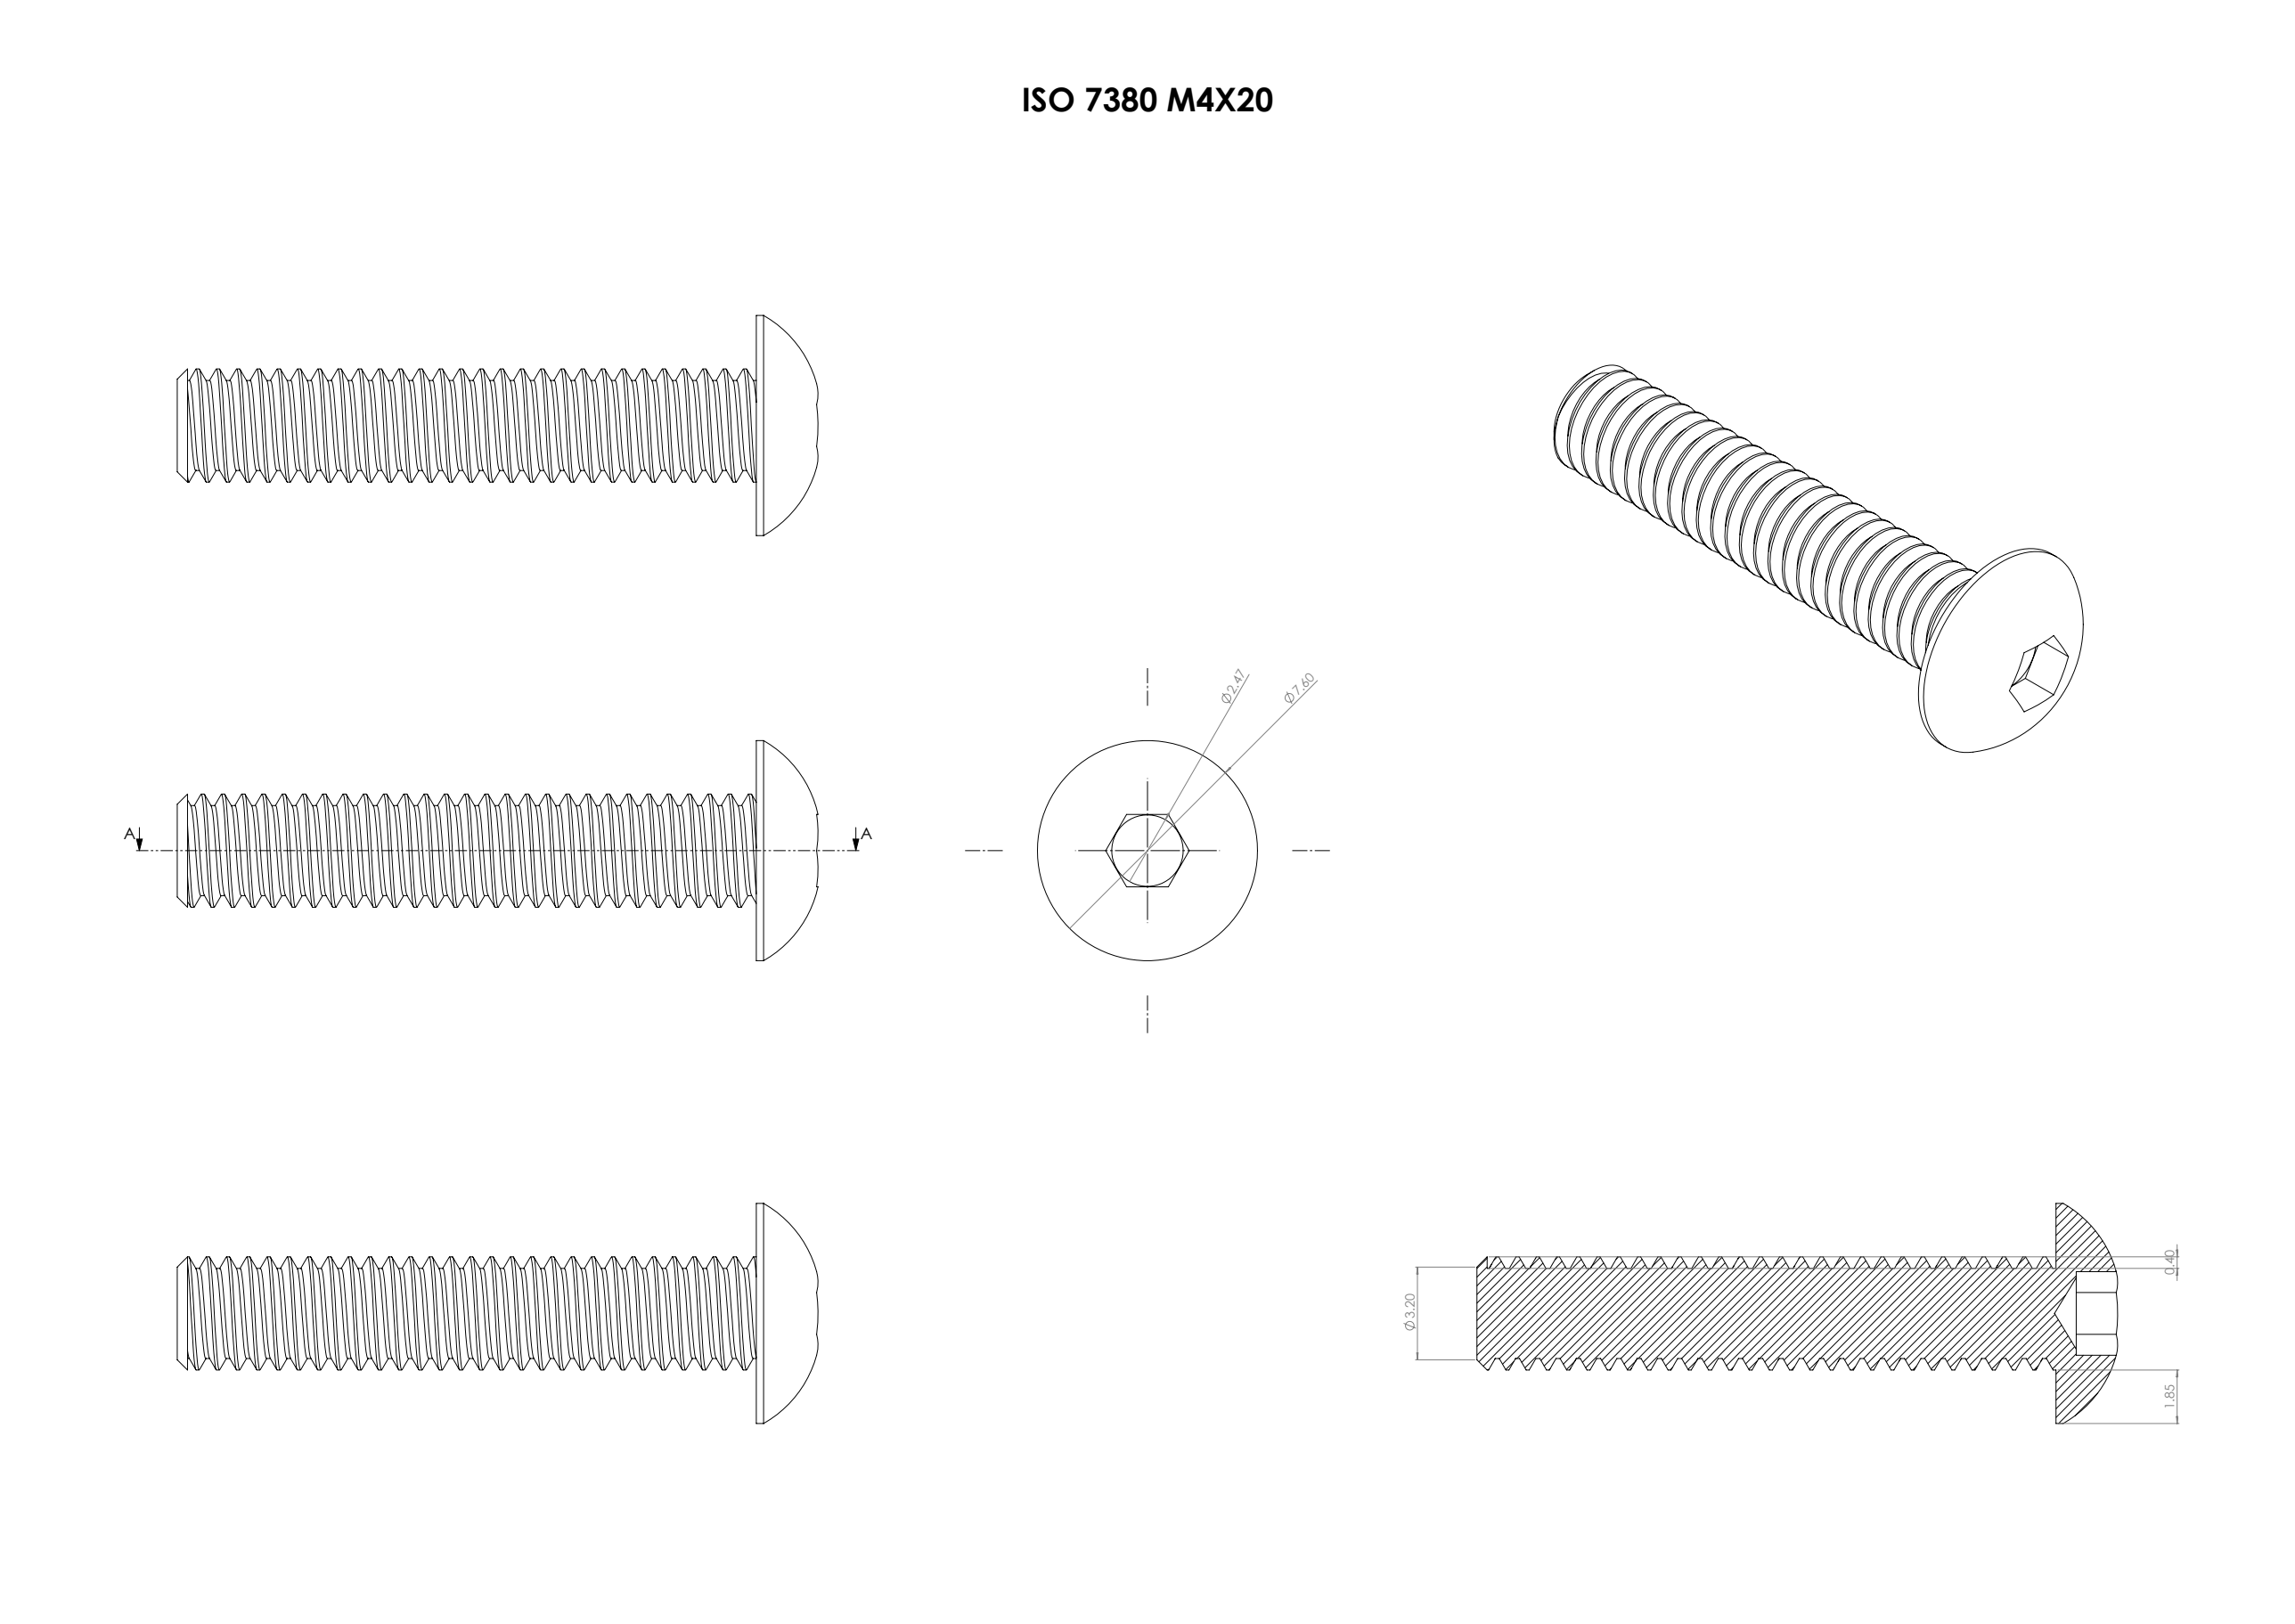
ISO-10303-21;
HEADER;
/* Generated by software containing ST-Developer
 * from STEP Tools, Inc. (www.steptools.com) 
 */

FILE_DESCRIPTION(
/* description */ (''),
/* implementation_level */ '2;1');

FILE_NAME(
/* name */ '11_ISO_7380_M4x20.step',
/* time_stamp */ '2026-10-21T02:01:14-07:00',
/* author */ (''),
/* organization */ (''),
/* preprocessor_version */ 'ST-DEVELOPER v20.2',
/* originating_system */ 'Autodesk Translation Framework v15.15.0.0',
/* authorisation */ '');

FILE_SCHEMA (('AUTOMOTIVE_DESIGN { 1 0 10303 214 3 1 1 }'));
ENDSEC;

DATA;
#10=MECHANICAL_DESIGN_GEOMETRIC_PRESENTATION_REPRESENTATION('',(#623),#37181);
#103=(
BOUNDED_SURFACE()
B_SPLINE_SURFACE(2,2,((#34249,#34250,#34251,#34252,#34253,#34254,#34255,
#34256,#34257),(#34258,#34259,#34260,#34261,#34262,#34263,#34264,#34265,
#34266),(#34267,#34268,#34269,#34270,#34271,#34272,#34273,#34274,#34275)),
 .UNSPECIFIED.,.F.,.T.,.F.)
B_SPLINE_SURFACE_WITH_KNOTS((3,3),(3,2,2,2,3),(0.516279708895519,1.35421937474488),
(-3.14159265358979,-1.5707963267949,0.,1.5707963267949,3.14159265358979),
 .UNSPECIFIED.)
GEOMETRIC_REPRESENTATION_ITEM()
RATIONAL_B_SPLINE_SURFACE(((1.,0.707106781186548,1.,0.707106781186548,1.,
0.707106781186548,1.,0.707106781186548,1.),(0.91350851712624,0.645948067131631,
0.91350851712624,0.645948067131631,0.91350851712624,0.645948067131631,0.91350851712624,
0.645948067131631,0.91350851712624),(1.,0.707106781186548,1.,0.707106781186548,
1.,0.707106781186548,1.,0.707106781186548,1.)))
REPRESENTATION_ITEM('')
SURFACE()
);
#116=B_SPLINE_SURFACE_WITH_KNOTS('',3,3,((#32297,#32298,#32299,#32300,#32301,
#32302,#32303,#32304,#32305,#32306,#32307,#32308,#32309,#32310,#32311,#32312,
#32313,#32314,#32315,#32316,#32317,#32318,#32319,#32320,#32321,#32322,#32323,
#32324,#32325,#32326,#32327,#32328,#32329,#32330,#32331,#32332,#32333,#32334,
#32335,#32336,#32337,#32338,#32339,#32340,#32341,#32342,#32343,#32344,#32345,
#32346,#32347,#32348,#32349,#32350,#32351,#32352,#32353,#32354,#32355,#32356,
#32357,#32358,#32359,#32360,#32361,#32362,#32363,#32364,#32365,#32366,#32367,
#32368,#32369,#32370,#32371,#32372,#32373,#32374,#32375,#32376,#32377,#32378,
#32379,#32380,#32381,#32382,#32383,#32384,#32385,#32386,#32387,#32388,#32389,
#32390,#32391,#32392,#32393,#32394,#32395,#32396,#32397,#32398,#32399,#32400,
#32401,#32402,#32403,#32404,#32405,#32406,#32407,#32408,#32409,#32410,#32411,
#32412,#32413,#32414,#32415,#32416,#32417,#32418,#32419,#32420,#32421,#32422,
#32423,#32424,#32425,#32426,#32427,#32428,#32429,#32430,#32431,#32432,#32433,
#32434,#32435,#32436,#32437,#32438,#32439,#32440,#32441,#32442,#32443,#32444,
#32445,#32446,#32447,#32448,#32449,#32450,#32451,#32452,#32453,#32454,#32455,
#32456,#32457,#32458,#32459,#32460,#32461,#32462,#32463,#32464,#32465,#32466,
#32467,#32468,#32469,#32470,#32471,#32472,#32473,#32474,#32475,#32476,#32477,
#32478),(#32479,#32480,#32481,#32482,#32483,#32484,#32485,#32486,#32487,
#32488,#32489,#32490,#32491,#32492,#32493,#32494,#32495,#32496,#32497,#32498,
#32499,#32500,#32501,#32502,#32503,#32504,#32505,#32506,#32507,#32508,#32509,
#32510,#32511,#32512,#32513,#32514,#32515,#32516,#32517,#32518,#32519,#32520,
#32521,#32522,#32523,#32524,#32525,#32526,#32527,#32528,#32529,#32530,#32531,
#32532,#32533,#32534,#32535,#32536,#32537,#32538,#32539,#32540,#32541,#32542,
#32543,#32544,#32545,#32546,#32547,#32548,#32549,#32550,#32551,#32552,#32553,
#32554,#32555,#32556,#32557,#32558,#32559,#32560,#32561,#32562,#32563,#32564,
#32565,#32566,#32567,#32568,#32569,#32570,#32571,#32572,#32573,#32574,#32575,
#32576,#32577,#32578,#32579,#32580,#32581,#32582,#32583,#32584,#32585,#32586,
#32587,#32588,#32589,#32590,#32591,#32592,#32593,#32594,#32595,#32596,#32597,
#32598,#32599,#32600,#32601,#32602,#32603,#32604,#32605,#32606,#32607,#32608,
#32609,#32610,#32611,#32612,#32613,#32614,#32615,#32616,#32617,#32618,#32619,
#32620,#32621,#32622,#32623,#32624,#32625,#32626,#32627,#32628,#32629,#32630,
#32631,#32632,#32633,#32634,#32635,#32636,#32637,#32638,#32639,#32640,#32641,
#32642,#32643,#32644,#32645,#32646,#32647,#32648,#32649,#32650,#32651,#32652,
#32653,#32654,#32655,#32656,#32657,#32658,#32659,#32660),(#32661,#32662,
#32663,#32664,#32665,#32666,#32667,#32668,#32669,#32670,#32671,#32672,#32673,
#32674,#32675,#32676,#32677,#32678,#32679,#32680,#32681,#32682,#32683,#32684,
#32685,#32686,#32687,#32688,#32689,#32690,#32691,#32692,#32693,#32694,#32695,
#32696,#32697,#32698,#32699,#32700,#32701,#32702,#32703,#32704,#32705,#32706,
#32707,#32708,#32709,#32710,#32711,#32712,#32713,#32714,#32715,#32716,#32717,
#32718,#32719,#32720,#32721,#32722,#32723,#32724,#32725,#32726,#32727,#32728,
#32729,#32730,#32731,#32732,#32733,#32734,#32735,#32736,#32737,#32738,#32739,
#32740,#32741,#32742,#32743,#32744,#32745,#32746,#32747,#32748,#32749,#32750,
#32751,#32752,#32753,#32754,#32755,#32756,#32757,#32758,#32759,#32760,#32761,
#32762,#32763,#32764,#32765,#32766,#32767,#32768,#32769,#32770,#32771,#32772,
#32773,#32774,#32775,#32776,#32777,#32778,#32779,#32780,#32781,#32782,#32783,
#32784,#32785,#32786,#32787,#32788,#32789,#32790,#32791,#32792,#32793,#32794,
#32795,#32796,#32797,#32798,#32799,#32800,#32801,#32802,#32803,#32804,#32805,
#32806,#32807,#32808,#32809,#32810,#32811,#32812,#32813,#32814,#32815,#32816,
#32817,#32818,#32819,#32820,#32821,#32822,#32823,#32824,#32825,#32826,#32827,
#32828,#32829,#32830,#32831,#32832,#32833,#32834,#32835,#32836,#32837,#32838,
#32839,#32840,#32841,#32842),(#32843,#32844,#32845,#32846,#32847,#32848,
#32849,#32850,#32851,#32852,#32853,#32854,#32855,#32856,#32857,#32858,#32859,
#32860,#32861,#32862,#32863,#32864,#32865,#32866,#32867,#32868,#32869,#32870,
#32871,#32872,#32873,#32874,#32875,#32876,#32877,#32878,#32879,#32880,#32881,
#32882,#32883,#32884,#32885,#32886,#32887,#32888,#32889,#32890,#32891,#32892,
#32893,#32894,#32895,#32896,#32897,#32898,#32899,#32900,#32901,#32902,#32903,
#32904,#32905,#32906,#32907,#32908,#32909,#32910,#32911,#32912,#32913,#32914,
#32915,#32916,#32917,#32918,#32919,#32920,#32921,#32922,#32923,#32924,#32925,
#32926,#32927,#32928,#32929,#32930,#32931,#32932,#32933,#32934,#32935,#32936,
#32937,#32938,#32939,#32940,#32941,#32942,#32943,#32944,#32945,#32946,#32947,
#32948,#32949,#32950,#32951,#32952,#32953,#32954,#32955,#32956,#32957,#32958,
#32959,#32960,#32961,#32962,#32963,#32964,#32965,#32966,#32967,#32968,#32969,
#32970,#32971,#32972,#32973,#32974,#32975,#32976,#32977,#32978,#32979,#32980,
#32981,#32982,#32983,#32984,#32985,#32986,#32987,#32988,#32989,#32990,#32991,
#32992,#32993,#32994,#32995,#32996,#32997,#32998,#32999,#33000,#33001,#33002,
#33003,#33004,#33005,#33006,#33007,#33008,#33009,#33010,#33011,#33012,#33013,
#33014,#33015,#33016,#33017,#33018,#33019,#33020,#33021,#33022,#33023,#33024)),
 .UNSPECIFIED.,.F.,.F.,.F.,(4,4),(4,1,1,1,1,1,1,1,1,1,1,1,1,1,1,1,1,1,1,
1,1,1,1,1,1,1,1,1,1,1,1,1,1,1,1,1,1,1,1,1,1,1,1,1,1,1,1,1,1,1,1,1,1,1,1,
1,1,1,1,1,1,1,1,1,1,1,1,1,1,1,1,1,1,1,1,1,1,1,1,1,1,1,1,1,1,1,1,1,1,1,1,
1,1,1,1,1,1,1,1,1,1,1,1,1,1,1,1,1,1,1,1,1,1,1,1,1,1,1,1,1,1,1,1,1,1,1,1,
1,1,1,1,1,1,1,1,1,1,1,1,1,1,1,1,1,1,1,1,1,1,1,1,1,1,1,1,1,1,1,1,1,1,1,1,
1,1,1,1,1,1,1,1,1,1,1,1,1,1,1,1,4),(0.,0.0460148164544131),(8.3105869227399,
9.3072753236828,10.3039637246257,11.3006521255686,12.2973405265115,13.2940289274544,
14.2907173283973,15.2874057293402,16.2840941302831,17.280782531226,18.2774709321689,
19.2741593331118,20.2708477340547,21.2675361349975,22.2642245359404,23.2609129368833,
24.2576013378262,25.2542897387691,26.250978139712,27.2476665406549,28.2443549415978,
29.2410433425407,30.2377317434836,31.2344201444265,32.2311085453694,33.2277969463123,
34.2244853472552,35.2211737481981,36.217862149141,37.2145505500839,38.2112389510268,
39.2079273519697,40.2046157529126,41.2013041538555,42.1979925547984,43.1946809557413,
44.1913693566841,45.188057757627,46.18474615857,47.1814345595128,48.1781229604557,
49.1748113613986,50.1714997623415,51.1681881632844,52.1648765642273,53.1615649651702,
54.1582533661131,55.154941767056,56.1516301679989,57.1483185689418,58.1450069698847,
59.1416953708276,60.1383837717705,61.1350721727134,62.1317605736563,63.1284489745992,
64.1251373755421,65.121825776485,66.1185141774279,67.1152025783708,68.1118909793137,
69.1085793802565,70.1052677811994,71.1019561821423,72.0986445830852,73.0953329840281,
74.092021384971,75.0887097859139,76.0853981868568,77.0820865877997,78.0787749887426,
79.0754633896855,80.0721517906284,81.0688401915713,82.0655285925142,83.0622169934571,
84.0589053944,85.0555937953429,86.0522821962858,87.0489705972287,88.0456589981716,
89.0423473991145,90.0390358000574,91.0357242010002,92.0324126019432,93.029101002886,
94.0257894038289,95.0224778047718,96.0191662057147,97.0158546066576,98.0125430076005,
99.0092314085434,100.005919809486,101.002608210429,101.999296611372,102.995985012315,
103.992673413258,104.989361814201,105.986050215144,106.982738616087,107.979427017029,
108.976115417972,109.972803818915,110.969492219858,111.966180620801,112.962869021744,
113.959557422687,114.95624582363,115.952934224573,116.949622625516,117.946311026458,
118.942999427401,119.939687828344,120.936376229287,121.93306463023,122.929753031173,
123.926441432116,124.923129833059,125.919818234002,126.916506634944,127.913195035887,
128.90988343683,129.906571837773,130.903260238716,131.899948639659,132.896637040602,
133.893325441545,134.890013842488,135.886702243431,136.883390644373,137.880079045316,
138.876767446259,139.873455847202,140.870144248145,141.866832649088,142.863521050031,
143.860209450974,144.856897851917,145.85358625286,146.850274653802,147.846963054745,
148.843651455688,149.840339856631,150.837028257574,151.833716658517,152.83040505946,
153.827093460403,154.823781861346,155.820470262288,156.817158663231,157.813847064174,
158.810535465117,159.80722386606,160.803912267003,161.800600667946,162.797289068889,
163.793977469832,164.790665870775,165.787354271717,166.78404267266,167.780731073603,
168.777419474546,169.774107875489,170.770796276432,171.767484677375,172.764173078318,
173.760861479261,174.757549880203,175.754238281146,176.750926682089,177.747615083032,
178.744303483975,179.740991884918,180.737680285861,181.734368686804,182.731057087747,
183.72774548869,184.724433889632,185.721122290575,186.717810691518),
 .UNSPECIFIED.);
#117=B_SPLINE_SURFACE_WITH_KNOTS('',3,3,((#33328,#33329,#33330,#33331,#33332,
#33333,#33334,#33335,#33336,#33337,#33338,#33339,#33340,#33341,#33342,#33343,
#33344,#33345,#33346,#33347,#33348,#33349,#33350,#33351,#33352,#33353,#33354,
#33355,#33356,#33357,#33358,#33359,#33360,#33361,#33362,#33363,#33364,#33365,
#33366,#33367,#33368,#33369,#33370,#33371,#33372,#33373,#33374,#33375,#33376,
#33377,#33378,#33379,#33380,#33381,#33382,#33383,#33384,#33385,#33386,#33387,
#33388,#33389,#33390,#33391,#33392,#33393,#33394,#33395,#33396,#33397,#33398,
#33399,#33400,#33401,#33402,#33403,#33404,#33405,#33406,#33407,#33408,#33409,
#33410,#33411,#33412,#33413,#33414,#33415,#33416,#33417,#33418,#33419,#33420,
#33421,#33422,#33423,#33424,#33425,#33426,#33427,#33428,#33429,#33430,#33431,
#33432,#33433,#33434,#33435,#33436,#33437,#33438,#33439,#33440,#33441,#33442,
#33443,#33444,#33445,#33446,#33447,#33448,#33449,#33450,#33451,#33452,#33453,
#33454,#33455,#33456,#33457,#33458,#33459,#33460,#33461,#33462,#33463,#33464,
#33465,#33466,#33467,#33468,#33469,#33470,#33471,#33472,#33473,#33474,#33475,
#33476,#33477,#33478,#33479,#33480,#33481,#33482,#33483,#33484,#33485,#33486,
#33487,#33488,#33489,#33490,#33491,#33492,#33493,#33494,#33495,#33496,#33497,
#33498,#33499,#33500,#33501,#33502,#33503,#33504,#33505,#33506,#33507,#33508,
#33509),(#33510,#33511,#33512,#33513,#33514,#33515,#33516,#33517,#33518,
#33519,#33520,#33521,#33522,#33523,#33524,#33525,#33526,#33527,#33528,#33529,
#33530,#33531,#33532,#33533,#33534,#33535,#33536,#33537,#33538,#33539,#33540,
#33541,#33542,#33543,#33544,#33545,#33546,#33547,#33548,#33549,#33550,#33551,
#33552,#33553,#33554,#33555,#33556,#33557,#33558,#33559,#33560,#33561,#33562,
#33563,#33564,#33565,#33566,#33567,#33568,#33569,#33570,#33571,#33572,#33573,
#33574,#33575,#33576,#33577,#33578,#33579,#33580,#33581,#33582,#33583,#33584,
#33585,#33586,#33587,#33588,#33589,#33590,#33591,#33592,#33593,#33594,#33595,
#33596,#33597,#33598,#33599,#33600,#33601,#33602,#33603,#33604,#33605,#33606,
#33607,#33608,#33609,#33610,#33611,#33612,#33613,#33614,#33615,#33616,#33617,
#33618,#33619,#33620,#33621,#33622,#33623,#33624,#33625,#33626,#33627,#33628,
#33629,#33630,#33631,#33632,#33633,#33634,#33635,#33636,#33637,#33638,#33639,
#33640,#33641,#33642,#33643,#33644,#33645,#33646,#33647,#33648,#33649,#33650,
#33651,#33652,#33653,#33654,#33655,#33656,#33657,#33658,#33659,#33660,#33661,
#33662,#33663,#33664,#33665,#33666,#33667,#33668,#33669,#33670,#33671,#33672,
#33673,#33674,#33675,#33676,#33677,#33678,#33679,#33680,#33681,#33682,#33683,
#33684,#33685,#33686,#33687,#33688,#33689,#33690,#33691),(#33692,#33693,
#33694,#33695,#33696,#33697,#33698,#33699,#33700,#33701,#33702,#33703,#33704,
#33705,#33706,#33707,#33708,#33709,#33710,#33711,#33712,#33713,#33714,#33715,
#33716,#33717,#33718,#33719,#33720,#33721,#33722,#33723,#33724,#33725,#33726,
#33727,#33728,#33729,#33730,#33731,#33732,#33733,#33734,#33735,#33736,#33737,
#33738,#33739,#33740,#33741,#33742,#33743,#33744,#33745,#33746,#33747,#33748,
#33749,#33750,#33751,#33752,#33753,#33754,#33755,#33756,#33757,#33758,#33759,
#33760,#33761,#33762,#33763,#33764,#33765,#33766,#33767,#33768,#33769,#33770,
#33771,#33772,#33773,#33774,#33775,#33776,#33777,#33778,#33779,#33780,#33781,
#33782,#33783,#33784,#33785,#33786,#33787,#33788,#33789,#33790,#33791,#33792,
#33793,#33794,#33795,#33796,#33797,#33798,#33799,#33800,#33801,#33802,#33803,
#33804,#33805,#33806,#33807,#33808,#33809,#33810,#33811,#33812,#33813,#33814,
#33815,#33816,#33817,#33818,#33819,#33820,#33821,#33822,#33823,#33824,#33825,
#33826,#33827,#33828,#33829,#33830,#33831,#33832,#33833,#33834,#33835,#33836,
#33837,#33838,#33839,#33840,#33841,#33842,#33843,#33844,#33845,#33846,#33847,
#33848,#33849,#33850,#33851,#33852,#33853,#33854,#33855,#33856,#33857,#33858,
#33859,#33860,#33861,#33862,#33863,#33864,#33865,#33866,#33867,#33868,#33869,
#33870,#33871,#33872,#33873),(#33874,#33875,#33876,#33877,#33878,#33879,
#33880,#33881,#33882,#33883,#33884,#33885,#33886,#33887,#33888,#33889,#33890,
#33891,#33892,#33893,#33894,#33895,#33896,#33897,#33898,#33899,#33900,#33901,
#33902,#33903,#33904,#33905,#33906,#33907,#33908,#33909,#33910,#33911,#33912,
#33913,#33914,#33915,#33916,#33917,#33918,#33919,#33920,#33921,#33922,#33923,
#33924,#33925,#33926,#33927,#33928,#33929,#33930,#33931,#33932,#33933,#33934,
#33935,#33936,#33937,#33938,#33939,#33940,#33941,#33942,#33943,#33944,#33945,
#33946,#33947,#33948,#33949,#33950,#33951,#33952,#33953,#33954,#33955,#33956,
#33957,#33958,#33959,#33960,#33961,#33962,#33963,#33964,#33965,#33966,#33967,
#33968,#33969,#33970,#33971,#33972,#33973,#33974,#33975,#33976,#33977,#33978,
#33979,#33980,#33981,#33982,#33983,#33984,#33985,#33986,#33987,#33988,#33989,
#33990,#33991,#33992,#33993,#33994,#33995,#33996,#33997,#33998,#33999,#34000,
#34001,#34002,#34003,#34004,#34005,#34006,#34007,#34008,#34009,#34010,#34011,
#34012,#34013,#34014,#34015,#34016,#34017,#34018,#34019,#34020,#34021,#34022,
#34023,#34024,#34025,#34026,#34027,#34028,#34029,#34030,#34031,#34032,#34033,
#34034,#34035,#34036,#34037,#34038,#34039,#34040,#34041,#34042,#34043,#34044,
#34045,#34046,#34047,#34048,#34049,#34050,#34051,#34052,#34053,#34054,#34055)),
 .UNSPECIFIED.,.F.,.F.,.F.,(4,4),(4,1,1,1,1,1,1,1,1,1,1,1,1,1,1,1,1,1,1,
1,1,1,1,1,1,1,1,1,1,1,1,1,1,1,1,1,1,1,1,1,1,1,1,1,1,1,1,1,1,1,1,1,1,1,1,
1,1,1,1,1,1,1,1,1,1,1,1,1,1,1,1,1,1,1,1,1,1,1,1,1,1,1,1,1,1,1,1,1,1,1,1,
1,1,1,1,1,1,1,1,1,1,1,1,1,1,1,1,1,1,1,1,1,1,1,1,1,1,1,1,1,1,1,1,1,1,1,1,
1,1,1,1,1,1,1,1,1,1,1,1,1,1,1,1,1,1,1,1,1,1,1,1,1,1,1,1,1,1,1,1,1,1,1,1,
1,1,1,1,1,1,1,1,1,1,1,1,1,1,1,1,4),(0.,0.0460148164544131),(11.6154215191108,
12.6121099200537,13.6087983209966,14.6054867219395,15.6021751228824,16.5988635238253,
17.5955519247682,18.592240325711,19.5889287266539,20.5856171275968,21.5823055285397,
22.5789939294826,23.5756823304255,24.5723707313684,25.5690591323113,26.5657475332542,
27.5624359341971,28.55912433514,29.5558127360829,30.5525011370258,31.5491895379687,
32.5458779389116,33.5425663398545,34.5392547407974,35.5359431417403,36.5326315426832,
37.5293199436261,38.526008344569,39.5226967455119,40.5193851464548,41.5160735473976,
42.5127619483405,43.5094503492834,44.5061387502263,45.5028271511692,46.4995155521121,
47.496203953055,48.4928923539979,49.4895807549408,50.4862691558837,51.4829575568266,
52.4796459577695,53.4763343587124,54.4730227596553,55.4697111605982,56.4663995615411,
57.463087962484,58.4597763634269,59.4564647643698,60.4531531653127,61.4498415662556,
62.4465299671985,63.4432183681413,64.4399067690842,65.4365951700271,66.43328357097,
67.4299719719129,68.4266603728558,69.4233487737987,70.4200371747416,71.4167255756845,
72.4134139766274,73.4101023775703,74.4067907785132,75.4034791794561,76.400167580399,
77.3968559813419,78.3935443822848,79.3902327832277,80.3869211841706,81.3836095851135,
82.3802979860564,83.3769863869992,84.3736747879422,85.3703631888851,86.3670515898279,
87.3637399907708,88.3604283917137,89.3571167926566,90.3538051935995,91.3504935945424,
92.3471819954853,93.3438703964282,94.3405587973711,95.337247198314,96.3339355992569,
97.3306240001998,98.3273124011427,99.3240008020856,100.320689203028,101.317377603971,
102.314066004914,103.310754405857,104.3074428068,105.304131207743,106.300819608686,
107.297508009629,108.294196410572,109.290884811515,110.287573212457,111.2842616134,
112.280950014343,113.277638415286,114.274326816229,115.271015217172,116.267703618115,
117.264392019058,118.261080420001,119.257768820943,120.254457221886,121.251145622829,
122.247834023772,123.244522424715,124.241210825658,125.237899226601,126.234587627544,
127.231276028487,128.22796442943,129.224652830372,130.221341231315,131.218029632258,
132.214718033201,133.211406434144,134.208094835087,135.20478323603,136.201471636973,
137.198160037916,138.194848438859,139.191536839801,140.188225240744,141.184913641687,
142.18160204263,143.178290443573,144.174978844516,145.171667245459,146.168355646402,
147.165044047345,148.161732448287,149.15842084923,150.155109250173,151.151797651116,
152.148486052059,153.145174453002,154.141862853945,155.138551254888,156.135239655831,
157.131928056774,158.128616457716,159.125304858659,160.121993259602,161.118681660545,
162.115370061488,163.112058462431,164.108746863374,165.105435264317,166.10212366526,
167.098812066202,168.095500467145,169.092188868088,170.088877269031,171.085565669974,
172.082254070917,173.07894247186,174.075630872803,175.072319273746,176.069007674689,
177.065696075631,178.062384476574,179.059072877517,180.05576127846,181.052449679403,
182.049138080346,183.045826481289,184.042514882232,185.039203283175,186.035891684118,
187.03258008506,188.029268486003,189.025956886946,190.022645287889),
 .UNSPECIFIED.);
#379=B_SPLINE_CURVE_WITH_KNOTS('',3,(#30252,#30253,#30254,#30255,#30256,
#30257,#30258,#30259,#30260,#30261),.UNSPECIFIED.,.F.,.F.,(4,3,3,4),(-4.09254174883827,
-3.98675360377158,-2.99006520282869,-2.06514013327809),.UNSPECIFIED.);
#380=B_SPLINE_CURVE_WITH_KNOTS('',3,(#30264,#30265,#30266,#30267,#30268,
#30269,#30270),.UNSPECIFIED.,.F.,.F.,(4,3,4),(0.,0.996688400942905,1.11419103802963),
 .UNSPECIFIED.);
#381=B_SPLINE_CURVE_WITH_KNOTS('',3,(#30275,#30276,#30277,#30278,#30279,
#30280,#30281,#30282,#30283,#30284,#30285,#30286,#30287,#30288,#30289,#30290,
#30291,#30292,#30293,#30294,#30295,#30296),.UNSPECIFIED.,.F.,.F.,(4,3,3,
3,3,3,3,4),(-10.3757270560179,-9.96688400942895,-8.97019560848606,-7.97350720754317,
-6.97681880660027,-5.98013040565738,-4.98344200471448,-4.09254174883827),
 .UNSPECIFIED.);
#382=B_SPLINE_CURVE_WITH_KNOTS('',3,(#30297,#30298,#30299,#30300,#30301,
#30302,#30303,#30304,#30305,#30306,#30307,#30308,#30309,#30310,#30311,#30312,
#30313,#30314,#30315,#30316,#30317,#30318),.UNSPECIFIED.,.F.,.F.,(4,3,3,
3,3,3,3,4),(1.11419103802963,1.9933768018858,2.99006520282869,3.98675360377159,
4.98344200471448,5.98013040565737,6.97681880660027,7.39737634520922),
 .UNSPECIFIED.);
#383=B_SPLINE_CURVE_WITH_KNOTS('',3,(#30323,#30324,#30325,#30326,#30327,
#30328,#30329,#30330,#30331,#30332,#30333,#30334,#30335,#30336,#30337,#30338,
#30339,#30340,#30341,#30342,#30343,#30344),.UNSPECIFIED.,.F.,.F.,(4,3,3,
3,3,3,3,4),(-16.6589123631975,-15.9470144150863,-14.9503260141434,-13.9536376132005,
-12.9569492122576,-11.9602608113147,-10.9635724103719,-10.3757270560179),
 .UNSPECIFIED.);
#384=B_SPLINE_CURVE_WITH_KNOTS('',3,(#30345,#30346,#30347,#30348,#30349,
#30350,#30351,#30352,#30353,#30354,#30355,#30356,#30357,#30358,#30359,#30360,
#30361,#30362,#30363,#30364,#30365,#30366),.UNSPECIFIED.,.F.,.F.,(4,3,3,
3,3,3,3,4),(7.39737634520922,7.97350720754316,8.97019560848606,9.96688400942896,
10.9635724103719,11.9602608113148,12.9569492122576,13.6805616523888),
 .UNSPECIFIED.);
#385=B_SPLINE_CURVE_WITH_KNOTS('',3,(#30371,#30372,#30373,#30374,#30375,
#30376,#30377,#30378,#30379,#30380,#30381,#30382,#30383,#30384,#30385,#30386,
#30387,#30388,#30389,#30390,#30391,#30392,#30393,#30394,#30395),
 .UNSPECIFIED.,.F.,.F.,(4,3,3,3,3,3,3,3,4),(-22.942097670377,-22.9238332216866,
-21.9271448207437,-20.9304564198008,-19.9337680188579,-18.937079617915,
-17.9403912169721,-16.9437028160292,-16.6589123631975),.UNSPECIFIED.);
#386=B_SPLINE_CURVE_WITH_KNOTS('',3,(#30396,#30397,#30398,#30399,#30400,
#30401,#30402,#30403,#30404,#30405,#30406,#30407,#30408,#30409,#30410,#30411,
#30412,#30413,#30414,#30415,#30416,#30417,#30418,#30419,#30420),
 .UNSPECIFIED.,.F.,.F.,(4,3,3,3,3,3,3,3,4),(13.6805616523888,13.9536376132005,
14.9503260141434,15.9470144150863,16.9437028160292,17.9403912169721,18.937079617915,
19.9337680188579,19.9637469595684),.UNSPECIFIED.);
#387=B_SPLINE_CURVE_WITH_KNOTS('',3,(#30425,#30426,#30427,#30428,#30429,
#30430,#30431,#30432,#30433,#30434,#30435,#30436,#30437,#30438,#30439,#30440,
#30441,#30442,#30443,#30444,#30445,#30446),.UNSPECIFIED.,.F.,.F.,(4,3,3,
3,3,3,3,4),(-29.2252829775566,-28.903963627344,-27.9072752264011,-26.9105868254582,
-25.9138984245153,-24.9172100235724,-23.9205216226295,-22.942097670377),
 .UNSPECIFIED.);
#388=B_SPLINE_CURVE_WITH_KNOTS('',3,(#30447,#30448,#30449,#30450,#30451,
#30452,#30453,#30454,#30455,#30456,#30457,#30458,#30459,#30460,#30461,#30462,
#30463,#30464,#30465,#30466,#30467,#30468),.UNSPECIFIED.,.F.,.F.,(4,3,3,
3,3,3,3,4),(19.9637469595684,20.9304564198008,21.9271448207437,22.9238332216866,
23.9205216226295,24.9172100235724,25.9138984245153,26.246932266748),
 .UNSPECIFIED.);
#389=B_SPLINE_CURVE_WITH_KNOTS('',3,(#30473,#30474,#30475,#30476,#30477,
#30478,#30479,#30480,#30481,#30482,#30483,#30484,#30485,#30486,#30487,#30488,
#30489,#30490,#30491,#30492,#30493,#30494),.UNSPECIFIED.,.F.,.F.,(4,3,3,
3,3,3,3,4),(-35.5084682847362,-34.8840940330013,-33.8874056320584,-32.8907172311156,
-31.8940288301727,-30.8973404292298,-29.9006520282869,-29.2252829775566),
 .UNSPECIFIED.);
#390=B_SPLINE_CURVE_WITH_KNOTS('',3,(#30495,#30496,#30497,#30498,#30499,
#30500,#30501,#30502,#30503,#30504,#30505,#30506,#30507,#30508,#30509,#30510,
#30511,#30512,#30513,#30514,#30515,#30516),.UNSPECIFIED.,.F.,.F.,(4,3,3,
3,3,3,3,4),(26.246932266748,26.9105868254582,27.9072752264011,28.903963627344,
29.9006520282869,30.8973404292298,31.8940288301727,32.5301175739276),
 .UNSPECIFIED.);
#391=B_SPLINE_CURVE_WITH_KNOTS('',3,(#30521,#30522,#30523,#30524,#30525,
#30526,#30527,#30528,#30529,#30530,#30531,#30532,#30533,#30534,#30535,#30536,
#30537,#30538,#30539,#30540,#30541,#30542),.UNSPECIFIED.,.F.,.F.,(4,3,3,
3,3,3,3,4),(-41.7916535919158,-40.8642244386587,-39.8675360377158,-38.8708476367729,
-37.87415923583,-36.8774708348871,-35.8807824339442,-35.5084682847362),
 .UNSPECIFIED.);
#392=B_SPLINE_CURVE_WITH_KNOTS('',3,(#30543,#30544,#30545,#30546,#30547,
#30548,#30549,#30550,#30551,#30552,#30553,#30554,#30555,#30556,#30557,#30558,
#30559,#30560,#30561,#30562,#30563,#30564),.UNSPECIFIED.,.F.,.F.,(4,3,3,
3,3,3,3,4),(32.5301175739276,32.8907172311156,33.8874056320585,34.8840940330014,
35.8807824339443,36.8774708348872,37.8741592358301,38.8133028811072),
 .UNSPECIFIED.);
#393=B_SPLINE_CURVE_WITH_KNOTS('',3,(#30569,#30570,#30571,#30572,#30573,
#30574,#30575,#30576,#30577,#30578,#30579,#30580,#30581,#30582,#30583,#30584,
#30585,#30586,#30587,#30588,#30589,#30590,#30591,#30592,#30593),
 .UNSPECIFIED.,.F.,.F.,(4,3,3,3,3,3,3,3,4),(-48.0748388990954,-47.841043245259,
-46.8443548443161,-45.8476664433732,-44.8509780424303,-43.8542896414874,
-42.8576012405445,-41.8609128396016,-41.7916535919158),.UNSPECIFIED.);
#394=B_SPLINE_CURVE_WITH_KNOTS('',3,(#30594,#30595,#30596,#30597,#30598,
#30599,#30600,#30601,#30602,#30603,#30604,#30605,#30606,#30607,#30608,#30609,
#30610,#30611,#30612,#30613,#30614,#30615,#30616,#30617,#30618),
 .UNSPECIFIED.,.F.,.F.,(4,3,3,3,3,3,3,3,4),(38.8133028811072,38.8708476367729,
39.8675360377158,40.8642244386587,41.8609128396016,42.8576012405445,43.8542896414874,
44.8509780424303,45.0964881882868),.UNSPECIFIED.);
#395=B_SPLINE_CURVE_WITH_KNOTS('',3,(#30623,#30624,#30625,#30626,#30627,
#30628,#30629,#30630,#30631,#30632,#30633,#30634,#30635,#30636,#30637,#30638,
#30639,#30640,#30641,#30642,#30643,#30644),.UNSPECIFIED.,.F.,.F.,(4,3,3,
3,3,3,3,4),(-54.358024206275,-53.8211736509164,-52.8244852499735,-51.8277968490306,
-50.8311084480877,-49.8344200471448,-48.8377316462019,-48.0748388990954),
 .UNSPECIFIED.);
#396=B_SPLINE_CURVE_WITH_KNOTS('',3,(#30645,#30646,#30647,#30648,#30649,
#30650,#30651,#30652,#30653,#30654,#30655,#30656,#30657,#30658,#30659,#30660,
#30661,#30662,#30663,#30664,#30665,#30666),.UNSPECIFIED.,.F.,.F.,(4,3,3,
3,3,3,3,4),(45.0964881882868,45.8476664433732,46.8443548443161,47.841043245259,
48.8377316462019,49.8344200471448,50.8311084480877,51.3796734954663),
 .UNSPECIFIED.);
#397=B_SPLINE_CURVE_WITH_KNOTS('',3,(#30671,#30672,#30673,#30674,#30675,
#30676,#30677,#30678,#30679,#30680,#30681,#30682,#30683,#30684,#30685,#30686,
#30687,#30688,#30689,#30690,#30691,#30692),.UNSPECIFIED.,.F.,.F.,(4,3,3,
3,3,3,3,4),(-60.6412095134546,-59.8013040565737,-58.8046156556308,-57.8079272546879,
-56.811238853745,-55.8145504528021,-54.8178620518593,-54.358024206275),
 .UNSPECIFIED.);
#398=B_SPLINE_CURVE_WITH_KNOTS('',3,(#30693,#30694,#30695,#30696,#30697,
#30698,#30699,#30700,#30701,#30702,#30703,#30704,#30705,#30706,#30707,#30708,
#30709,#30710,#30711,#30712,#30713,#30714),.UNSPECIFIED.,.F.,.F.,(4,3,3,
3,3,3,3,4),(51.3796734954663,51.8277968490306,52.8244852499735,53.8211736509164,
54.8178620518593,55.8145504528022,56.8112388537451,57.6628588026459),
 .UNSPECIFIED.);
#399=B_SPLINE_CURVE_WITH_KNOTS('',3,(#30719,#30720,#30721,#30722,#30723,
#30724,#30725,#30726,#30727,#30728,#30729,#30730,#30731,#30732,#30733,#30734,
#30735,#30736,#30737,#30738,#30739,#30740,#30741,#30742,#30743),
 .UNSPECIFIED.,.F.,.F.,(4,3,3,3,3,3,3,3,4),(-66.9243948206342,-66.778122863174,
-65.7814344622311,-64.7847460612882,-63.7880576603453,-62.7913692594024,
-61.7946808584595,-60.7979924575166,-60.6412095134546),.UNSPECIFIED.);
#400=B_SPLINE_CURVE_WITH_KNOTS('',3,(#30744,#30745,#30746,#30747,#30748,
#30749,#30750,#30751,#30752,#30753,#30754,#30755,#30756,#30757,#30758,#30759,
#30760,#30761,#30762,#30763,#30764,#30765,#30766,#30767,#30768),
 .UNSPECIFIED.,.F.,.F.,(4,3,3,3,3,3,3,3,4),(57.6628588026459,57.8079272546879,
58.8046156556308,59.8013040565737,60.7979924575166,61.7946808584595,62.7913692594024,
63.7880576603453,63.9460441098255),.UNSPECIFIED.);
#401=B_SPLINE_CURVE_WITH_KNOTS('',3,(#30773,#30774,#30775,#30776,#30777,
#30778,#30779,#30780,#30781,#30782,#30783,#30784,#30785,#30786,#30787,#30788,
#30789,#30790,#30791,#30792,#30793,#30794),.UNSPECIFIED.,.F.,.F.,(4,3,3,
3,3,3,3,4),(-73.2075801278138,-72.7582532688314,-71.7615648678885,-70.7648764669456,
-69.7681880660027,-68.7714996650598,-67.7748112641169,-66.9243948206342),
 .UNSPECIFIED.);
#402=B_SPLINE_CURVE_WITH_KNOTS('',3,(#30795,#30796,#30797,#30798,#30799,
#30800,#30801,#30802,#30803,#30804,#30805,#30806,#30807,#30808,#30809,#30810,
#30811,#30812,#30813,#30814,#30815,#30816),.UNSPECIFIED.,.F.,.F.,(4,3,3,
3,3,3,3,4),(63.9460441098255,64.7847460612882,65.7814344622311,66.778122863174,
67.7748112641169,68.7714996650598,69.7681880660027,70.2292294170051),
 .UNSPECIFIED.);
#403=B_SPLINE_CURVE_WITH_KNOTS('',3,(#30821,#30822,#30823,#30824,#30825,
#30826,#30827,#30828,#30829,#30830,#30831,#30832,#30833,#30834,#30835,#30836,
#30837,#30838,#30839,#30840,#30841,#30842),.UNSPECIFIED.,.F.,.F.,(4,3,3,
3,3,3,3,4),(-79.4907654349934,-78.7383836744887,-77.7416952735459,-76.745006872603,
-75.7483184716601,-74.7516300707172,-73.7549416697743,-73.2075801278138),
 .UNSPECIFIED.);
#404=B_SPLINE_CURVE_WITH_KNOTS('',3,(#30843,#30844,#30845,#30846,#30847,
#30848,#30849,#30850,#30851,#30852,#30853,#30854,#30855,#30856,#30857,#30858,
#30859,#30860,#30861,#30862,#30863,#30864),.UNSPECIFIED.,.F.,.F.,(4,3,3,
3,3,3,3,4),(70.2292294170051,70.7648764669456,71.7615648678885,72.7582532688314,
73.7549416697743,74.7516300707172,75.7483184716601,76.5124147241847),
 .UNSPECIFIED.);
#405=B_SPLINE_CURVE_WITH_KNOTS('',3,(#30869,#30870,#30871,#30872,#30873,
#30874,#30875,#30876,#30877,#30878,#30879,#30880,#30881,#30882,#30883,#30884,
#30885,#30886,#30887,#30888,#30889,#30890,#30891,#30892,#30893),
 .UNSPECIFIED.,.F.,.F.,(4,3,3,3,3,3,3,3,4),(-85.773950742173,-85.715202481089,
-84.7185140801461,-83.7218256792032,-82.7251372782603,-81.7284488773174,
-80.7317604763745,-79.7350720754316,-79.4907654349934),.UNSPECIFIED.);
#406=B_SPLINE_CURVE_WITH_KNOTS('',3,(#30894,#30895,#30896,#30897,#30898,
#30899,#30900,#30901,#30902,#30903,#30904,#30905,#30906,#30907,#30908,#30909,
#30910,#30911,#30912,#30913,#30914,#30915,#30916,#30917,#30918),
 .UNSPECIFIED.,.F.,.F.,(4,3,3,3,3,3,3,3,4),(76.5124147241847,76.745006872603,
77.7416952735459,78.7383836744888,79.7350720754317,80.7317604763746,81.7284488773175,
82.7251372782604,82.7956000313643),.UNSPECIFIED.);
#407=B_SPLINE_CURVE_WITH_KNOTS('',3,(#30923,#30924,#30925,#30926,#30927,
#30928,#30929,#30930,#30931,#30932,#30933,#30934,#30935,#30936,#30937,#30938,
#30939,#30940,#30941,#30942,#30943,#30944),.UNSPECIFIED.,.F.,.F.,(4,3,3,
3,3,3,3,4),(-92.0571360493526,-91.6953328867464,-90.6986444858035,-89.7019560848606,
-88.7052676839177,-87.7085792829748,-86.7118908820319,-85.773950742173),
 .UNSPECIFIED.);
#408=B_SPLINE_CURVE_WITH_KNOTS('',3,(#30945,#30946,#30947,#30948,#30949,
#30950,#30951,#30952,#30953,#30954,#30955,#30956,#30957,#30958,#30959,#30960,
#30961,#30962,#30963,#30964,#30965,#30966),.UNSPECIFIED.,.F.,.F.,(4,3,3,
3,3,3,3,4),(82.7956000313643,83.7218256792033,84.7185140801462,85.715202481089,
86.711890882032,87.7085792829748,88.7052676839177,89.0787853385439),
 .UNSPECIFIED.);
#409=B_SPLINE_CURVE_WITH_KNOTS('',3,(#30971,#30972,#30973,#30974,#30975,
#30976,#30977,#30978,#30979,#30980,#30981,#30982,#30983,#30984,#30985,#30986,
#30987,#30988,#30989,#30990,#30991,#30992),.UNSPECIFIED.,.F.,.F.,(4,3,3,
3,3,3,3,4),(-98.3403213565321,-97.6754632924037,-96.6787748914608,-95.682086490518,
-94.6853980895751,-93.6887096886322,-92.6920212876893,-92.0571360493526),
 .UNSPECIFIED.);
#410=B_SPLINE_CURVE_WITH_KNOTS('',3,(#30993,#30994,#30995,#30996,#30997,
#30998,#30999,#31000,#31001,#31002,#31003,#31004,#31005,#31006,#31007,#31008,
#31009,#31010,#31011,#31012,#31013,#31014),.UNSPECIFIED.,.F.,.F.,(4,3,3,
3,3,3,3,4),(89.0787853385439,89.7019560848606,90.6986444858035,91.6953328867464,
92.6920212876893,93.6887096886322,94.6853980895751,95.3619706457235),
 .UNSPECIFIED.);
#411=B_SPLINE_CURVE_WITH_KNOTS('',3,(#31019,#31020,#31021,#31022,#31023,
#31024,#31025,#31026,#31027,#31028,#31029,#31030,#31031,#31032,#31033,#31034,
#31035,#31036,#31037,#31038,#31039,#31040),.UNSPECIFIED.,.F.,.F.,(4,3,3,
3,3,3,3,4),(-104.623506663712,-103.655593698061,-102.658905297118,-101.662216896175,
-100.665528495232,-99.6688400942895,-98.6721516933466,-98.3403213565321),
 .UNSPECIFIED.);
#412=B_SPLINE_CURVE_WITH_KNOTS('',3,(#31041,#31042,#31043,#31044,#31045,
#31046,#31047,#31048,#31049,#31050,#31051,#31052,#31053,#31054,#31055,#31056,
#31057,#31058,#31059,#31060,#31061,#31062),.UNSPECIFIED.,.F.,.F.,(4,3,3,
3,3,3,3,4),(95.3619706457235,95.682086490518,96.6787748914609,97.6754632924038,
98.6721516933467,99.6688400942896,100.665528495232,101.645155952903),
 .UNSPECIFIED.);
#413=B_SPLINE_CURVE_WITH_KNOTS('',3,(#31067,#31068,#31069,#31070,#31071,
#31072,#31073,#31074,#31075,#31076,#31077,#31078,#31079,#31080,#31081,#31082,
#31083,#31084,#31085,#31086,#31087,#31088,#31089,#31090,#31091),
 .UNSPECIFIED.,.F.,.F.,(4,3,3,3,3,3,3,3,4),(-110.906691970891,-110.632412504661,
-109.635724103719,-108.639035702776,-107.642347301833,-106.64565890089,
-105.648970499947,-104.652282099004,-104.623506663712),.UNSPECIFIED.);
#414=B_SPLINE_CURVE_WITH_KNOTS('',3,(#31092,#31093,#31094,#31095,#31096,
#31097,#31098,#31099,#31100,#31101,#31102,#31103,#31104,#31105,#31106,#31107,
#31108,#31109,#31110,#31111,#31112,#31113,#31114,#31115,#31116),
 .UNSPECIFIED.,.F.,.F.,(4,3,3,3,3,3,3,3,4),(101.645155952903,101.662216896175,
102.658905297118,103.655593698061,104.652282099004,105.648970499947,106.64565890089,
107.642347301833,107.928341260083),.UNSPECIFIED.);
#415=B_SPLINE_CURVE_WITH_KNOTS('',3,(#31121,#31122,#31123,#31124,#31125,
#31126,#31127,#31128,#31129,#31130,#31131,#31132,#31133,#31134,#31135,#31136,
#31137,#31138,#31139,#31140,#31141,#31142),.UNSPECIFIED.,.F.,.F.,(4,3,3,
3,3,3,3,4),(-117.189877278071,-116.612542910319,-115.615854509376,-114.619166108433,
-113.62247770749,-112.625789306547,-111.629100905604,-110.906691970891),
 .UNSPECIFIED.);
#416=B_SPLINE_CURVE_WITH_KNOTS('',3,(#31143,#31144,#31145,#31146,#31147,
#31148,#31149,#31150,#31151,#31152,#31153,#31154,#31155,#31156,#31157,#31158,
#31159,#31160,#31161,#31162,#31163,#31164),.UNSPECIFIED.,.F.,.F.,(4,3,3,
3,3,3,3,4),(107.928341260083,108.639035702776,109.635724103719,110.632412504661,
111.629100905604,112.625789306547,113.62247770749,114.211526567262),
 .UNSPECIFIED.);
#417=B_SPLINE_CURVE_WITH_KNOTS('',3,(#31169,#31170,#31171,#31172,#31173,
#31174,#31175,#31176,#31177,#31178,#31179,#31180,#31181,#31182,#31183,#31184,
#31185,#31186,#31187,#31188,#31189,#31190),.UNSPECIFIED.,.F.,.F.,(4,3,3,
3,3,3,3,4),(-123.473062585251,-122.592673315976,-121.595984915033,-120.59929651409,
-119.602608113147,-118.605919712205,-117.609231311262,-117.189877278071),
 .UNSPECIFIED.);
#418=B_SPLINE_CURVE_WITH_KNOTS('',3,(#31191,#31192,#31193,#31194,#31195,
#31196,#31197,#31198,#31199,#31200,#31201,#31202,#31203,#31204,#31205,#31206,
#31207,#31208,#31209,#31210,#31211,#31212),.UNSPECIFIED.,.F.,.F.,(4,3,3,
3,3,3,3,4),(114.211526567262,114.619166108433,115.615854509376,116.612542910319,
117.609231311262,118.605919712205,119.602608113147,120.494711874442),
 .UNSPECIFIED.);
#419=B_SPLINE_CURVE_WITH_KNOTS('',3,(#31217,#31218,#31219,#31220,#31221,
#31222,#31223,#31224,#31225,#31226,#31227,#31228,#31229,#31230,#31231,#31232,
#31233,#31234,#31235,#31236,#31237,#31238,#31239,#31240,#31241),
 .UNSPECIFIED.,.F.,.F.,(4,3,3,3,3,3,3,3,4),(-129.75624789243,-129.569492122576,
-128.572803721634,-127.576115320691,-126.579426919748,-125.582738518805,
-124.586050117862,-123.589361716919,-123.473062585251),.UNSPECIFIED.);
#420=B_SPLINE_CURVE_WITH_KNOTS('',3,(#31242,#31243,#31244,#31245,#31246,
#31247,#31248,#31249,#31250,#31251,#31252,#31253,#31254,#31255,#31256,#31257,
#31258,#31259,#31260,#31261,#31262,#31263,#31264,#31265,#31266),
 .UNSPECIFIED.,.F.,.F.,(4,3,3,3,3,3,3,3,4),(120.494711874442,120.59929651409,
121.595984915033,122.592673315976,123.589361716919,124.586050117862,125.582738518805,
126.579426919748,126.777897181621),.UNSPECIFIED.);
#421=B_SPLINE_CURVE_WITH_KNOTS('',3,(#31271,#31272,#31273,#31274,#31275,
#31276,#31277,#31278,#31279,#31280,#31281,#31282,#31283,#31284,#31285,#31286,
#31287,#31288,#31289,#31290,#31291,#31292),.UNSPECIFIED.,.F.,.F.,(4,3,3,
3,3,3,3,4),(-136.03943319961,-135.549622528234,-134.552934127291,-133.556245726348,
-132.559557325405,-131.562868924462,-130.566180523519,-129.75624789243),
 .UNSPECIFIED.);
#422=B_SPLINE_CURVE_WITH_KNOTS('',3,(#31293,#31294,#31295,#31296,#31297,
#31298,#31299,#31300,#31301,#31302,#31303,#31304,#31305,#31306,#31307,#31308,
#31309,#31310,#31311,#31312,#31313,#31314),.UNSPECIFIED.,.F.,.F.,(4,3,3,
3,3,3,3,4),(126.777897181621,127.576115320691,128.572803721634,129.569492122576,
130.566180523519,131.562868924462,132.559557325405,133.061082488801),
 .UNSPECIFIED.);
#423=B_SPLINE_CURVE_WITH_KNOTS('',3,(#31319,#31320,#31321,#31322,#31323,
#31324,#31325,#31326,#31327,#31328,#31329,#31330,#31331,#31332,#31333,#31334,
#31335,#31336,#31337,#31338,#31339,#31340),.UNSPECIFIED.,.F.,.F.,(4,3,3,
3,3,3,3,4),(-142.322618506789,-141.529752933891,-140.533064532948,-139.536376132005,
-138.539687731062,-137.54299933012,-136.546310929177,-136.03943319961),
 .UNSPECIFIED.);
#424=B_SPLINE_CURVE_WITH_KNOTS('',3,(#31341,#31342,#31343,#31344,#31345,
#31346,#31347,#31348,#31349,#31350,#31351,#31352,#31353,#31354,#31355,#31356,
#31357,#31358,#31359,#31360,#31361,#31362),.UNSPECIFIED.,.F.,.F.,(4,3,3,
3,3,3,3,4),(133.061082488801,133.556245726348,134.552934127291,135.549622528234,
136.546310929177,137.54299933012,138.539687731063,139.344267795981),
 .UNSPECIFIED.);
#425=B_SPLINE_CURVE_WITH_KNOTS('',3,(#31367,#31368,#31369,#31370,#31371,
#31372,#31373,#31374,#31375,#31376,#31377,#31378,#31379,#31380,#31381,#31382,
#31383,#31384,#31385,#31386,#31387,#31388,#31389,#31390,#31391),
 .UNSPECIFIED.,.F.,.F.,(4,3,3,3,3,3,3,3,4),(-148.605803813969,-148.506571740491,
-147.509883339549,-146.513194938606,-145.516506537663,-144.51981813672,
-143.523129735777,-142.526441334834,-142.322618506789),.UNSPECIFIED.);
#426=B_SPLINE_CURVE_WITH_KNOTS('',3,(#31392,#31393,#31394,#31395,#31396,
#31397,#31398,#31399,#31400,#31401,#31402,#31403,#31404,#31405,#31406,#31407,
#31408,#31409,#31410,#31411,#31412,#31413,#31414,#31415,#31416),
 .UNSPECIFIED.,.F.,.F.,(4,3,3,3,3,3,3,3,4),(139.344267795981,139.536376132005,
140.533064532948,141.529752933891,142.526441334834,143.523129735777,144.51981813672,
145.516506537663,145.62745310316),.UNSPECIFIED.);
#427=B_SPLINE_CURVE_WITH_KNOTS('',3,(#31421,#31422,#31423,#31424,#31425,
#31426,#31427,#31428,#31429,#31430,#31431,#31432,#31433,#31434,#31435,#31436,
#31437,#31438,#31439,#31440,#31441,#31442),.UNSPECIFIED.,.F.,.F.,(4,3,3,
3,3,3,3,4),(-154.888989121148,-154.486702146149,-153.490013745206,-152.493325344263,
-151.49663694332,-150.499948542377,-149.503260141434,-148.605803813969),
 .UNSPECIFIED.);
#428=B_SPLINE_CURVE_WITH_KNOTS('',3,(#31443,#31444,#31445,#31446,#31447,
#31448,#31449,#31450,#31451,#31452,#31453,#31454,#31455,#31456,#31457,#31458,
#31459,#31460,#31461,#31462,#31463,#31464),.UNSPECIFIED.,.F.,.F.,(4,3,3,
3,3,3,3,4),(145.62745310316,146.513194938606,147.509883339549,148.506571740491,
149.503260141434,150.499948542377,151.49663694332,151.91063841034),
 .UNSPECIFIED.);
#429=B_SPLINE_CURVE_WITH_KNOTS('',3,(#31469,#31470,#31471,#31472,#31473,
#31474,#31475,#31476,#31477,#31478,#31479,#31480,#31481,#31482,#31483,#31484,
#31485,#31486,#31487,#31488,#31489,#31490),.UNSPECIFIED.,.F.,.F.,(4,3,3,
3,3,3,3,4),(-161.172174428328,-160.466832551806,-159.470144150863,-158.47345574992,
-157.476767348977,-156.480078948035,-155.483390547092,-154.888989121148),
 .UNSPECIFIED.);
#430=B_SPLINE_CURVE_WITH_KNOTS('',3,(#31491,#31492,#31493,#31494,#31495,
#31496,#31497,#31498,#31499,#31500,#31501,#31502,#31503,#31504,#31505,#31506,
#31507,#31508,#31509,#31510,#31511,#31512),.UNSPECIFIED.,.F.,.F.,(4,3,3,
3,3,3,3,4),(151.91063841034,152.493325344263,153.490013745206,154.486702146149,
155.483390547092,156.480078948035,157.476767348978,158.193823717519),
 .UNSPECIFIED.);
#431=B_SPLINE_CURVE_WITH_KNOTS('',3,(#31517,#31518,#31519,#31520,#31521,
#31522,#31523,#31524,#31525,#31526,#31527,#31528,#31529,#31530,#31531,#31532,
#31533,#31534,#31535,#31536,#31537,#31538,#31539,#31540,#31541),
 .UNSPECIFIED.,.F.,.F.,(4,3,3,3,3,3,3,3,4),(-167.455359735507,-167.443651358406,
-166.446962957464,-165.450274556521,-164.453586155578,-163.456897754635,
-162.460209353692,-161.463520952749,-161.172174428328),.UNSPECIFIED.);
#432=B_SPLINE_CURVE_WITH_KNOTS('',3,(#31542,#31543,#31544,#31545,#31546,
#31547,#31548,#31549,#31550,#31551,#31552,#31553,#31554,#31555,#31556,#31557,
#31558,#31559,#31560,#31561,#31562,#31563,#31564,#31565,#31566),
 .UNSPECIFIED.,.F.,.F.,(4,3,3,3,3,3,3,3,4),(158.193823717519,158.47345574992,
159.470144150863,160.466832551806,161.463520952749,162.460209353692,163.456897754635,
164.453586155578,164.477009024699),.UNSPECIFIED.);
#433=B_SPLINE_CURVE_WITH_KNOTS('',3,(#31571,#31572,#31573,#31574,#31575,
#31576,#31577,#31578,#31579,#31580,#31581,#31582,#31583,#31584,#31585,#31586,
#31587,#31588,#31589,#31590,#31591,#31592),.UNSPECIFIED.,.F.,.F.,(4,3,3,
3,3,3,3,4),(-173.738545042687,-173.423781764064,-172.427093363121,-171.430404962178,
-170.433716561235,-169.437028160292,-168.440339759349,-167.455359735507),
 .UNSPECIFIED.);
#434=B_SPLINE_CURVE_WITH_KNOTS('',3,(#31593,#31594,#31595,#31596,#31597,
#31598,#31599,#31600,#31601,#31602,#31603,#31604,#31605,#31606,#31607,#31608,
#31609,#31610,#31611,#31612,#31613,#31614),.UNSPECIFIED.,.F.,.F.,(4,3,3,
3,3,3,3,4),(164.477009024699,165.450274556521,166.446962957464,167.443651358406,
168.440339759349,169.437028160292,170.433716561235,170.760194331878),
 .UNSPECIFIED.);
#435=B_SPLINE_CURVE_WITH_KNOTS('',3,(#31620,#31621,#31622,#31623,#31624,
#31625),.UNSPECIFIED.,.F.,.F.,(4,1,1,4),(185.353966561798,186.035891684118,
187.03258008506,187.957505154611),.UNSPECIFIED.);
#436=B_SPLINE_CURVE_WITH_KNOTS('',3,(#31628,#31629,#31630,#31631,#31632),
 .UNSPECIFIED.,.F.,.F.,(4,1,4),(185.353966561798,185.721122290575,186.717810691518),
 .UNSPECIFIED.);
#437=B_SPLINE_CURVE_WITH_KNOTS('',3,(#31637,#31638,#31639,#31640,#31641,
#31642,#31643,#31644,#31645,#31646),.UNSPECIFIED.,.F.,.F.,(4,1,1,1,1,1,
1,4),(179.070781254618,180.05576127846,181.052449679403,182.049138080346,
183.045826481289,184.042514882232,185.039203283175,185.353966561798),
 .UNSPECIFIED.);
#438=B_SPLINE_CURVE_WITH_KNOTS('',3,(#31647,#31648,#31649,#31650,#31651,
#31652,#31653,#31654,#31655,#31656),.UNSPECIFIED.,.F.,.F.,(4,1,1,1,1,1,
1,4),(179.070781254618,179.740991884918,180.737680285861,181.734368686804,
182.731057087747,183.72774548869,184.724433889632,185.353966561798),
 .UNSPECIFIED.);
#439=B_SPLINE_CURVE_WITH_KNOTS('',3,(#31661,#31662,#31663,#31664,#31665,
#31666,#31667,#31668,#31669,#31670,#31671),.UNSPECIFIED.,.F.,.F.,(4,1,1,
1,1,1,1,1,4),(172.787595947439,173.07894247186,174.075630872803,175.072319273746,
176.069007674689,177.065696075631,178.062384476574,179.059072877517,179.070781254618),
 .UNSPECIFIED.);
#440=B_SPLINE_CURVE_WITH_KNOTS('',3,(#31672,#31673,#31674,#31675,#31676,
#31677,#31678,#31679,#31680,#31681),.UNSPECIFIED.,.F.,.F.,(4,1,1,1,1,1,
1,4),(172.787595947439,173.760861479261,174.757549880203,175.754238281146,
176.750926682089,177.747615083032,178.744303483975,179.070781254618),
 .UNSPECIFIED.);
#441=B_SPLINE_CURVE_WITH_KNOTS('',3,(#31686,#31687,#31688,#31689,#31690,
#31691,#31692,#31693,#31694,#31695),.UNSPECIFIED.,.F.,.F.,(4,1,1,1,1,1,
1,4),(166.504410640259,167.098812066202,168.095500467145,169.092188868088,
170.088877269031,171.085565669974,172.082254070917,172.787595947439),
 .UNSPECIFIED.);
#442=B_SPLINE_CURVE_WITH_KNOTS('',3,(#31696,#31697,#31698,#31699,#31700,
#31701,#31702,#31703,#31704,#31705,#31706),.UNSPECIFIED.,.F.,.F.,(4,1,1,
1,1,1,1,1,4),(166.504410640259,166.78404267266,167.780731073603,168.777419474546,
169.774107875489,170.770796276432,171.767484677375,172.764173078318,172.787595947439),
 .UNSPECIFIED.);
#443=B_SPLINE_CURVE_WITH_KNOTS('',3,(#31711,#31712,#31713,#31714,#31715,
#31716,#31717,#31718,#31719,#31720),.UNSPECIFIED.,.F.,.F.,(4,1,1,1,1,1,
1,4),(160.22122533308,161.118681660545,162.115370061488,163.112058462431,
164.108746863374,165.105435264317,166.10212366526,166.504410640259),
 .UNSPECIFIED.);
#444=B_SPLINE_CURVE_WITH_KNOTS('',3,(#31721,#31722,#31723,#31724,#31725,
#31726,#31727,#31728,#31729,#31730),.UNSPECIFIED.,.F.,.F.,(4,1,1,1,1,1,
1,4),(160.22122533308,160.803912267003,161.800600667946,162.797289068889,
163.793977469832,164.790665870775,165.787354271717,166.504410640259),
 .UNSPECIFIED.);
#445=B_SPLINE_CURVE_WITH_KNOTS('',3,(#31735,#31736,#31737,#31738,#31739,
#31740,#31741,#31742,#31743,#31744,#31745),.UNSPECIFIED.,.F.,.F.,(4,1,1,
1,1,1,1,1,4),(153.9380400259,154.141862853945,155.138551254888,156.135239655831,
157.131928056774,158.128616457716,159.125304858659,160.121993259602,160.22122533308),
 .UNSPECIFIED.);
#446=B_SPLINE_CURVE_WITH_KNOTS('',3,(#31746,#31747,#31748,#31749,#31750,
#31751,#31752,#31753,#31754,#31755),.UNSPECIFIED.,.F.,.F.,(4,1,1,1,1,1,
1,4),(153.9380400259,154.823781861346,155.820470262288,156.817158663231,
157.813847064174,158.810535465117,159.80722386606,160.22122533308),
 .UNSPECIFIED.);
#447=B_SPLINE_CURVE_WITH_KNOTS('',3,(#31760,#31761,#31762,#31763,#31764,
#31765,#31766,#31767,#31768,#31769),.UNSPECIFIED.,.F.,.F.,(4,1,1,1,1,1,
1,4),(147.65485471872,148.161732448287,149.15842084923,150.155109250173,
151.151797651116,152.148486052059,153.145174453002,153.9380400259),
 .UNSPECIFIED.);
#448=B_SPLINE_CURVE_WITH_KNOTS('',3,(#31770,#31771,#31772,#31773,#31774,
#31775,#31776,#31777,#31778,#31779,#31780),.UNSPECIFIED.,.F.,.F.,(4,1,1,
1,1,1,1,1,4),(147.65485471872,147.846963054745,148.843651455688,149.840339856631,
150.837028257574,151.833716658517,152.83040505946,153.827093460403,153.9380400259),
 .UNSPECIFIED.);
#449=B_SPLINE_CURVE_WITH_KNOTS('',3,(#31785,#31786,#31787,#31788,#31789,
#31790,#31791,#31792,#31793,#31794),.UNSPECIFIED.,.F.,.F.,(4,1,1,1,1,1,
1,4),(141.371669411541,142.18160204263,143.178290443573,144.174978844516,
145.171667245459,146.168355646402,147.165044047345,147.65485471872),
 .UNSPECIFIED.);
#450=B_SPLINE_CURVE_WITH_KNOTS('',3,(#31795,#31796,#31797,#31798,#31799,
#31800,#31801,#31802,#31803,#31804),.UNSPECIFIED.,.F.,.F.,(4,1,1,1,1,1,
1,4),(141.371669411541,141.866832649088,142.863521050031,143.860209450974,
144.856897851917,145.85358625286,146.850274653802,147.65485471872),
 .UNSPECIFIED.);
#451=B_SPLINE_CURVE_WITH_KNOTS('',3,(#31809,#31810,#31811,#31812,#31813,
#31814,#31815,#31816,#31817,#31818,#31819),.UNSPECIFIED.,.F.,.F.,(4,1,1,
1,1,1,1,1,4),(135.088484104361,135.20478323603,136.201471636973,137.198160037916,
138.194848438859,139.191536839801,140.188225240744,141.184913641687,141.371669411541),
 .UNSPECIFIED.);
#452=B_SPLINE_CURVE_WITH_KNOTS('',3,(#31820,#31821,#31822,#31823,#31824,
#31825,#31826,#31827,#31828,#31829),.UNSPECIFIED.,.F.,.F.,(4,1,1,1,1,1,
1,4),(135.088484104361,135.886702243431,136.883390644373,137.880079045316,
138.876767446259,139.873455847202,140.870144248145,141.371669411541),
 .UNSPECIFIED.);
#453=B_SPLINE_CURVE_WITH_KNOTS('',3,(#31834,#31835,#31836,#31837,#31838,
#31839,#31840,#31841,#31842,#31843),.UNSPECIFIED.,.F.,.F.,(4,1,1,1,1,1,
1,4),(128.805298797182,129.224652830372,130.221341231315,131.218029632258,
132.214718033201,133.211406434144,134.208094835087,135.088484104361),
 .UNSPECIFIED.);
#454=B_SPLINE_CURVE_WITH_KNOTS('',3,(#31844,#31845,#31846,#31847,#31848,
#31849,#31850,#31851,#31852,#31853,#31854),.UNSPECIFIED.,.F.,.F.,(4,1,1,
1,1,1,1,1,4),(128.805298797182,128.90988343683,129.906571837773,130.903260238716,
131.899948639659,132.896637040602,133.893325441545,134.890013842488,135.088484104361),
 .UNSPECIFIED.);
#455=B_SPLINE_CURVE_WITH_KNOTS('',3,(#31859,#31860,#31861,#31862,#31863,
#31864,#31865,#31866,#31867,#31868),.UNSPECIFIED.,.F.,.F.,(4,1,1,1,1,1,
1,4),(122.522113490002,123.244522424715,124.241210825658,125.237899226601,
126.234587627544,127.231276028487,128.22796442943,128.805298797182),
 .UNSPECIFIED.);
#456=B_SPLINE_CURVE_WITH_KNOTS('',3,(#31869,#31870,#31871,#31872,#31873,
#31874,#31875,#31876,#31877,#31878),.UNSPECIFIED.,.F.,.F.,(4,1,1,1,1,1,
1,4),(122.522113490002,122.929753031173,123.926441432116,124.923129833059,
125.919818234002,126.916506634944,127.913195035887,128.805298797182),
 .UNSPECIFIED.);
#457=B_SPLINE_CURVE_WITH_KNOTS('',3,(#31883,#31884,#31885,#31886,#31887,
#31888,#31889,#31890,#31891,#31892,#31893),.UNSPECIFIED.,.F.,.F.,(4,1,1,
1,1,1,1,1,4),(116.238928182822,116.267703618115,117.264392019058,118.261080420001,
119.257768820943,120.254457221886,121.251145622829,122.247834023772,122.522113490002),
 .UNSPECIFIED.);
#458=B_SPLINE_CURVE_WITH_KNOTS('',3,(#31894,#31895,#31896,#31897,#31898,
#31899,#31900,#31901,#31902,#31903),.UNSPECIFIED.,.F.,.F.,(4,1,1,1,1,1,
1,4),(116.238928182823,116.949622625516,117.946311026458,118.942999427401,
119.939687828344,120.936376229287,121.93306463023,122.522113490002),
 .UNSPECIFIED.);
#459=B_SPLINE_CURVE_WITH_KNOTS('',3,(#31908,#31909,#31910,#31911,#31912,
#31913,#31914,#31915,#31916,#31917),.UNSPECIFIED.,.F.,.F.,(4,1,1,1,1,1,
1,4),(109.955742875643,110.287573212457,111.2842616134,112.280950014343,
113.277638415286,114.274326816229,115.271015217172,116.238928182822),
 .UNSPECIFIED.);
#460=B_SPLINE_CURVE_WITH_KNOTS('',3,(#31918,#31919,#31920,#31921,#31922,
#31923,#31924,#31925,#31926,#31927,#31928),.UNSPECIFIED.,.F.,.F.,(4,1,1,
1,1,1,1,1,4),(109.955742875643,109.972803818915,110.969492219858,111.966180620801,
112.962869021744,113.959557422687,114.95624582363,115.952934224573,116.238928182823),
 .UNSPECIFIED.);
#461=B_SPLINE_CURVE_WITH_KNOTS('',3,(#31933,#31934,#31935,#31936,#31937,
#31938,#31939,#31940,#31941,#31942),.UNSPECIFIED.,.F.,.F.,(4,1,1,1,1,1,
1,4),(103.672557568463,104.3074428068,105.304131207743,106.300819608686,
107.297508009629,108.294196410572,109.290884811515,109.955742875643),
 .UNSPECIFIED.);
#462=B_SPLINE_CURVE_WITH_KNOTS('',3,(#31943,#31944,#31945,#31946,#31947,
#31948,#31949,#31950,#31951,#31952),.UNSPECIFIED.,.F.,.F.,(4,1,1,1,1,1,
1,4),(103.672557568463,103.992673413258,104.989361814201,105.986050215144,
106.982738616087,107.979427017029,108.976115417972,109.955742875643),
 .UNSPECIFIED.);
#463=B_SPLINE_CURVE_WITH_KNOTS('',3,(#31957,#31958,#31959,#31960,#31961,
#31962,#31963,#31964,#31965,#31966),.UNSPECIFIED.,.F.,.F.,(4,1,1,1,1,1,
1,4),(97.3893722612837,98.3273124011427,99.3240008020856,100.320689203028,
101.317377603971,102.314066004914,103.310754405857,103.672557568463),
 .UNSPECIFIED.);
#464=B_SPLINE_CURVE_WITH_KNOTS('',3,(#31967,#31968,#31969,#31970,#31971,
#31972,#31973,#31974,#31975,#31976),.UNSPECIFIED.,.F.,.F.,(4,1,1,1,1,1,
1,4),(97.3893722612837,98.0125430076005,99.0092314085434,100.005919809486,
101.002608210429,101.999296611372,102.995985012315,103.672557568463),
 .UNSPECIFIED.);
#465=B_SPLINE_CURVE_WITH_KNOTS('',3,(#31981,#31982,#31983,#31984,#31985,
#31986,#31987,#31988,#31989,#31990,#31991),.UNSPECIFIED.,.F.,.F.,(4,1,1,
1,1,1,1,1,4),(91.1061869541041,91.3504935945424,92.3471819954853,93.3438703964282,
94.3405587973711,95.337247198314,96.3339355992569,97.3306240001998,97.3893722612837),
 .UNSPECIFIED.);
#466=B_SPLINE_CURVE_WITH_KNOTS('',3,(#31992,#31993,#31994,#31995,#31996,
#31997,#31998,#31999,#32000,#32001),.UNSPECIFIED.,.F.,.F.,(4,1,1,1,1,1,
1,4),(91.1061869541041,92.0324126019432,93.029101002886,94.0257894038289,
95.0224778047718,96.0191662057147,97.0158546066576,97.3893722612837),
 .UNSPECIFIED.);
#467=B_SPLINE_CURVE_WITH_KNOTS('',3,(#32006,#32007,#32008,#32009,#32010,
#32011,#32012,#32013,#32014,#32015),.UNSPECIFIED.,.F.,.F.,(4,1,1,1,1,1,
1,4),(84.8230016469245,85.3703631888851,86.3670515898279,87.3637399907708,
88.3604283917137,89.3571167926566,90.3538051935995,91.1061869541041),
 .UNSPECIFIED.);
#468=B_SPLINE_CURVE_WITH_KNOTS('',3,(#32016,#32017,#32018,#32019,#32020,
#32021,#32022,#32023,#32024,#32025,#32026),.UNSPECIFIED.,.F.,.F.,(4,1,1,
1,1,1,1,1,4),(84.8230016469246,85.0555937953429,86.0522821962858,87.0489705972287,
88.0456589981716,89.0423473991145,90.0390358000574,91.0357242010002,91.1061869541041),
 .UNSPECIFIED.);
#469=B_SPLINE_CURVE_WITH_KNOTS('',3,(#32031,#32032,#32033,#32034,#32035,
#32036,#32037,#32038,#32039,#32040),.UNSPECIFIED.,.F.,.F.,(4,1,1,1,1,1,
1,4),(78.5398163397449,79.3902327832277,80.3869211841706,81.3836095851135,
82.3802979860564,83.3769863869992,84.3736747879422,84.8230016469245),
 .UNSPECIFIED.);
#470=B_SPLINE_CURVE_WITH_KNOTS('',3,(#32041,#32042,#32043,#32044,#32045,
#32046,#32047,#32048,#32049,#32050),.UNSPECIFIED.,.F.,.F.,(4,1,1,1,1,1,
1,4),(78.539816339745,79.0754633896855,80.0721517906284,81.0688401915713,
82.0655285925142,83.0622169934571,84.0589053944,84.8230016469246),
 .UNSPECIFIED.);
#471=B_SPLINE_CURVE_WITH_KNOTS('',3,(#32055,#32056,#32057,#32058,#32059,
#32060,#32061,#32062,#32063,#32064,#32065),.UNSPECIFIED.,.F.,.F.,(4,1,1,
1,1,1,1,1,4),(72.2566310325653,72.4134139766274,73.4101023775703,74.4067907785132,
75.4034791794561,76.400167580399,77.3968559813419,78.3935443822848,78.5398163397449),
 .UNSPECIFIED.);
#472=B_SPLINE_CURVE_WITH_KNOTS('',3,(#32066,#32067,#32068,#32069,#32070,
#32071,#32072,#32073,#32074,#32075),.UNSPECIFIED.,.F.,.F.,(4,1,1,1,1,1,
1,4),(72.2566310325654,73.0953329840281,74.092021384971,75.0887097859139,
76.0853981868568,77.0820865877997,78.0787749887426,78.539816339745),
 .UNSPECIFIED.);
#473=B_SPLINE_CURVE_WITH_KNOTS('',3,(#32080,#32081,#32082,#32083,#32084,
#32085,#32086,#32087,#32088,#32089),.UNSPECIFIED.,.F.,.F.,(4,1,1,1,1,1,
1,4),(65.9734457253857,66.43328357097,67.4299719719129,68.4266603728558,
69.4233487737987,70.4200371747416,71.4167255756845,72.2566310325653),
 .UNSPECIFIED.);
#474=B_SPLINE_CURVE_WITH_KNOTS('',3,(#32090,#32091,#32092,#32093,#32094,
#32095,#32096,#32097,#32098,#32099,#32100),.UNSPECIFIED.,.F.,.F.,(4,1,1,
1,1,1,1,1,4),(65.9734457253858,66.1185141774279,67.1152025783708,68.1118909793137,
69.1085793802565,70.1052677811994,71.1019561821423,72.0986445830852,72.2566310325654),
 .UNSPECIFIED.);
#475=B_SPLINE_CURVE_WITH_KNOTS('',3,(#32105,#32106,#32107,#32108,#32109,
#32110,#32111,#32112,#32113,#32114),.UNSPECIFIED.,.F.,.F.,(4,1,1,1,1,1,
1,4),(59.6902604182062,60.4531531653127,61.4498415662556,62.4465299671985,
63.4432183681413,64.4399067690842,65.4365951700271,65.9734457253857),
 .UNSPECIFIED.);
#476=B_SPLINE_CURVE_WITH_KNOTS('',3,(#32115,#32116,#32117,#32118,#32119,
#32120,#32121,#32122,#32123,#32124),.UNSPECIFIED.,.F.,.F.,(4,1,1,1,1,1,
1,4),(59.6902604182062,60.1383837717705,61.1350721727134,62.1317605736563,
63.1284489745992,64.1251373755421,65.121825776485,65.9734457253858),
 .UNSPECIFIED.);
#477=B_SPLINE_CURVE_WITH_KNOTS('',3,(#32129,#32130,#32131,#32132,#32133,
#32134,#32135,#32136,#32137,#32138,#32139),.UNSPECIFIED.,.F.,.F.,(4,1,1,
1,1,1,1,1,4),(53.4070751110266,53.4763343587124,54.4730227596553,55.4697111605982,
56.4663995615411,57.463087962484,58.4597763634269,59.4564647643698,59.6902604182062),
 .UNSPECIFIED.);
#478=B_SPLINE_CURVE_WITH_KNOTS('',3,(#32140,#32141,#32142,#32143,#32144,
#32145,#32146,#32147,#32148,#32149),.UNSPECIFIED.,.F.,.F.,(4,1,1,1,1,1,
1,4),(53.4070751110266,54.1582533661131,55.154941767056,56.1516301679989,
57.1483185689418,58.1450069698847,59.1416953708276,59.6902604182062),
 .UNSPECIFIED.);
#479=B_SPLINE_CURVE_WITH_KNOTS('',3,(#32154,#32155,#32156,#32157,#32158,
#32159,#32160,#32161,#32162,#32163),.UNSPECIFIED.,.F.,.F.,(4,1,1,1,1,1,
1,4),(47.123889803847,47.496203953055,48.4928923539979,49.4895807549408,
50.4862691558837,51.4829575568266,52.4796459577695,53.4070751110266),
 .UNSPECIFIED.);
#480=B_SPLINE_CURVE_WITH_KNOTS('',3,(#32164,#32165,#32166,#32167,#32168,
#32169,#32170,#32171,#32172,#32173,#32174),.UNSPECIFIED.,.F.,.F.,(4,1,1,
1,1,1,1,1,4),(47.123889803847,47.1814345595128,48.1781229604557,49.1748113613986,
50.1714997623415,51.1681881632844,52.1648765642273,53.1615649651702,53.4070751110266),
 .UNSPECIFIED.);
#481=B_SPLINE_CURVE_WITH_KNOTS('',3,(#32179,#32180,#32181,#32182,#32183,
#32184,#32185,#32186,#32187,#32188),.UNSPECIFIED.,.F.,.F.,(4,1,1,1,1,1,
1,4),(40.8407044966674,41.5160735473976,42.5127619483405,43.5094503492834,
44.5061387502263,45.5028271511692,46.4995155521121,47.123889803847),
 .UNSPECIFIED.);
#482=B_SPLINE_CURVE_WITH_KNOTS('',3,(#32189,#32190,#32191,#32192,#32193,
#32194,#32195,#32196,#32197,#32198),.UNSPECIFIED.,.F.,.F.,(4,1,1,1,1,1,
1,4),(40.8407044966674,41.2013041538555,42.1979925547984,43.1946809557413,
44.1913693566841,45.188057757627,46.18474615857,47.123889803847),
 .UNSPECIFIED.);
#483=B_SPLINE_CURVE_WITH_KNOTS('',3,(#32203,#32204,#32205,#32206,#32207,
#32208,#32209,#32210,#32211,#32212),.UNSPECIFIED.,.F.,.F.,(4,1,1,1,1,1,
1,4),(34.5575191894878,35.5359431417403,36.5326315426832,37.5293199436261,
38.526008344569,39.5226967455119,40.5193851464548,40.8407044966674),
 .UNSPECIFIED.);
#484=B_SPLINE_CURVE_WITH_KNOTS('',3,(#32213,#32214,#32215,#32216,#32217,
#32218,#32219,#32220,#32221,#32222),.UNSPECIFIED.,.F.,.F.,(4,1,1,1,1,1,
1,4),(34.5575191894878,35.2211737481981,36.217862149141,37.2145505500839,
38.2112389510268,39.2079273519697,40.2046157529126,40.8407044966674),
 .UNSPECIFIED.);
#485=B_SPLINE_CURVE_WITH_KNOTS('',3,(#32227,#32228,#32229,#32230,#32231,
#32232,#32233,#32234,#32235,#32236,#32237),.UNSPECIFIED.,.F.,.F.,(4,1,1,
1,1,1,1,1,4),(28.2743338823082,28.55912433514,29.5558127360829,30.5525011370258,
31.5491895379687,32.5458779389116,33.5425663398545,34.5392547407974,34.5575191894878),
 .UNSPECIFIED.);
#486=B_SPLINE_CURVE_WITH_KNOTS('',3,(#32238,#32239,#32240,#32241,#32242,
#32243,#32244,#32245,#32246,#32247),.UNSPECIFIED.,.F.,.F.,(4,1,1,1,1,1,
1,4),(28.2743338823082,29.2410433425407,30.2377317434836,31.2344201444265,
32.2311085453694,33.2277969463123,34.2244853472552,34.5575191894878),
 .UNSPECIFIED.);
#487=B_SPLINE_CURVE_WITH_KNOTS('',3,(#32252,#32253,#32254,#32255,#32256,
#32257,#32258,#32259,#32260,#32261),.UNSPECIFIED.,.F.,.F.,(4,1,1,1,1,1,
1,4),(21.9911485751286,22.5789939294826,23.5756823304255,24.5723707313684,
25.5690591323113,26.5657475332542,27.5624359341971,28.2743338823082),
 .UNSPECIFIED.);
#488=B_SPLINE_CURVE_WITH_KNOTS('',3,(#32262,#32263,#32264,#32265,#32266,
#32267,#32268,#32269,#32270,#32271,#32272),.UNSPECIFIED.,.F.,.F.,(4,1,1,
1,1,1,1,1,4),(21.9911485751286,22.2642245359404,23.2609129368833,24.2576013378262,
25.2542897387691,26.250978139712,27.2476665406549,28.2443549415978,28.2743338823082),
 .UNSPECIFIED.);
#489=B_SPLINE_CURVE_WITH_KNOTS('',3,(#32277,#32278,#32279,#32280,#32281,
#32282,#32283,#32284,#32285,#32286),.UNSPECIFIED.,.F.,.F.,(4,1,1,1,1,1,
1,4),(15.707963267949,16.5988635238253,17.5955519247682,18.592240325711,
19.5889287266539,20.5856171275968,21.5823055285397,21.9911485751286),
 .UNSPECIFIED.);
#490=B_SPLINE_CURVE_WITH_KNOTS('',3,(#32287,#32288,#32289,#32290,#32291,
#32292,#32293,#32294,#32295,#32296),.UNSPECIFIED.,.F.,.F.,(4,1,1,1,1,1,
1,4),(15.7079632679491,16.2840941302831,17.280782531226,18.2774709321689,
19.2741593331118,20.2708477340547,21.2675361349975,21.9911485751286),
 .UNSPECIFIED.);
#491=B_SPLINE_CURVE_WITH_KNOTS('',3,(#33026,#33027,#33028,#33029,#33030,
#33031,#33032,#33033,#33034,#33035,#33036,#33037,#33038,#33039,#33040,#33041,
#33042,#33043,#33044,#33045,#33046,#33047,#33048,#33049,#33050,#33051,#33052,
#33053,#33054,#33055,#33056,#33057,#33058,#33059,#33060,#33061,#33062,#33063,
#33064,#33065,#33066,#33067,#33068,#33069,#33070,#33071,#33072,#33073,#33074,
#33075,#33076,#33077,#33078,#33079,#33080,#33081,#33082,#33083,#33084,#33085,
#33086,#33087,#33088,#33089,#33090,#33091,#33092,#33093,#33094,#33095,#33096,
#33097,#33098,#33099,#33100,#33101,#33102,#33103,#33104,#33105,#33106,#33107,
#33108,#33109,#33110),.UNSPECIFIED.,.F.,.F.,(4,3,3,3,3,3,3,3,3,3,3,3,3,
3,3,3,3,3,3,3,3,3,3,3,3,3,3,3,4),(-0.364629307890677,-0.350633900072411,
-0.329041704670282,-0.318610240360053,-0.314211809209346,-0.309991562440127,
-0.288669495842773,-0.273343246647572,-0.264936046207356,-0.261282518776684,
-0.240547548924119,-0.220305350751337,-0.206743888633794,-0.195908185817342,
-0.191307393253942,-0.171722665567813,-0.166059502281165,-0.145302064496019,
-0.126512361062532,-0.122942915179013,-0.103486325737185,-0.0841149564703082,
-0.0651452351091335,-0.0617524799581062,-0.0585973862637413,-0.0400118512028539,
-0.0217626000928946,-0.00409409640715274,0.),.UNSPECIFIED.);
#492=B_SPLINE_CURVE_WITH_KNOTS('',3,(#33111,#33112,#33113,#33114,#33115,
#33116,#33117,#33118,#33119,#33120,#33121,#33122,#33123,#33124,#33125,#33126,
#33127,#33128,#33129),.UNSPECIFIED.,.F.,.F.,(4,3,3,3,3,3,4),(170.760194331878,
171.430404962178,172.427093363121,173.423781764064,174.420470165007,175.41715856595,
176.3420836355),.UNSPECIFIED.);
#493=B_SPLINE_CURVE_WITH_KNOTS('',3,(#33131,#33132,#33133,#33134,#33135,
#33136,#33137,#33138,#33139,#33140,#33141,#33142,#33143,#33144,#33145,#33146,
#33147,#33148,#33149,#33150,#33151,#33152,#33153,#33154,#33155,#33156,#33157,
#33158,#33159,#33160,#33161,#33162,#33163,#33164,#33165,#33166,#33167,#33168,
#33169,#33170,#33171,#33172,#33173,#33174,#33175,#33176,#33177,#33178,#33179,
#33180,#33181,#33182,#33183,#33184,#33185,#33186,#33187,#33188,#33189,#33190,
#33191,#33192,#33193,#33194,#33195,#33196,#33197,#33198,#33199,#33200,#33201,
#33202,#33203,#33204,#33205,#33206,#33207,#33208,#33209,#33210,#33211,#33212,
#33213,#33214,#33215,#33216,#33217,#33218),.UNSPECIFIED.,.F.,.F.,(4,3,3,
3,3,3,3,3,3,3,3,3,3,3,3,3,3,3,3,3,3,3,3,3,3,3,3,3,3,4),(-0.366397579005836,
-0.355041886299224,-0.337062787725164,-0.326501278567632,-0.321631321273088,
-0.302824937919741,-0.288343590237545,-0.283403867206792,-0.278586063274018,
-0.259172750250793,-0.239354368340686,-0.226259315371058,-0.219843000340891,
-0.21589805551395,-0.212600028401396,-0.192167406827401,-0.186974156462173,
-0.16726465537396,-0.156579741514883,-0.14850118895299,-0.143866273868592,
-0.123388341850169,-0.102479735695224,-0.0814132858967858,-0.0760794007410636,
-0.0722494160080696,-0.050607200648757,-0.0289135329765765,-0.00768187993829445,
0.),.UNSPECIFIED.);
#494=B_SPLINE_CURVE_WITH_KNOTS('',3,(#33219,#33220,#33221,#33222,#33223,
#33224,#33225,#33226,#33227),.UNSPECIFIED.,.F.,.F.,(4,1,1,1,1,1,4),(10.375727056018,
11.3006521255686,12.2973405265115,13.2940289274544,14.2907173283973,15.2874057293402,
15.7079632679491),.UNSPECIFIED.);
#495=B_SPLINE_CURVE_WITH_KNOTS('',3,(#33233,#33234,#33235,#33236,#33237,
#33238,#33239,#33240,#33241,#33242,#33243,#33244,#33245,#33246,#33247,#33248,
#33249,#33250,#33251,#33252,#33253,#33254,#33255,#33256,#33257,#33258,#33259,
#33260,#33261,#33262,#33263,#33264,#33265,#33266,#33267,#33268,#33269,#33270,
#33271,#33272,#33273,#33274,#33275,#33276,#33277,#33278,#33279,#33280,#33281,
#33282,#33283,#33284,#33285,#33286,#33287,#33288,#33289,#33290,#33291,#33292,
#33293,#33294,#33295,#33296,#33297,#33298,#33299,#33300,#33301,#33302,#33303,
#33304,#33305,#33306,#33307,#33308,#33309,#33310,#33311,#33312,#33313,#33314,
#33315,#33316,#33317),.UNSPECIFIED.,.F.,.F.,(4,3,3,3,3,3,3,3,3,3,3,3,3,
3,3,3,3,3,3,3,3,3,3,3,3,3,3,3,4),(-0.364629307890672,-0.350633900072397,
-0.329041704541407,-0.318610239007672,-0.314211805903378,-0.309991556626561,
-0.288669489872321,-0.273343241423426,-0.264936036487681,-0.261282509824091,
-0.240547539435301,-0.22030533709963,-0.206743878395012,-0.19590817040634,
-0.191307393248018,-0.171722661165846,-0.166059502281157,-0.145302064496012,
-0.126512358429279,-0.122942914832795,-0.103486324429666,-0.0841149582984427,
-0.0651452432836519,-0.0617525129582775,-0.0585973930124723,-0.0400118624810509,
-0.0217626179331671,-0.00409412217882526,0.),.UNSPECIFIED.);
#496=B_SPLINE_CURVE_WITH_KNOTS('',3,(#33320,#33321,#33322,#33323,#33324,
#33325,#33326,#33327),.UNSPECIFIED.,.F.,.F.,(4,1,1,1,1,4),(11.6154215191108,
12.6121099200537,13.6087983209966,14.6054867219395,15.6021751228824,15.707963267949),
 .UNSPECIFIED.);
#497=B_SPLINE_CURVE_WITH_KNOTS('',3,(#34057,#34058,#34059,#34060,#34061,
#34062,#34063,#34064,#34065,#34066,#34067,#34068,#34069,#34070,#34071,#34072,
#34073,#34074,#34075,#34076,#34077,#34078,#34079,#34080,#34081,#34082,#34083,
#34084,#34085,#34086,#34087,#34088,#34089,#34090,#34091,#34092,#34093,#34094,
#34095,#34096,#34097,#34098,#34099,#34100,#34101,#34102,#34103,#34104,#34105,
#34106,#34107,#34108,#34109,#34110,#34111,#34112,#34113,#34114,#34115,#34116,
#34117,#34118,#34119,#34120,#34121,#34122,#34123,#34124,#34125,#34126,#34127,
#34128,#34129,#34130,#34131,#34132,#34133,#34134,#34135,#34136,#34137,#34138,
#34139,#34140,#34141,#34142,#34143,#34144),.UNSPECIFIED.,.F.,.F.,(4,3,3,
3,3,3,3,3,3,3,3,3,3,3,3,3,3,3,3,3,3,3,3,3,3,3,3,3,3,4),(-0.366397579005864,
-0.355041886299263,-0.337062782468908,-0.326501268799074,-0.321631319446025,
-0.302824932606277,-0.288343585588267,-0.28340384950488,-0.278586062019024,
-0.25917274616902,-0.23935436447467,-0.226259312471552,-0.219842994646873,
-0.21589802025165,-0.212599984542311,-0.192167363138322,-0.186974156462199,
-0.16726465363277,-0.156579738901073,-0.14850118045862,-0.143866272303297,
-0.123388338113734,-0.102479729738396,-0.0814132797369128,-0.076079391630003,
-0.0722494180511983,-0.050607201191144,-0.0289135346127569,-0.00768188780162423,
0.),.UNSPECIFIED.);
#498=B_SPLINE_CURVE_WITH_KNOTS('',3,(#34145,#34146,#34147,#34148,#34149,
#34150,#34151,#34152,#34153,#34154,#34155,#34156,#34157,#34158,#34159,#34160),
 .UNSPECIFIED.,.F.,.F.,(4,3,3,3,3,4),(-178.407223768778,-177.410535367835,
-176.413846966892,-175.41715856595,-174.420470165007,-173.738545042687),
 .UNSPECIFIED.);
#499=B_SPLINE_CURVE_WITH_KNOTS('',3,(#34169,#34170,#34171,#34172,#34173,
#34174),.UNSPECIFIED.,.F.,.F.,(4,2,4),(1.11299043816547,1.18225571013767,
1.25152098210987),.UNSPECIFIED.);
#500=B_SPLINE_CURVE_WITH_KNOTS('',3,(#34182,#34183,#34184,#34185,#34186,
#34187),.UNSPECIFIED.,.F.,.F.,(4,2,4),(1.11299043816547,1.18225571013767,
1.25152098210987),.UNSPECIFIED.);
#501=B_SPLINE_CURVE_WITH_KNOTS('',3,(#34193,#34194,#34195,#34196,#34197,
#34198),.UNSPECIFIED.,.F.,.F.,(4,2,4),(1.11299043816547,1.18225571013767,
1.25152098210987),.UNSPECIFIED.);
#502=B_SPLINE_CURVE_WITH_KNOTS('',3,(#34204,#34205,#34206,#34207,#34208,
#34209),.UNSPECIFIED.,.F.,.F.,(4,2,4),(1.11299043816547,1.18225571013767,
1.25152098210987),.UNSPECIFIED.);
#503=B_SPLINE_CURVE_WITH_KNOTS('',3,(#34215,#34216,#34217,#34218,#34219,
#34220),.UNSPECIFIED.,.F.,.F.,(4,2,4),(1.11299043816547,1.18225571013767,
1.25152098210987),.UNSPECIFIED.);
#504=B_SPLINE_CURVE_WITH_KNOTS('',3,(#34225,#34226,#34227,#34228,#34229,
#34230),.UNSPECIFIED.,.F.,.F.,(4,2,4),(1.11299043816547,1.18225571013767,
1.25152098210987),.UNSPECIFIED.);
#597=SHAPE_REPRESENTATION_RELATIONSHIP('SRR','None',#37247,#610);
#610=ADVANCED_BREP_SHAPE_REPRESENTATION('',(#636),#37177);
#623=STYLED_ITEM('',(#37380),#636);
#636=MANIFOLD_SOLID_BREP('Body1',#14785);
#682=FACE_BOUND('',#3006,.T.);
#683=FACE_BOUND('',#3011,.T.);
#851=CYLINDRICAL_SURFACE('',#15917,1.954);
#852=CYLINDRICAL_SURFACE('',#15919,1.954);
#853=CYLINDRICAL_SURFACE('',#15920,1.954);
#854=CYLINDRICAL_SURFACE('',#15921,1.954);
#855=CYLINDRICAL_SURFACE('',#15922,1.954);
#856=CYLINDRICAL_SURFACE('',#15923,1.954);
#857=CYLINDRICAL_SURFACE('',#15924,1.954);
#858=CYLINDRICAL_SURFACE('',#15925,1.954);
#859=CYLINDRICAL_SURFACE('',#15926,1.954);
#860=CYLINDRICAL_SURFACE('',#15927,1.954);
#861=CYLINDRICAL_SURFACE('',#15928,1.954);
#862=CYLINDRICAL_SURFACE('',#15929,1.954);
#863=CYLINDRICAL_SURFACE('',#15930,1.954);
#864=CYLINDRICAL_SURFACE('',#15931,1.954);
#865=CYLINDRICAL_SURFACE('',#15932,1.954);
#866=CYLINDRICAL_SURFACE('',#15933,1.954);
#867=CYLINDRICAL_SURFACE('',#15934,1.954);
#868=CYLINDRICAL_SURFACE('',#15935,1.954);
#869=CYLINDRICAL_SURFACE('',#15936,1.954);
#870=CYLINDRICAL_SURFACE('',#15937,1.954);
#871=CYLINDRICAL_SURFACE('',#15938,1.954);
#872=CYLINDRICAL_SURFACE('',#15939,1.954);
#873=CYLINDRICAL_SURFACE('',#15940,1.954);
#874=CYLINDRICAL_SURFACE('',#15941,1.954);
#875=CYLINDRICAL_SURFACE('',#15942,1.954);
#876=CYLINDRICAL_SURFACE('',#15943,1.954);
#877=CYLINDRICAL_SURFACE('',#15944,1.954);
#878=CYLINDRICAL_SURFACE('',#15945,1.954);
#879=CYLINDRICAL_SURFACE('',#15946,1.5555);
#880=CYLINDRICAL_SURFACE('',#15948,1.5555);
#881=CYLINDRICAL_SURFACE('',#15949,1.5555);
#882=CYLINDRICAL_SURFACE('',#15950,1.5555);
#883=CYLINDRICAL_SURFACE('',#15951,1.5555);
#884=CYLINDRICAL_SURFACE('',#15952,1.5555);
#885=CYLINDRICAL_SURFACE('',#15953,1.5555);
#886=CYLINDRICAL_SURFACE('',#15954,1.5555);
#887=CYLINDRICAL_SURFACE('',#15955,1.5555);
#888=CYLINDRICAL_SURFACE('',#15956,1.5555);
#889=CYLINDRICAL_SURFACE('',#15957,1.5555);
#890=CYLINDRICAL_SURFACE('',#15958,1.5555);
#891=CYLINDRICAL_SURFACE('',#15959,1.5555);
#892=CYLINDRICAL_SURFACE('',#15960,1.5555);
#893=CYLINDRICAL_SURFACE('',#15961,1.5555);
#894=CYLINDRICAL_SURFACE('',#15962,1.5555);
#895=CYLINDRICAL_SURFACE('',#15963,1.5555);
#896=CYLINDRICAL_SURFACE('',#15964,1.5555);
#897=CYLINDRICAL_SURFACE('',#15965,1.5555);
#898=CYLINDRICAL_SURFACE('',#15966,1.5555);
#899=CYLINDRICAL_SURFACE('',#15967,1.5555);
#900=CYLINDRICAL_SURFACE('',#15968,1.5555);
#901=CYLINDRICAL_SURFACE('',#15969,1.5555);
#902=CYLINDRICAL_SURFACE('',#15970,1.5555);
#903=CYLINDRICAL_SURFACE('',#15971,1.5555);
#904=CYLINDRICAL_SURFACE('',#15972,1.5555);
#905=CYLINDRICAL_SURFACE('',#15973,1.5555);
#906=CYLINDRICAL_SURFACE('',#15974,1.5555);
#907=CYLINDRICAL_SURFACE('',#15979,1.5555);
#908=CYLINDRICAL_SURFACE('',#15992,1.954);
#909=CYLINDRICAL_SURFACE('',#15996,3.8);
#1247=CIRCLE('',#15918,1.954);
#1248=CIRCLE('',#15947,1.5555);
#1249=CIRCLE('',#15976,1.954);
#1250=CIRCLE('',#15977,1.954);
#1251=CIRCLE('',#15978,1.5555);
#1252=CIRCLE('',#15981,1.23357587978679);
#1253=CIRCLE('',#15990,1.6);
#1254=CIRCLE('',#15993,1.954);
#1255=CIRCLE('',#15995,3.8);
#1256=CIRCLE('',#15997,3.8);
#1257=CIRCLE('',#15998,3.8);
#1358=CONICAL_SURFACE('',#15980,0.625,1.02388712580674);
#1359=CONICAL_SURFACE('',#15991,1.8,0.785398163397451);
#2056=FACE_OUTER_BOUND('',#2938,.T.);
#2057=FACE_OUTER_BOUND('',#2939,.T.);
#2058=FACE_OUTER_BOUND('',#2940,.T.);
#2059=FACE_OUTER_BOUND('',#2941,.T.);
#2060=FACE_OUTER_BOUND('',#2942,.T.);
#2061=FACE_OUTER_BOUND('',#2943,.T.);
#2062=FACE_OUTER_BOUND('',#2944,.T.);
#2063=FACE_OUTER_BOUND('',#2945,.T.);
#2064=FACE_OUTER_BOUND('',#2946,.T.);
#2065=FACE_OUTER_BOUND('',#2947,.T.);
#2066=FACE_OUTER_BOUND('',#2948,.T.);
#2067=FACE_OUTER_BOUND('',#2949,.T.);
#2068=FACE_OUTER_BOUND('',#2950,.T.);
#2069=FACE_OUTER_BOUND('',#2951,.T.);
#2070=FACE_OUTER_BOUND('',#2952,.T.);
#2071=FACE_OUTER_BOUND('',#2953,.T.);
#2072=FACE_OUTER_BOUND('',#2954,.T.);
#2073=FACE_OUTER_BOUND('',#2955,.T.);
#2074=FACE_OUTER_BOUND('',#2956,.T.);
#2075=FACE_OUTER_BOUND('',#2957,.T.);
#2076=FACE_OUTER_BOUND('',#2958,.T.);
#2077=FACE_OUTER_BOUND('',#2959,.T.);
#2078=FACE_OUTER_BOUND('',#2960,.T.);
#2079=FACE_OUTER_BOUND('',#2961,.T.);
#2080=FACE_OUTER_BOUND('',#2962,.T.);
#2081=FACE_OUTER_BOUND('',#2963,.T.);
#2082=FACE_OUTER_BOUND('',#2964,.T.);
#2083=FACE_OUTER_BOUND('',#2965,.T.);
#2084=FACE_OUTER_BOUND('',#2966,.T.);
#2085=FACE_OUTER_BOUND('',#2967,.T.);
#2086=FACE_OUTER_BOUND('',#2968,.T.);
#2087=FACE_OUTER_BOUND('',#2969,.T.);
#2088=FACE_OUTER_BOUND('',#2970,.T.);
#2089=FACE_OUTER_BOUND('',#2971,.T.);
#2090=FACE_OUTER_BOUND('',#2972,.T.);
#2091=FACE_OUTER_BOUND('',#2973,.T.);
#2092=FACE_OUTER_BOUND('',#2974,.T.);
#2093=FACE_OUTER_BOUND('',#2975,.T.);
#2094=FACE_OUTER_BOUND('',#2976,.T.);
#2095=FACE_OUTER_BOUND('',#2977,.T.);
#2096=FACE_OUTER_BOUND('',#2978,.T.);
#2097=FACE_OUTER_BOUND('',#2979,.T.);
#2098=FACE_OUTER_BOUND('',#2980,.T.);
#2099=FACE_OUTER_BOUND('',#2981,.T.);
#2100=FACE_OUTER_BOUND('',#2982,.T.);
#2101=FACE_OUTER_BOUND('',#2983,.T.);
#2102=FACE_OUTER_BOUND('',#2984,.T.);
#2103=FACE_OUTER_BOUND('',#2985,.T.);
#2104=FACE_OUTER_BOUND('',#2986,.T.);
#2105=FACE_OUTER_BOUND('',#2987,.T.);
#2106=FACE_OUTER_BOUND('',#2988,.T.);
#2107=FACE_OUTER_BOUND('',#2989,.T.);
#2108=FACE_OUTER_BOUND('',#2990,.T.);
#2109=FACE_OUTER_BOUND('',#2991,.T.);
#2110=FACE_OUTER_BOUND('',#2992,.T.);
#2111=FACE_OUTER_BOUND('',#2993,.T.);
#2112=FACE_OUTER_BOUND('',#2994,.T.);
#2113=FACE_OUTER_BOUND('',#2995,.T.);
#2114=FACE_OUTER_BOUND('',#2996,.T.);
#2115=FACE_OUTER_BOUND('',#2997,.T.);
#2116=FACE_OUTER_BOUND('',#2998,.T.);
#2117=FACE_OUTER_BOUND('',#2999,.T.);
#2118=FACE_OUTER_BOUND('',#3000,.T.);
#2119=FACE_OUTER_BOUND('',#3001,.T.);
#2120=FACE_OUTER_BOUND('',#3002,.T.);
#2121=FACE_OUTER_BOUND('',#3003,.T.);
#2122=FACE_OUTER_BOUND('',#3004,.T.);
#2123=FACE_OUTER_BOUND('',#3005,.T.);
#2124=FACE_OUTER_BOUND('',#3007,.T.);
#2125=FACE_OUTER_BOUND('',#3008,.T.);
#2126=FACE_OUTER_BOUND('',#3009,.T.);
#2127=FACE_OUTER_BOUND('',#3010,.T.);
#2128=FACE_OUTER_BOUND('',#3012,.T.);
#2129=FACE_OUTER_BOUND('',#3013,.T.);
#2938=EDGE_LOOP('',(#12629,#12630,#12631,#12632));
#2939=EDGE_LOOP('',(#12633,#12634,#12635,#12636));
#2940=EDGE_LOOP('',(#12637,#12638,#12639,#12640));
#2941=EDGE_LOOP('',(#12641,#12642,#12643,#12644));
#2942=EDGE_LOOP('',(#12645,#12646,#12647,#12648));
#2943=EDGE_LOOP('',(#12649,#12650,#12651,#12652));
#2944=EDGE_LOOP('',(#12653,#12654,#12655,#12656));
#2945=EDGE_LOOP('',(#12657,#12658,#12659,#12660));
#2946=EDGE_LOOP('',(#12661,#12662,#12663,#12664));
#2947=EDGE_LOOP('',(#12665,#12666,#12667,#12668));
#2948=EDGE_LOOP('',(#12669,#12670,#12671,#12672));
#2949=EDGE_LOOP('',(#12673,#12674,#12675,#12676));
#2950=EDGE_LOOP('',(#12677,#12678,#12679,#12680));
#2951=EDGE_LOOP('',(#12681,#12682,#12683,#12684));
#2952=EDGE_LOOP('',(#12685,#12686,#12687,#12688));
#2953=EDGE_LOOP('',(#12689,#12690,#12691,#12692));
#2954=EDGE_LOOP('',(#12693,#12694,#12695,#12696));
#2955=EDGE_LOOP('',(#12697,#12698,#12699,#12700));
#2956=EDGE_LOOP('',(#12701,#12702,#12703,#12704));
#2957=EDGE_LOOP('',(#12705,#12706,#12707,#12708));
#2958=EDGE_LOOP('',(#12709,#12710,#12711,#12712));
#2959=EDGE_LOOP('',(#12713,#12714,#12715,#12716));
#2960=EDGE_LOOP('',(#12717,#12718,#12719,#12720));
#2961=EDGE_LOOP('',(#12721,#12722,#12723,#12724));
#2962=EDGE_LOOP('',(#12725,#12726,#12727,#12728));
#2963=EDGE_LOOP('',(#12729,#12730,#12731,#12732));
#2964=EDGE_LOOP('',(#12733,#12734,#12735,#12736));
#2965=EDGE_LOOP('',(#12737,#12738,#12739,#12740));
#2966=EDGE_LOOP('',(#12741,#12742,#12743,#12744));
#2967=EDGE_LOOP('',(#12745,#12746,#12747,#12748));
#2968=EDGE_LOOP('',(#12749,#12750,#12751,#12752));
#2969=EDGE_LOOP('',(#12753,#12754,#12755,#12756));
#2970=EDGE_LOOP('',(#12757,#12758,#12759,#12760));
#2971=EDGE_LOOP('',(#12761,#12762,#12763,#12764));
#2972=EDGE_LOOP('',(#12765,#12766,#12767,#12768));
#2973=EDGE_LOOP('',(#12769,#12770,#12771,#12772));
#2974=EDGE_LOOP('',(#12773,#12774,#12775,#12776));
#2975=EDGE_LOOP('',(#12777,#12778,#12779,#12780));
#2976=EDGE_LOOP('',(#12781,#12782,#12783,#12784));
#2977=EDGE_LOOP('',(#12785,#12786,#12787,#12788));
#2978=EDGE_LOOP('',(#12789,#12790,#12791,#12792));
#2979=EDGE_LOOP('',(#12793,#12794,#12795,#12796));
#2980=EDGE_LOOP('',(#12797,#12798,#12799,#12800));
#2981=EDGE_LOOP('',(#12801,#12802,#12803,#12804));
#2982=EDGE_LOOP('',(#12805,#12806,#12807,#12808));
#2983=EDGE_LOOP('',(#12809,#12810,#12811,#12812));
#2984=EDGE_LOOP('',(#12813,#12814,#12815,#12816));
#2985=EDGE_LOOP('',(#12817,#12818,#12819,#12820));
#2986=EDGE_LOOP('',(#12821,#12822,#12823,#12824));
#2987=EDGE_LOOP('',(#12825,#12826,#12827,#12828));
#2988=EDGE_LOOP('',(#12829,#12830,#12831,#12832));
#2989=EDGE_LOOP('',(#12833,#12834,#12835,#12836));
#2990=EDGE_LOOP('',(#12837,#12838,#12839,#12840));
#2991=EDGE_LOOP('',(#12841,#12842,#12843,#12844));
#2992=EDGE_LOOP('',(#12845,#12846,#12847,#12848));
#2993=EDGE_LOOP('',(#12849,#12850,#12851,#12852));
#2994=EDGE_LOOP('',(#12853,#12854,#12855,#12856,#12857,#12858,#12859,#12860,
#12861,#12862,#12863,#12864,#12865,#12866,#12867,#12868,#12869,#12870,#12871,
#12872,#12873,#12874,#12875,#12876,#12877,#12878,#12879,#12880,#12881,#12882,
#12883,#12884,#12885,#12886,#12887,#12888,#12889,#12890,#12891,#12892,#12893,
#12894,#12895,#12896,#12897,#12898,#12899,#12900,#12901,#12902,#12903,#12904,
#12905,#12906,#12907,#12908,#12909,#12910,#12911,#12912));
#2995=EDGE_LOOP('',(#12913,#12914,#12915,#12916,#12917));
#2996=EDGE_LOOP('',(#12918,#12919,#12920,#12921));
#2997=EDGE_LOOP('',(#12922,#12923,#12924,#12925,#12926,#12927,#12928,#12929,
#12930,#12931,#12932,#12933,#12934,#12935,#12936,#12937,#12938,#12939,#12940,
#12941,#12942,#12943,#12944,#12945,#12946,#12947,#12948,#12949,#12950,#12951,
#12952,#12953,#12954,#12955,#12956,#12957,#12958,#12959,#12960,#12961,#12962,
#12963,#12964,#12965,#12966,#12967,#12968,#12969,#12970,#12971,#12972,#12973,
#12974,#12975,#12976,#12977,#12978,#12979,#12980,#12981));
#2998=EDGE_LOOP('',(#12982,#12983,#12984));
#2999=EDGE_LOOP('',(#12985,#12986,#12987,#12988));
#3000=EDGE_LOOP('',(#12989,#12990,#12991,#12992));
#3001=EDGE_LOOP('',(#12993,#12994,#12995,#12996));
#3002=EDGE_LOOP('',(#12997,#12998,#12999,#13000));
#3003=EDGE_LOOP('',(#13001,#13002,#13003,#13004));
#3004=EDGE_LOOP('',(#13005,#13006,#13007,#13008));
#3005=EDGE_LOOP('',(#13009,#13010,#13011,#13012,#13013,#13014));
#3006=EDGE_LOOP('',(#13015));
#3007=EDGE_LOOP('',(#13016));
#3008=EDGE_LOOP('',(#13017,#13018,#13019,#13020,#13021,#13022));
#3009=EDGE_LOOP('',(#13023,#13024,#13025,#13026));
#3010=EDGE_LOOP('',(#13027));
#3011=EDGE_LOOP('',(#13028,#13029,#13030,#13031));
#3012=EDGE_LOOP('',(#13032,#13033,#13034,#13035,#13036));
#3013=EDGE_LOOP('',(#13037,#13038,#13039,#13040,#13041,#13042,#13043,#13044,
#13045,#13046));
#3175=(
BOUNDED_CURVE()
B_SPLINE_CURVE(2,(#34276,#34277,#34278),.UNSPECIFIED.,.F.,.F.)
B_SPLINE_CURVE_WITH_KNOTS((3,3),(-1.30181351501822,-0.516279708895519),
 .UNSPECIFIED.)
CURVE()
GEOMETRIC_REPRESENTATION_ITEM()
RATIONAL_B_SPLINE_CURVE((0.98985802419273,0.918917809350684,1.))
REPRESENTATION_ITEM('')
);
#4300=LINE('',#30250,#5539);
#4301=LINE('',#30274,#5540);
#4302=LINE('',#30322,#5541);
#4303=LINE('',#30370,#5542);
#4304=LINE('',#30424,#5543);
#4305=LINE('',#30472,#5544);
#4306=LINE('',#30520,#5545);
#4307=LINE('',#30568,#5546);
#4308=LINE('',#30622,#5547);
#4309=LINE('',#30670,#5548);
#4310=LINE('',#30718,#5549);
#4311=LINE('',#30772,#5550);
#4312=LINE('',#30820,#5551);
#4313=LINE('',#30868,#5552);
#4314=LINE('',#30922,#5553);
#4315=LINE('',#30970,#5554);
#4316=LINE('',#31018,#5555);
#4317=LINE('',#31066,#5556);
#4318=LINE('',#31120,#5557);
#4319=LINE('',#31168,#5558);
#4320=LINE('',#31216,#5559);
#4321=LINE('',#31270,#5560);
#4322=LINE('',#31318,#5561);
#4323=LINE('',#31366,#5562);
#4324=LINE('',#31420,#5563);
#4325=LINE('',#31468,#5564);
#4326=LINE('',#31516,#5565);
#4327=LINE('',#31570,#5566);
#4328=LINE('',#31618,#5567);
#4329=LINE('',#31636,#5568);
#4330=LINE('',#31660,#5569);
#4331=LINE('',#31685,#5570);
#4332=LINE('',#31710,#5571);
#4333=LINE('',#31734,#5572);
#4334=LINE('',#31759,#5573);
#4335=LINE('',#31784,#5574);
#4336=LINE('',#31808,#5575);
#4337=LINE('',#31833,#5576);
#4338=LINE('',#31858,#5577);
#4339=LINE('',#31882,#5578);
#4340=LINE('',#31907,#5579);
#4341=LINE('',#31932,#5580);
#4342=LINE('',#31956,#5581);
#4343=LINE('',#31980,#5582);
#4344=LINE('',#32005,#5583);
#4345=LINE('',#32030,#5584);
#4346=LINE('',#32054,#5585);
#4347=LINE('',#32079,#5586);
#4348=LINE('',#32104,#5587);
#4349=LINE('',#32128,#5588);
#4350=LINE('',#32153,#5589);
#4351=LINE('',#32178,#5590);
#4352=LINE('',#32202,#5591);
#4353=LINE('',#32226,#5592);
#4354=LINE('',#32251,#5593);
#4355=LINE('',#32276,#5594);
#4356=LINE('',#34164,#5595);
#4357=LINE('',#34176,#5596);
#4358=LINE('',#34178,#5597);
#4359=LINE('',#34179,#5598);
#4360=LINE('',#34189,#5599);
#4361=LINE('',#34190,#5600);
#4362=LINE('',#34200,#5601);
#4363=LINE('',#34201,#5602);
#4364=LINE('',#34211,#5603);
#4365=LINE('',#34212,#5604);
#4366=LINE('',#34222,#5605);
#4367=LINE('',#34223,#5606);
#4368=LINE('',#34231,#5607);
#4369=LINE('',#34237,#5608);
#4370=LINE('',#34247,#5609);
#5539=VECTOR('',#19192,2.);
#5540=VECTOR('',#19197,2.);
#5541=VECTOR('',#19200,2.);
#5542=VECTOR('',#19203,2.);
#5543=VECTOR('',#19206,2.);
#5544=VECTOR('',#19209,2.);
#5545=VECTOR('',#19212,2.);
#5546=VECTOR('',#19215,2.);
#5547=VECTOR('',#19218,2.);
#5548=VECTOR('',#19221,2.);
#5549=VECTOR('',#19224,2.);
#5550=VECTOR('',#19227,2.);
#5551=VECTOR('',#19230,2.);
#5552=VECTOR('',#19233,2.);
#5553=VECTOR('',#19236,2.);
#5554=VECTOR('',#19239,2.);
#5555=VECTOR('',#19242,2.);
#5556=VECTOR('',#19245,2.);
#5557=VECTOR('',#19248,2.);
#5558=VECTOR('',#19251,2.);
#5559=VECTOR('',#19254,2.);
#5560=VECTOR('',#19257,2.);
#5561=VECTOR('',#19260,2.);
#5562=VECTOR('',#19263,2.);
#5563=VECTOR('',#19266,2.);
#5564=VECTOR('',#19269,2.);
#5565=VECTOR('',#19272,2.);
#5566=VECTOR('',#19275,2.);
#5567=VECTOR('',#19278,1.5555);
#5568=VECTOR('',#19283,1.5555);
#5569=VECTOR('',#19286,1.5555);
#5570=VECTOR('',#19289,1.5555);
#5571=VECTOR('',#19292,1.5555);
#5572=VECTOR('',#19295,1.5555);
#5573=VECTOR('',#19298,1.5555);
#5574=VECTOR('',#19301,1.5555);
#5575=VECTOR('',#19304,1.5555);
#5576=VECTOR('',#19307,1.5555);
#5577=VECTOR('',#19310,1.5555);
#5578=VECTOR('',#19313,1.5555);
#5579=VECTOR('',#19316,1.5555);
#5580=VECTOR('',#19319,1.5555);
#5581=VECTOR('',#19322,1.5555);
#5582=VECTOR('',#19325,1.5555);
#5583=VECTOR('',#19328,1.5555);
#5584=VECTOR('',#19331,1.5555);
#5585=VECTOR('',#19334,1.5555);
#5586=VECTOR('',#19337,1.5555);
#5587=VECTOR('',#19340,1.5555);
#5588=VECTOR('',#19343,1.5555);
#5589=VECTOR('',#19346,1.5555);
#5590=VECTOR('',#19349,1.5555);
#5591=VECTOR('',#19352,1.5555);
#5592=VECTOR('',#19355,1.5555);
#5593=VECTOR('',#19358,1.5555);
#5594=VECTOR('',#19361,1.5555);
#5595=VECTOR('',#19374,0.625);
#5596=VECTOR('',#19379,10.);
#5597=VECTOR('',#19380,10.);
#5598=VECTOR('',#19381,10.);
#5599=VECTOR('',#19384,10.);
#5600=VECTOR('',#19385,10.);
#5601=VECTOR('',#19388,10.);
#5602=VECTOR('',#19389,10.);
#5603=VECTOR('',#19392,10.);
#5604=VECTOR('',#19393,10.);
#5605=VECTOR('',#19396,10.);
#5606=VECTOR('',#19397,10.);
#5607=VECTOR('',#19400,10.);
#5608=VECTOR('',#19409,1.8);
#5609=VECTOR('',#19422,3.8);
#6752=VERTEX_POINT('',#30248);
#6753=VERTEX_POINT('',#30249);
#6754=VERTEX_POINT('',#30251);
#6755=VERTEX_POINT('',#30262);
#6756=VERTEX_POINT('',#30272);
#6757=VERTEX_POINT('',#30273);
#6758=VERTEX_POINT('',#30320);
#6759=VERTEX_POINT('',#30321);
#6760=VERTEX_POINT('',#30368);
#6761=VERTEX_POINT('',#30369);
#6762=VERTEX_POINT('',#30422);
#6763=VERTEX_POINT('',#30423);
#6764=VERTEX_POINT('',#30470);
#6765=VERTEX_POINT('',#30471);
#6766=VERTEX_POINT('',#30518);
#6767=VERTEX_POINT('',#30519);
#6768=VERTEX_POINT('',#30566);
#6769=VERTEX_POINT('',#30567);
#6770=VERTEX_POINT('',#30620);
#6771=VERTEX_POINT('',#30621);
#6772=VERTEX_POINT('',#30668);
#6773=VERTEX_POINT('',#30669);
#6774=VERTEX_POINT('',#30716);
#6775=VERTEX_POINT('',#30717);
#6776=VERTEX_POINT('',#30770);
#6777=VERTEX_POINT('',#30771);
#6778=VERTEX_POINT('',#30818);
#6779=VERTEX_POINT('',#30819);
#6780=VERTEX_POINT('',#30866);
#6781=VERTEX_POINT('',#30867);
#6782=VERTEX_POINT('',#30920);
#6783=VERTEX_POINT('',#30921);
#6784=VERTEX_POINT('',#30968);
#6785=VERTEX_POINT('',#30969);
#6786=VERTEX_POINT('',#31016);
#6787=VERTEX_POINT('',#31017);
#6788=VERTEX_POINT('',#31064);
#6789=VERTEX_POINT('',#31065);
#6790=VERTEX_POINT('',#31118);
#6791=VERTEX_POINT('',#31119);
#6792=VERTEX_POINT('',#31166);
#6793=VERTEX_POINT('',#31167);
#6794=VERTEX_POINT('',#31214);
#6795=VERTEX_POINT('',#31215);
#6796=VERTEX_POINT('',#31268);
#6797=VERTEX_POINT('',#31269);
#6798=VERTEX_POINT('',#31316);
#6799=VERTEX_POINT('',#31317);
#6800=VERTEX_POINT('',#31364);
#6801=VERTEX_POINT('',#31365);
#6802=VERTEX_POINT('',#31418);
#6803=VERTEX_POINT('',#31419);
#6804=VERTEX_POINT('',#31466);
#6805=VERTEX_POINT('',#31467);
#6806=VERTEX_POINT('',#31514);
#6807=VERTEX_POINT('',#31515);
#6808=VERTEX_POINT('',#31568);
#6809=VERTEX_POINT('',#31569);
#6810=VERTEX_POINT('',#31616);
#6811=VERTEX_POINT('',#31617);
#6812=VERTEX_POINT('',#31619);
#6813=VERTEX_POINT('',#31626);
#6814=VERTEX_POINT('',#31634);
#6815=VERTEX_POINT('',#31635);
#6816=VERTEX_POINT('',#31658);
#6817=VERTEX_POINT('',#31659);
#6818=VERTEX_POINT('',#31683);
#6819=VERTEX_POINT('',#31684);
#6820=VERTEX_POINT('',#31708);
#6821=VERTEX_POINT('',#31709);
#6822=VERTEX_POINT('',#31732);
#6823=VERTEX_POINT('',#31733);
#6824=VERTEX_POINT('',#31757);
#6825=VERTEX_POINT('',#31758);
#6826=VERTEX_POINT('',#31782);
#6827=VERTEX_POINT('',#31783);
#6828=VERTEX_POINT('',#31806);
#6829=VERTEX_POINT('',#31807);
#6830=VERTEX_POINT('',#31831);
#6831=VERTEX_POINT('',#31832);
#6832=VERTEX_POINT('',#31856);
#6833=VERTEX_POINT('',#31857);
#6834=VERTEX_POINT('',#31880);
#6835=VERTEX_POINT('',#31881);
#6836=VERTEX_POINT('',#31905);
#6837=VERTEX_POINT('',#31906);
#6838=VERTEX_POINT('',#31930);
#6839=VERTEX_POINT('',#31931);
#6840=VERTEX_POINT('',#31954);
#6841=VERTEX_POINT('',#31955);
#6842=VERTEX_POINT('',#31978);
#6843=VERTEX_POINT('',#31979);
#6844=VERTEX_POINT('',#32003);
#6845=VERTEX_POINT('',#32004);
#6846=VERTEX_POINT('',#32028);
#6847=VERTEX_POINT('',#32029);
#6848=VERTEX_POINT('',#32052);
#6849=VERTEX_POINT('',#32053);
#6850=VERTEX_POINT('',#32077);
#6851=VERTEX_POINT('',#32078);
#6852=VERTEX_POINT('',#32102);
#6853=VERTEX_POINT('',#32103);
#6854=VERTEX_POINT('',#32126);
#6855=VERTEX_POINT('',#32127);
#6856=VERTEX_POINT('',#32151);
#6857=VERTEX_POINT('',#32152);
#6858=VERTEX_POINT('',#32176);
#6859=VERTEX_POINT('',#32177);
#6860=VERTEX_POINT('',#32200);
#6861=VERTEX_POINT('',#32201);
#6862=VERTEX_POINT('',#32224);
#6863=VERTEX_POINT('',#32225);
#6864=VERTEX_POINT('',#32249);
#6865=VERTEX_POINT('',#32250);
#6866=VERTEX_POINT('',#32274);
#6867=VERTEX_POINT('',#32275);
#6868=VERTEX_POINT('',#33025);
#6869=VERTEX_POINT('',#33130);
#6870=VERTEX_POINT('',#33229);
#6871=VERTEX_POINT('',#33232);
#6872=VERTEX_POINT('',#34056);
#6873=VERTEX_POINT('',#34162);
#6874=VERTEX_POINT('',#34163);
#6875=VERTEX_POINT('',#34167);
#6876=VERTEX_POINT('',#34168);
#6877=VERTEX_POINT('',#34175);
#6878=VERTEX_POINT('',#34177);
#6879=VERTEX_POINT('',#34181);
#6880=VERTEX_POINT('',#34188);
#6881=VERTEX_POINT('',#34192);
#6882=VERTEX_POINT('',#34199);
#6883=VERTEX_POINT('',#34203);
#6884=VERTEX_POINT('',#34210);
#6885=VERTEX_POINT('',#34214);
#6886=VERTEX_POINT('',#34221);
#6887=VERTEX_POINT('',#34234);
#6888=VERTEX_POINT('',#34241);
#6889=VERTEX_POINT('',#34244);
#6890=VERTEX_POINT('',#34245);
#8756=EDGE_CURVE('',#6752,#6753,#4300,.T.);
#8757=EDGE_CURVE('',#6752,#6754,#379,.T.);
#8758=EDGE_CURVE('',#6754,#6755,#1247,.T.);
#8759=EDGE_CURVE('',#6755,#6753,#380,.T.);
#8760=EDGE_CURVE('',#6756,#6757,#4301,.T.);
#8761=EDGE_CURVE('',#6756,#6752,#381,.T.);
#8762=EDGE_CURVE('',#6753,#6757,#382,.T.);
#8763=EDGE_CURVE('',#6758,#6759,#4302,.T.);
#8764=EDGE_CURVE('',#6758,#6756,#383,.T.);
#8765=EDGE_CURVE('',#6757,#6759,#384,.T.);
#8766=EDGE_CURVE('',#6760,#6761,#4303,.T.);
#8767=EDGE_CURVE('',#6760,#6758,#385,.T.);
#8768=EDGE_CURVE('',#6759,#6761,#386,.T.);
#8769=EDGE_CURVE('',#6762,#6763,#4304,.T.);
#8770=EDGE_CURVE('',#6762,#6760,#387,.T.);
#8771=EDGE_CURVE('',#6761,#6763,#388,.T.);
#8772=EDGE_CURVE('',#6764,#6765,#4305,.T.);
#8773=EDGE_CURVE('',#6764,#6762,#389,.T.);
#8774=EDGE_CURVE('',#6763,#6765,#390,.T.);
#8775=EDGE_CURVE('',#6766,#6767,#4306,.T.);
#8776=EDGE_CURVE('',#6766,#6764,#391,.T.);
#8777=EDGE_CURVE('',#6765,#6767,#392,.T.);
#8778=EDGE_CURVE('',#6768,#6769,#4307,.T.);
#8779=EDGE_CURVE('',#6768,#6766,#393,.T.);
#8780=EDGE_CURVE('',#6767,#6769,#394,.T.);
#8781=EDGE_CURVE('',#6770,#6771,#4308,.T.);
#8782=EDGE_CURVE('',#6770,#6768,#395,.T.);
#8783=EDGE_CURVE('',#6769,#6771,#396,.T.);
#8784=EDGE_CURVE('',#6772,#6773,#4309,.T.);
#8785=EDGE_CURVE('',#6772,#6770,#397,.T.);
#8786=EDGE_CURVE('',#6771,#6773,#398,.T.);
#8787=EDGE_CURVE('',#6774,#6775,#4310,.T.);
#8788=EDGE_CURVE('',#6774,#6772,#399,.T.);
#8789=EDGE_CURVE('',#6773,#6775,#400,.T.);
#8790=EDGE_CURVE('',#6776,#6777,#4311,.T.);
#8791=EDGE_CURVE('',#6776,#6774,#401,.T.);
#8792=EDGE_CURVE('',#6775,#6777,#402,.T.);
#8793=EDGE_CURVE('',#6778,#6779,#4312,.T.);
#8794=EDGE_CURVE('',#6778,#6776,#403,.T.);
#8795=EDGE_CURVE('',#6777,#6779,#404,.T.);
#8796=EDGE_CURVE('',#6780,#6781,#4313,.T.);
#8797=EDGE_CURVE('',#6780,#6778,#405,.T.);
#8798=EDGE_CURVE('',#6779,#6781,#406,.T.);
#8799=EDGE_CURVE('',#6782,#6783,#4314,.T.);
#8800=EDGE_CURVE('',#6782,#6780,#407,.T.);
#8801=EDGE_CURVE('',#6781,#6783,#408,.T.);
#8802=EDGE_CURVE('',#6784,#6785,#4315,.T.);
#8803=EDGE_CURVE('',#6784,#6782,#409,.T.);
#8804=EDGE_CURVE('',#6783,#6785,#410,.T.);
#8805=EDGE_CURVE('',#6786,#6787,#4316,.T.);
#8806=EDGE_CURVE('',#6786,#6784,#411,.T.);
#8807=EDGE_CURVE('',#6785,#6787,#412,.T.);
#8808=EDGE_CURVE('',#6788,#6789,#4317,.T.);
#8809=EDGE_CURVE('',#6788,#6786,#413,.T.);
#8810=EDGE_CURVE('',#6787,#6789,#414,.T.);
#8811=EDGE_CURVE('',#6790,#6791,#4318,.T.);
#8812=EDGE_CURVE('',#6790,#6788,#415,.T.);
#8813=EDGE_CURVE('',#6789,#6791,#416,.T.);
#8814=EDGE_CURVE('',#6792,#6793,#4319,.T.);
#8815=EDGE_CURVE('',#6792,#6790,#417,.T.);
#8816=EDGE_CURVE('',#6791,#6793,#418,.T.);
#8817=EDGE_CURVE('',#6794,#6795,#4320,.T.);
#8818=EDGE_CURVE('',#6794,#6792,#419,.T.);
#8819=EDGE_CURVE('',#6793,#6795,#420,.T.);
#8820=EDGE_CURVE('',#6796,#6797,#4321,.T.);
#8821=EDGE_CURVE('',#6796,#6794,#421,.T.);
#8822=EDGE_CURVE('',#6795,#6797,#422,.T.);
#8823=EDGE_CURVE('',#6798,#6799,#4322,.T.);
#8824=EDGE_CURVE('',#6798,#6796,#423,.T.);
#8825=EDGE_CURVE('',#6797,#6799,#424,.T.);
#8826=EDGE_CURVE('',#6800,#6801,#4323,.T.);
#8827=EDGE_CURVE('',#6800,#6798,#425,.T.);
#8828=EDGE_CURVE('',#6799,#6801,#426,.T.);
#8829=EDGE_CURVE('',#6802,#6803,#4324,.T.);
#8830=EDGE_CURVE('',#6802,#6800,#427,.T.);
#8831=EDGE_CURVE('',#6801,#6803,#428,.T.);
#8832=EDGE_CURVE('',#6804,#6805,#4325,.T.);
#8833=EDGE_CURVE('',#6804,#6802,#429,.T.);
#8834=EDGE_CURVE('',#6803,#6805,#430,.T.);
#8835=EDGE_CURVE('',#6806,#6807,#4326,.T.);
#8836=EDGE_CURVE('',#6806,#6804,#431,.T.);
#8837=EDGE_CURVE('',#6805,#6807,#432,.T.);
#8838=EDGE_CURVE('',#6808,#6809,#4327,.T.);
#8839=EDGE_CURVE('',#6808,#6806,#433,.T.);
#8840=EDGE_CURVE('',#6807,#6809,#434,.T.);
#8841=EDGE_CURVE('',#6810,#6811,#4328,.T.);
#8842=EDGE_CURVE('',#6810,#6812,#435,.T.);
#8843=EDGE_CURVE('',#6813,#6812,#1248,.T.);
#8844=EDGE_CURVE('',#6811,#6813,#436,.T.);
#8845=EDGE_CURVE('',#6814,#6815,#4329,.T.);
#8846=EDGE_CURVE('',#6814,#6810,#437,.T.);
#8847=EDGE_CURVE('',#6815,#6811,#438,.T.);
#8848=EDGE_CURVE('',#6816,#6817,#4330,.T.);
#8849=EDGE_CURVE('',#6816,#6814,#439,.T.);
#8850=EDGE_CURVE('',#6817,#6815,#440,.T.);
#8851=EDGE_CURVE('',#6818,#6819,#4331,.T.);
#8852=EDGE_CURVE('',#6818,#6816,#441,.T.);
#8853=EDGE_CURVE('',#6819,#6817,#442,.T.);
#8854=EDGE_CURVE('',#6820,#6821,#4332,.T.);
#8855=EDGE_CURVE('',#6820,#6818,#443,.T.);
#8856=EDGE_CURVE('',#6821,#6819,#444,.T.);
#8857=EDGE_CURVE('',#6822,#6823,#4333,.T.);
#8858=EDGE_CURVE('',#6822,#6820,#445,.T.);
#8859=EDGE_CURVE('',#6823,#6821,#446,.T.);
#8860=EDGE_CURVE('',#6824,#6825,#4334,.T.);
#8861=EDGE_CURVE('',#6824,#6822,#447,.T.);
#8862=EDGE_CURVE('',#6825,#6823,#448,.T.);
#8863=EDGE_CURVE('',#6826,#6827,#4335,.T.);
#8864=EDGE_CURVE('',#6826,#6824,#449,.T.);
#8865=EDGE_CURVE('',#6827,#6825,#450,.T.);
#8866=EDGE_CURVE('',#6828,#6829,#4336,.T.);
#8867=EDGE_CURVE('',#6828,#6826,#451,.T.);
#8868=EDGE_CURVE('',#6829,#6827,#452,.T.);
#8869=EDGE_CURVE('',#6830,#6831,#4337,.T.);
#8870=EDGE_CURVE('',#6830,#6828,#453,.T.);
#8871=EDGE_CURVE('',#6831,#6829,#454,.T.);
#8872=EDGE_CURVE('',#6832,#6833,#4338,.T.);
#8873=EDGE_CURVE('',#6832,#6830,#455,.T.);
#8874=EDGE_CURVE('',#6833,#6831,#456,.T.);
#8875=EDGE_CURVE('',#6834,#6835,#4339,.T.);
#8876=EDGE_CURVE('',#6834,#6832,#457,.T.);
#8877=EDGE_CURVE('',#6835,#6833,#458,.T.);
#8878=EDGE_CURVE('',#6836,#6837,#4340,.T.);
#8879=EDGE_CURVE('',#6836,#6834,#459,.T.);
#8880=EDGE_CURVE('',#6837,#6835,#460,.T.);
#8881=EDGE_CURVE('',#6838,#6839,#4341,.T.);
#8882=EDGE_CURVE('',#6838,#6836,#461,.T.);
#8883=EDGE_CURVE('',#6839,#6837,#462,.T.);
#8884=EDGE_CURVE('',#6840,#6841,#4342,.T.);
#8885=EDGE_CURVE('',#6840,#6838,#463,.T.);
#8886=EDGE_CURVE('',#6841,#6839,#464,.T.);
#8887=EDGE_CURVE('',#6842,#6843,#4343,.T.);
#8888=EDGE_CURVE('',#6842,#6840,#465,.T.);
#8889=EDGE_CURVE('',#6843,#6841,#466,.T.);
#8890=EDGE_CURVE('',#6844,#6845,#4344,.T.);
#8891=EDGE_CURVE('',#6844,#6842,#467,.T.);
#8892=EDGE_CURVE('',#6845,#6843,#468,.T.);
#8893=EDGE_CURVE('',#6846,#6847,#4345,.T.);
#8894=EDGE_CURVE('',#6846,#6844,#469,.T.);
#8895=EDGE_CURVE('',#6847,#6845,#470,.T.);
#8896=EDGE_CURVE('',#6848,#6849,#4346,.T.);
#8897=EDGE_CURVE('',#6848,#6846,#471,.T.);
#8898=EDGE_CURVE('',#6849,#6847,#472,.T.);
#8899=EDGE_CURVE('',#6850,#6851,#4347,.T.);
#8900=EDGE_CURVE('',#6850,#6848,#473,.T.);
#8901=EDGE_CURVE('',#6851,#6849,#474,.T.);
#8902=EDGE_CURVE('',#6852,#6853,#4348,.T.);
#8903=EDGE_CURVE('',#6852,#6850,#475,.T.);
#8904=EDGE_CURVE('',#6853,#6851,#476,.T.);
#8905=EDGE_CURVE('',#6854,#6855,#4349,.T.);
#8906=EDGE_CURVE('',#6854,#6852,#477,.T.);
#8907=EDGE_CURVE('',#6855,#6853,#478,.T.);
#8908=EDGE_CURVE('',#6856,#6857,#4350,.T.);
#8909=EDGE_CURVE('',#6856,#6854,#479,.T.);
#8910=EDGE_CURVE('',#6857,#6855,#480,.T.);
#8911=EDGE_CURVE('',#6858,#6859,#4351,.T.);
#8912=EDGE_CURVE('',#6858,#6856,#481,.T.);
#8913=EDGE_CURVE('',#6859,#6857,#482,.T.);
#8914=EDGE_CURVE('',#6860,#6861,#4352,.T.);
#8915=EDGE_CURVE('',#6860,#6858,#483,.T.);
#8916=EDGE_CURVE('',#6861,#6859,#484,.T.);
#8917=EDGE_CURVE('',#6862,#6863,#4353,.T.);
#8918=EDGE_CURVE('',#6862,#6860,#485,.T.);
#8919=EDGE_CURVE('',#6863,#6861,#486,.T.);
#8920=EDGE_CURVE('',#6864,#6865,#4354,.T.);
#8921=EDGE_CURVE('',#6864,#6862,#487,.T.);
#8922=EDGE_CURVE('',#6865,#6863,#488,.T.);
#8923=EDGE_CURVE('',#6866,#6867,#4355,.T.);
#8924=EDGE_CURVE('',#6866,#6864,#489,.T.);
#8925=EDGE_CURVE('',#6867,#6865,#490,.T.);
#8926=EDGE_CURVE('',#6868,#6813,#491,.T.);
#8927=EDGE_CURVE('',#6809,#6868,#492,.T.);
#8928=EDGE_CURVE('',#6869,#6755,#493,.T.);
#8929=EDGE_CURVE('',#6869,#6867,#494,.T.);
#8930=EDGE_CURVE('',#6755,#6870,#1249,.T.);
#8931=EDGE_CURVE('',#6870,#6754,#1250,.T.);
#8932=EDGE_CURVE('',#6754,#6871,#495,.T.);
#8933=EDGE_CURVE('',#6871,#6869,#1251,.T.);
#8934=EDGE_CURVE('',#6871,#6866,#496,.T.);
#8935=EDGE_CURVE('',#6812,#6872,#497,.T.);
#8936=EDGE_CURVE('',#6872,#6808,#498,.T.);
#8937=EDGE_CURVE('',#6873,#6874,#4356,.T.);
#8938=EDGE_CURVE('',#6874,#6874,#1252,.T.);
#8939=EDGE_CURVE('',#6875,#6876,#499,.T.);
#8940=EDGE_CURVE('',#6875,#6877,#4357,.T.);
#8941=EDGE_CURVE('',#6877,#6878,#4358,.T.);
#8942=EDGE_CURVE('',#6876,#6878,#4359,.T.);
#8943=EDGE_CURVE('',#6876,#6879,#500,.T.);
#8944=EDGE_CURVE('',#6878,#6880,#4360,.T.);
#8945=EDGE_CURVE('',#6879,#6880,#4361,.T.);
#8946=EDGE_CURVE('',#6879,#6881,#501,.T.);
#8947=EDGE_CURVE('',#6880,#6882,#4362,.T.);
#8948=EDGE_CURVE('',#6881,#6882,#4363,.T.);
#8949=EDGE_CURVE('',#6881,#6883,#502,.T.);
#8950=EDGE_CURVE('',#6882,#6884,#4364,.T.);
#8951=EDGE_CURVE('',#6883,#6884,#4365,.T.);
#8952=EDGE_CURVE('',#6885,#6875,#503,.T.);
#8953=EDGE_CURVE('',#6885,#6886,#4366,.T.);
#8954=EDGE_CURVE('',#6886,#6877,#4367,.T.);
#8955=EDGE_CURVE('',#6883,#6885,#504,.T.);
#8956=EDGE_CURVE('',#6884,#6886,#4368,.T.);
#8957=EDGE_CURVE('',#6887,#6887,#1253,.T.);
#8958=EDGE_CURVE('',#6870,#6887,#4369,.T.);
#8959=EDGE_CURVE('',#6872,#6868,#1254,.T.);
#8960=EDGE_CURVE('',#6888,#6888,#1255,.T.);
#8961=EDGE_CURVE('',#6889,#6890,#1256,.T.);
#8962=EDGE_CURVE('',#6889,#6888,#4370,.T.);
#8963=EDGE_CURVE('',#6890,#6889,#1257,.T.);
#8964=EDGE_CURVE('',#6881,#6890,#3175,.T.);
#12629=ORIENTED_EDGE('',*,*,#8756,.F.);
#12630=ORIENTED_EDGE('',*,*,#8757,.T.);
#12631=ORIENTED_EDGE('',*,*,#8758,.T.);
#12632=ORIENTED_EDGE('',*,*,#8759,.T.);
#12633=ORIENTED_EDGE('',*,*,#8760,.F.);
#12634=ORIENTED_EDGE('',*,*,#8761,.T.);
#12635=ORIENTED_EDGE('',*,*,#8756,.T.);
#12636=ORIENTED_EDGE('',*,*,#8762,.T.);
#12637=ORIENTED_EDGE('',*,*,#8763,.F.);
#12638=ORIENTED_EDGE('',*,*,#8764,.T.);
#12639=ORIENTED_EDGE('',*,*,#8760,.T.);
#12640=ORIENTED_EDGE('',*,*,#8765,.T.);
#12641=ORIENTED_EDGE('',*,*,#8766,.F.);
#12642=ORIENTED_EDGE('',*,*,#8767,.T.);
#12643=ORIENTED_EDGE('',*,*,#8763,.T.);
#12644=ORIENTED_EDGE('',*,*,#8768,.T.);
#12645=ORIENTED_EDGE('',*,*,#8769,.F.);
#12646=ORIENTED_EDGE('',*,*,#8770,.T.);
#12647=ORIENTED_EDGE('',*,*,#8766,.T.);
#12648=ORIENTED_EDGE('',*,*,#8771,.T.);
#12649=ORIENTED_EDGE('',*,*,#8772,.F.);
#12650=ORIENTED_EDGE('',*,*,#8773,.T.);
#12651=ORIENTED_EDGE('',*,*,#8769,.T.);
#12652=ORIENTED_EDGE('',*,*,#8774,.T.);
#12653=ORIENTED_EDGE('',*,*,#8775,.F.);
#12654=ORIENTED_EDGE('',*,*,#8776,.T.);
#12655=ORIENTED_EDGE('',*,*,#8772,.T.);
#12656=ORIENTED_EDGE('',*,*,#8777,.T.);
#12657=ORIENTED_EDGE('',*,*,#8778,.F.);
#12658=ORIENTED_EDGE('',*,*,#8779,.T.);
#12659=ORIENTED_EDGE('',*,*,#8775,.T.);
#12660=ORIENTED_EDGE('',*,*,#8780,.T.);
#12661=ORIENTED_EDGE('',*,*,#8781,.F.);
#12662=ORIENTED_EDGE('',*,*,#8782,.T.);
#12663=ORIENTED_EDGE('',*,*,#8778,.T.);
#12664=ORIENTED_EDGE('',*,*,#8783,.T.);
#12665=ORIENTED_EDGE('',*,*,#8784,.F.);
#12666=ORIENTED_EDGE('',*,*,#8785,.T.);
#12667=ORIENTED_EDGE('',*,*,#8781,.T.);
#12668=ORIENTED_EDGE('',*,*,#8786,.T.);
#12669=ORIENTED_EDGE('',*,*,#8787,.F.);
#12670=ORIENTED_EDGE('',*,*,#8788,.T.);
#12671=ORIENTED_EDGE('',*,*,#8784,.T.);
#12672=ORIENTED_EDGE('',*,*,#8789,.T.);
#12673=ORIENTED_EDGE('',*,*,#8790,.F.);
#12674=ORIENTED_EDGE('',*,*,#8791,.T.);
#12675=ORIENTED_EDGE('',*,*,#8787,.T.);
#12676=ORIENTED_EDGE('',*,*,#8792,.T.);
#12677=ORIENTED_EDGE('',*,*,#8793,.F.);
#12678=ORIENTED_EDGE('',*,*,#8794,.T.);
#12679=ORIENTED_EDGE('',*,*,#8790,.T.);
#12680=ORIENTED_EDGE('',*,*,#8795,.T.);
#12681=ORIENTED_EDGE('',*,*,#8796,.F.);
#12682=ORIENTED_EDGE('',*,*,#8797,.T.);
#12683=ORIENTED_EDGE('',*,*,#8793,.T.);
#12684=ORIENTED_EDGE('',*,*,#8798,.T.);
#12685=ORIENTED_EDGE('',*,*,#8799,.F.);
#12686=ORIENTED_EDGE('',*,*,#8800,.T.);
#12687=ORIENTED_EDGE('',*,*,#8796,.T.);
#12688=ORIENTED_EDGE('',*,*,#8801,.T.);
#12689=ORIENTED_EDGE('',*,*,#8802,.F.);
#12690=ORIENTED_EDGE('',*,*,#8803,.T.);
#12691=ORIENTED_EDGE('',*,*,#8799,.T.);
#12692=ORIENTED_EDGE('',*,*,#8804,.T.);
#12693=ORIENTED_EDGE('',*,*,#8805,.F.);
#12694=ORIENTED_EDGE('',*,*,#8806,.T.);
#12695=ORIENTED_EDGE('',*,*,#8802,.T.);
#12696=ORIENTED_EDGE('',*,*,#8807,.T.);
#12697=ORIENTED_EDGE('',*,*,#8808,.F.);
#12698=ORIENTED_EDGE('',*,*,#8809,.T.);
#12699=ORIENTED_EDGE('',*,*,#8805,.T.);
#12700=ORIENTED_EDGE('',*,*,#8810,.T.);
#12701=ORIENTED_EDGE('',*,*,#8811,.F.);
#12702=ORIENTED_EDGE('',*,*,#8812,.T.);
#12703=ORIENTED_EDGE('',*,*,#8808,.T.);
#12704=ORIENTED_EDGE('',*,*,#8813,.T.);
#12705=ORIENTED_EDGE('',*,*,#8814,.F.);
#12706=ORIENTED_EDGE('',*,*,#8815,.T.);
#12707=ORIENTED_EDGE('',*,*,#8811,.T.);
#12708=ORIENTED_EDGE('',*,*,#8816,.T.);
#12709=ORIENTED_EDGE('',*,*,#8817,.F.);
#12710=ORIENTED_EDGE('',*,*,#8818,.T.);
#12711=ORIENTED_EDGE('',*,*,#8814,.T.);
#12712=ORIENTED_EDGE('',*,*,#8819,.T.);
#12713=ORIENTED_EDGE('',*,*,#8820,.F.);
#12714=ORIENTED_EDGE('',*,*,#8821,.T.);
#12715=ORIENTED_EDGE('',*,*,#8817,.T.);
#12716=ORIENTED_EDGE('',*,*,#8822,.T.);
#12717=ORIENTED_EDGE('',*,*,#8823,.F.);
#12718=ORIENTED_EDGE('',*,*,#8824,.T.);
#12719=ORIENTED_EDGE('',*,*,#8820,.T.);
#12720=ORIENTED_EDGE('',*,*,#8825,.T.);
#12721=ORIENTED_EDGE('',*,*,#8826,.F.);
#12722=ORIENTED_EDGE('',*,*,#8827,.T.);
#12723=ORIENTED_EDGE('',*,*,#8823,.T.);
#12724=ORIENTED_EDGE('',*,*,#8828,.T.);
#12725=ORIENTED_EDGE('',*,*,#8829,.F.);
#12726=ORIENTED_EDGE('',*,*,#8830,.T.);
#12727=ORIENTED_EDGE('',*,*,#8826,.T.);
#12728=ORIENTED_EDGE('',*,*,#8831,.T.);
#12729=ORIENTED_EDGE('',*,*,#8832,.F.);
#12730=ORIENTED_EDGE('',*,*,#8833,.T.);
#12731=ORIENTED_EDGE('',*,*,#8829,.T.);
#12732=ORIENTED_EDGE('',*,*,#8834,.T.);
#12733=ORIENTED_EDGE('',*,*,#8835,.F.);
#12734=ORIENTED_EDGE('',*,*,#8836,.T.);
#12735=ORIENTED_EDGE('',*,*,#8832,.T.);
#12736=ORIENTED_EDGE('',*,*,#8837,.T.);
#12737=ORIENTED_EDGE('',*,*,#8838,.F.);
#12738=ORIENTED_EDGE('',*,*,#8839,.T.);
#12739=ORIENTED_EDGE('',*,*,#8835,.T.);
#12740=ORIENTED_EDGE('',*,*,#8840,.T.);
#12741=ORIENTED_EDGE('',*,*,#8841,.F.);
#12742=ORIENTED_EDGE('',*,*,#8842,.T.);
#12743=ORIENTED_EDGE('',*,*,#8843,.F.);
#12744=ORIENTED_EDGE('',*,*,#8844,.F.);
#12745=ORIENTED_EDGE('',*,*,#8845,.F.);
#12746=ORIENTED_EDGE('',*,*,#8846,.T.);
#12747=ORIENTED_EDGE('',*,*,#8841,.T.);
#12748=ORIENTED_EDGE('',*,*,#8847,.F.);
#12749=ORIENTED_EDGE('',*,*,#8848,.F.);
#12750=ORIENTED_EDGE('',*,*,#8849,.T.);
#12751=ORIENTED_EDGE('',*,*,#8845,.T.);
#12752=ORIENTED_EDGE('',*,*,#8850,.F.);
#12753=ORIENTED_EDGE('',*,*,#8851,.F.);
#12754=ORIENTED_EDGE('',*,*,#8852,.T.);
#12755=ORIENTED_EDGE('',*,*,#8848,.T.);
#12756=ORIENTED_EDGE('',*,*,#8853,.F.);
#12757=ORIENTED_EDGE('',*,*,#8854,.F.);
#12758=ORIENTED_EDGE('',*,*,#8855,.T.);
#12759=ORIENTED_EDGE('',*,*,#8851,.T.);
#12760=ORIENTED_EDGE('',*,*,#8856,.F.);
#12761=ORIENTED_EDGE('',*,*,#8857,.F.);
#12762=ORIENTED_EDGE('',*,*,#8858,.T.);
#12763=ORIENTED_EDGE('',*,*,#8854,.T.);
#12764=ORIENTED_EDGE('',*,*,#8859,.F.);
#12765=ORIENTED_EDGE('',*,*,#8860,.F.);
#12766=ORIENTED_EDGE('',*,*,#8861,.T.);
#12767=ORIENTED_EDGE('',*,*,#8857,.T.);
#12768=ORIENTED_EDGE('',*,*,#8862,.F.);
#12769=ORIENTED_EDGE('',*,*,#8863,.F.);
#12770=ORIENTED_EDGE('',*,*,#8864,.T.);
#12771=ORIENTED_EDGE('',*,*,#8860,.T.);
#12772=ORIENTED_EDGE('',*,*,#8865,.F.);
#12773=ORIENTED_EDGE('',*,*,#8866,.F.);
#12774=ORIENTED_EDGE('',*,*,#8867,.T.);
#12775=ORIENTED_EDGE('',*,*,#8863,.T.);
#12776=ORIENTED_EDGE('',*,*,#8868,.F.);
#12777=ORIENTED_EDGE('',*,*,#8869,.F.);
#12778=ORIENTED_EDGE('',*,*,#8870,.T.);
#12779=ORIENTED_EDGE('',*,*,#8866,.T.);
#12780=ORIENTED_EDGE('',*,*,#8871,.F.);
#12781=ORIENTED_EDGE('',*,*,#8872,.F.);
#12782=ORIENTED_EDGE('',*,*,#8873,.T.);
#12783=ORIENTED_EDGE('',*,*,#8869,.T.);
#12784=ORIENTED_EDGE('',*,*,#8874,.F.);
#12785=ORIENTED_EDGE('',*,*,#8875,.F.);
#12786=ORIENTED_EDGE('',*,*,#8876,.T.);
#12787=ORIENTED_EDGE('',*,*,#8872,.T.);
#12788=ORIENTED_EDGE('',*,*,#8877,.F.);
#12789=ORIENTED_EDGE('',*,*,#8878,.F.);
#12790=ORIENTED_EDGE('',*,*,#8879,.T.);
#12791=ORIENTED_EDGE('',*,*,#8875,.T.);
#12792=ORIENTED_EDGE('',*,*,#8880,.F.);
#12793=ORIENTED_EDGE('',*,*,#8881,.F.);
#12794=ORIENTED_EDGE('',*,*,#8882,.T.);
#12795=ORIENTED_EDGE('',*,*,#8878,.T.);
#12796=ORIENTED_EDGE('',*,*,#8883,.F.);
#12797=ORIENTED_EDGE('',*,*,#8884,.F.);
#12798=ORIENTED_EDGE('',*,*,#8885,.T.);
#12799=ORIENTED_EDGE('',*,*,#8881,.T.);
#12800=ORIENTED_EDGE('',*,*,#8886,.F.);
#12801=ORIENTED_EDGE('',*,*,#8887,.F.);
#12802=ORIENTED_EDGE('',*,*,#8888,.T.);
#12803=ORIENTED_EDGE('',*,*,#8884,.T.);
#12804=ORIENTED_EDGE('',*,*,#8889,.F.);
#12805=ORIENTED_EDGE('',*,*,#8890,.F.);
#12806=ORIENTED_EDGE('',*,*,#8891,.T.);
#12807=ORIENTED_EDGE('',*,*,#8887,.T.);
#12808=ORIENTED_EDGE('',*,*,#8892,.F.);
#12809=ORIENTED_EDGE('',*,*,#8893,.F.);
#12810=ORIENTED_EDGE('',*,*,#8894,.T.);
#12811=ORIENTED_EDGE('',*,*,#8890,.T.);
#12812=ORIENTED_EDGE('',*,*,#8895,.F.);
#12813=ORIENTED_EDGE('',*,*,#8896,.F.);
#12814=ORIENTED_EDGE('',*,*,#8897,.T.);
#12815=ORIENTED_EDGE('',*,*,#8893,.T.);
#12816=ORIENTED_EDGE('',*,*,#8898,.F.);
#12817=ORIENTED_EDGE('',*,*,#8899,.F.);
#12818=ORIENTED_EDGE('',*,*,#8900,.T.);
#12819=ORIENTED_EDGE('',*,*,#8896,.T.);
#12820=ORIENTED_EDGE('',*,*,#8901,.F.);
#12821=ORIENTED_EDGE('',*,*,#8902,.F.);
#12822=ORIENTED_EDGE('',*,*,#8903,.T.);
#12823=ORIENTED_EDGE('',*,*,#8899,.T.);
#12824=ORIENTED_EDGE('',*,*,#8904,.F.);
#12825=ORIENTED_EDGE('',*,*,#8905,.F.);
#12826=ORIENTED_EDGE('',*,*,#8906,.T.);
#12827=ORIENTED_EDGE('',*,*,#8902,.T.);
#12828=ORIENTED_EDGE('',*,*,#8907,.F.);
#12829=ORIENTED_EDGE('',*,*,#8908,.F.);
#12830=ORIENTED_EDGE('',*,*,#8909,.T.);
#12831=ORIENTED_EDGE('',*,*,#8905,.T.);
#12832=ORIENTED_EDGE('',*,*,#8910,.F.);
#12833=ORIENTED_EDGE('',*,*,#8911,.F.);
#12834=ORIENTED_EDGE('',*,*,#8912,.T.);
#12835=ORIENTED_EDGE('',*,*,#8908,.T.);
#12836=ORIENTED_EDGE('',*,*,#8913,.F.);
#12837=ORIENTED_EDGE('',*,*,#8914,.F.);
#12838=ORIENTED_EDGE('',*,*,#8915,.T.);
#12839=ORIENTED_EDGE('',*,*,#8911,.T.);
#12840=ORIENTED_EDGE('',*,*,#8916,.F.);
#12841=ORIENTED_EDGE('',*,*,#8917,.F.);
#12842=ORIENTED_EDGE('',*,*,#8918,.T.);
#12843=ORIENTED_EDGE('',*,*,#8914,.T.);
#12844=ORIENTED_EDGE('',*,*,#8919,.F.);
#12845=ORIENTED_EDGE('',*,*,#8920,.F.);
#12846=ORIENTED_EDGE('',*,*,#8921,.T.);
#12847=ORIENTED_EDGE('',*,*,#8917,.T.);
#12848=ORIENTED_EDGE('',*,*,#8922,.F.);
#12849=ORIENTED_EDGE('',*,*,#8923,.F.);
#12850=ORIENTED_EDGE('',*,*,#8924,.T.);
#12851=ORIENTED_EDGE('',*,*,#8920,.T.);
#12852=ORIENTED_EDGE('',*,*,#8925,.F.);
#12853=ORIENTED_EDGE('',*,*,#8926,.F.);
#12854=ORIENTED_EDGE('',*,*,#8927,.F.);
#12855=ORIENTED_EDGE('',*,*,#8840,.F.);
#12856=ORIENTED_EDGE('',*,*,#8837,.F.);
#12857=ORIENTED_EDGE('',*,*,#8834,.F.);
#12858=ORIENTED_EDGE('',*,*,#8831,.F.);
#12859=ORIENTED_EDGE('',*,*,#8828,.F.);
#12860=ORIENTED_EDGE('',*,*,#8825,.F.);
#12861=ORIENTED_EDGE('',*,*,#8822,.F.);
#12862=ORIENTED_EDGE('',*,*,#8819,.F.);
#12863=ORIENTED_EDGE('',*,*,#8816,.F.);
#12864=ORIENTED_EDGE('',*,*,#8813,.F.);
#12865=ORIENTED_EDGE('',*,*,#8810,.F.);
#12866=ORIENTED_EDGE('',*,*,#8807,.F.);
#12867=ORIENTED_EDGE('',*,*,#8804,.F.);
#12868=ORIENTED_EDGE('',*,*,#8801,.F.);
#12869=ORIENTED_EDGE('',*,*,#8798,.F.);
#12870=ORIENTED_EDGE('',*,*,#8795,.F.);
#12871=ORIENTED_EDGE('',*,*,#8792,.F.);
#12872=ORIENTED_EDGE('',*,*,#8789,.F.);
#12873=ORIENTED_EDGE('',*,*,#8786,.F.);
#12874=ORIENTED_EDGE('',*,*,#8783,.F.);
#12875=ORIENTED_EDGE('',*,*,#8780,.F.);
#12876=ORIENTED_EDGE('',*,*,#8777,.F.);
#12877=ORIENTED_EDGE('',*,*,#8774,.F.);
#12878=ORIENTED_EDGE('',*,*,#8771,.F.);
#12879=ORIENTED_EDGE('',*,*,#8768,.F.);
#12880=ORIENTED_EDGE('',*,*,#8765,.F.);
#12881=ORIENTED_EDGE('',*,*,#8762,.F.);
#12882=ORIENTED_EDGE('',*,*,#8759,.F.);
#12883=ORIENTED_EDGE('',*,*,#8928,.F.);
#12884=ORIENTED_EDGE('',*,*,#8929,.T.);
#12885=ORIENTED_EDGE('',*,*,#8925,.T.);
#12886=ORIENTED_EDGE('',*,*,#8922,.T.);
#12887=ORIENTED_EDGE('',*,*,#8919,.T.);
#12888=ORIENTED_EDGE('',*,*,#8916,.T.);
#12889=ORIENTED_EDGE('',*,*,#8913,.T.);
#12890=ORIENTED_EDGE('',*,*,#8910,.T.);
#12891=ORIENTED_EDGE('',*,*,#8907,.T.);
#12892=ORIENTED_EDGE('',*,*,#8904,.T.);
#12893=ORIENTED_EDGE('',*,*,#8901,.T.);
#12894=ORIENTED_EDGE('',*,*,#8898,.T.);
#12895=ORIENTED_EDGE('',*,*,#8895,.T.);
#12896=ORIENTED_EDGE('',*,*,#8892,.T.);
#12897=ORIENTED_EDGE('',*,*,#8889,.T.);
#12898=ORIENTED_EDGE('',*,*,#8886,.T.);
#12899=ORIENTED_EDGE('',*,*,#8883,.T.);
#12900=ORIENTED_EDGE('',*,*,#8880,.T.);
#12901=ORIENTED_EDGE('',*,*,#8877,.T.);
#12902=ORIENTED_EDGE('',*,*,#8874,.T.);
#12903=ORIENTED_EDGE('',*,*,#8871,.T.);
#12904=ORIENTED_EDGE('',*,*,#8868,.T.);
#12905=ORIENTED_EDGE('',*,*,#8865,.T.);
#12906=ORIENTED_EDGE('',*,*,#8862,.T.);
#12907=ORIENTED_EDGE('',*,*,#8859,.T.);
#12908=ORIENTED_EDGE('',*,*,#8856,.T.);
#12909=ORIENTED_EDGE('',*,*,#8853,.T.);
#12910=ORIENTED_EDGE('',*,*,#8850,.T.);
#12911=ORIENTED_EDGE('',*,*,#8847,.T.);
#12912=ORIENTED_EDGE('',*,*,#8844,.T.);
#12913=ORIENTED_EDGE('',*,*,#8930,.T.);
#12914=ORIENTED_EDGE('',*,*,#8931,.T.);
#12915=ORIENTED_EDGE('',*,*,#8932,.T.);
#12916=ORIENTED_EDGE('',*,*,#8933,.T.);
#12917=ORIENTED_EDGE('',*,*,#8928,.T.);
#12918=ORIENTED_EDGE('',*,*,#8923,.T.);
#12919=ORIENTED_EDGE('',*,*,#8929,.F.);
#12920=ORIENTED_EDGE('',*,*,#8933,.F.);
#12921=ORIENTED_EDGE('',*,*,#8934,.T.);
#12922=ORIENTED_EDGE('',*,*,#8935,.F.);
#12923=ORIENTED_EDGE('',*,*,#8842,.F.);
#12924=ORIENTED_EDGE('',*,*,#8846,.F.);
#12925=ORIENTED_EDGE('',*,*,#8849,.F.);
#12926=ORIENTED_EDGE('',*,*,#8852,.F.);
#12927=ORIENTED_EDGE('',*,*,#8855,.F.);
#12928=ORIENTED_EDGE('',*,*,#8858,.F.);
#12929=ORIENTED_EDGE('',*,*,#8861,.F.);
#12930=ORIENTED_EDGE('',*,*,#8864,.F.);
#12931=ORIENTED_EDGE('',*,*,#8867,.F.);
#12932=ORIENTED_EDGE('',*,*,#8870,.F.);
#12933=ORIENTED_EDGE('',*,*,#8873,.F.);
#12934=ORIENTED_EDGE('',*,*,#8876,.F.);
#12935=ORIENTED_EDGE('',*,*,#8879,.F.);
#12936=ORIENTED_EDGE('',*,*,#8882,.F.);
#12937=ORIENTED_EDGE('',*,*,#8885,.F.);
#12938=ORIENTED_EDGE('',*,*,#8888,.F.);
#12939=ORIENTED_EDGE('',*,*,#8891,.F.);
#12940=ORIENTED_EDGE('',*,*,#8894,.F.);
#12941=ORIENTED_EDGE('',*,*,#8897,.F.);
#12942=ORIENTED_EDGE('',*,*,#8900,.F.);
#12943=ORIENTED_EDGE('',*,*,#8903,.F.);
#12944=ORIENTED_EDGE('',*,*,#8906,.F.);
#12945=ORIENTED_EDGE('',*,*,#8909,.F.);
#12946=ORIENTED_EDGE('',*,*,#8912,.F.);
#12947=ORIENTED_EDGE('',*,*,#8915,.F.);
#12948=ORIENTED_EDGE('',*,*,#8918,.F.);
#12949=ORIENTED_EDGE('',*,*,#8921,.F.);
#12950=ORIENTED_EDGE('',*,*,#8924,.F.);
#12951=ORIENTED_EDGE('',*,*,#8934,.F.);
#12952=ORIENTED_EDGE('',*,*,#8932,.F.);
#12953=ORIENTED_EDGE('',*,*,#8757,.F.);
#12954=ORIENTED_EDGE('',*,*,#8761,.F.);
#12955=ORIENTED_EDGE('',*,*,#8764,.F.);
#12956=ORIENTED_EDGE('',*,*,#8767,.F.);
#12957=ORIENTED_EDGE('',*,*,#8770,.F.);
#12958=ORIENTED_EDGE('',*,*,#8773,.F.);
#12959=ORIENTED_EDGE('',*,*,#8776,.F.);
#12960=ORIENTED_EDGE('',*,*,#8779,.F.);
#12961=ORIENTED_EDGE('',*,*,#8782,.F.);
#12962=ORIENTED_EDGE('',*,*,#8785,.F.);
#12963=ORIENTED_EDGE('',*,*,#8788,.F.);
#12964=ORIENTED_EDGE('',*,*,#8791,.F.);
#12965=ORIENTED_EDGE('',*,*,#8794,.F.);
#12966=ORIENTED_EDGE('',*,*,#8797,.F.);
#12967=ORIENTED_EDGE('',*,*,#8800,.F.);
#12968=ORIENTED_EDGE('',*,*,#8803,.F.);
#12969=ORIENTED_EDGE('',*,*,#8806,.F.);
#12970=ORIENTED_EDGE('',*,*,#8809,.F.);
#12971=ORIENTED_EDGE('',*,*,#8812,.F.);
#12972=ORIENTED_EDGE('',*,*,#8815,.F.);
#12973=ORIENTED_EDGE('',*,*,#8818,.F.);
#12974=ORIENTED_EDGE('',*,*,#8821,.F.);
#12975=ORIENTED_EDGE('',*,*,#8824,.F.);
#12976=ORIENTED_EDGE('',*,*,#8827,.F.);
#12977=ORIENTED_EDGE('',*,*,#8830,.F.);
#12978=ORIENTED_EDGE('',*,*,#8833,.F.);
#12979=ORIENTED_EDGE('',*,*,#8836,.F.);
#12980=ORIENTED_EDGE('',*,*,#8839,.F.);
#12981=ORIENTED_EDGE('',*,*,#8936,.F.);
#12982=ORIENTED_EDGE('',*,*,#8937,.T.);
#12983=ORIENTED_EDGE('',*,*,#8938,.F.);
#12984=ORIENTED_EDGE('',*,*,#8937,.F.);
#12985=ORIENTED_EDGE('',*,*,#8939,.F.);
#12986=ORIENTED_EDGE('',*,*,#8940,.T.);
#12987=ORIENTED_EDGE('',*,*,#8941,.T.);
#12988=ORIENTED_EDGE('',*,*,#8942,.F.);
#12989=ORIENTED_EDGE('',*,*,#8943,.F.);
#12990=ORIENTED_EDGE('',*,*,#8942,.T.);
#12991=ORIENTED_EDGE('',*,*,#8944,.T.);
#12992=ORIENTED_EDGE('',*,*,#8945,.F.);
#12993=ORIENTED_EDGE('',*,*,#8946,.F.);
#12994=ORIENTED_EDGE('',*,*,#8945,.T.);
#12995=ORIENTED_EDGE('',*,*,#8947,.T.);
#12996=ORIENTED_EDGE('',*,*,#8948,.F.);
#12997=ORIENTED_EDGE('',*,*,#8949,.F.);
#12998=ORIENTED_EDGE('',*,*,#8948,.T.);
#12999=ORIENTED_EDGE('',*,*,#8950,.T.);
#13000=ORIENTED_EDGE('',*,*,#8951,.F.);
#13001=ORIENTED_EDGE('',*,*,#8952,.F.);
#13002=ORIENTED_EDGE('',*,*,#8953,.T.);
#13003=ORIENTED_EDGE('',*,*,#8954,.T.);
#13004=ORIENTED_EDGE('',*,*,#8940,.F.);
#13005=ORIENTED_EDGE('',*,*,#8955,.F.);
#13006=ORIENTED_EDGE('',*,*,#8951,.T.);
#13007=ORIENTED_EDGE('',*,*,#8956,.T.);
#13008=ORIENTED_EDGE('',*,*,#8953,.F.);
#13009=ORIENTED_EDGE('',*,*,#8956,.F.);
#13010=ORIENTED_EDGE('',*,*,#8950,.F.);
#13011=ORIENTED_EDGE('',*,*,#8947,.F.);
#13012=ORIENTED_EDGE('',*,*,#8944,.F.);
#13013=ORIENTED_EDGE('',*,*,#8941,.F.);
#13014=ORIENTED_EDGE('',*,*,#8954,.F.);
#13015=ORIENTED_EDGE('',*,*,#8938,.T.);
#13016=ORIENTED_EDGE('',*,*,#8957,.F.);
#13017=ORIENTED_EDGE('',*,*,#8930,.F.);
#13018=ORIENTED_EDGE('',*,*,#8758,.F.);
#13019=ORIENTED_EDGE('',*,*,#8931,.F.);
#13020=ORIENTED_EDGE('',*,*,#8958,.T.);
#13021=ORIENTED_EDGE('',*,*,#8957,.T.);
#13022=ORIENTED_EDGE('',*,*,#8958,.F.);
#13023=ORIENTED_EDGE('',*,*,#8838,.T.);
#13024=ORIENTED_EDGE('',*,*,#8927,.T.);
#13025=ORIENTED_EDGE('',*,*,#8959,.F.);
#13026=ORIENTED_EDGE('',*,*,#8936,.T.);
#13027=ORIENTED_EDGE('',*,*,#8960,.F.);
#13028=ORIENTED_EDGE('',*,*,#8959,.T.);
#13029=ORIENTED_EDGE('',*,*,#8926,.T.);
#13030=ORIENTED_EDGE('',*,*,#8843,.T.);
#13031=ORIENTED_EDGE('',*,*,#8935,.T.);
#13032=ORIENTED_EDGE('',*,*,#8961,.F.);
#13033=ORIENTED_EDGE('',*,*,#8962,.T.);
#13034=ORIENTED_EDGE('',*,*,#8960,.T.);
#13035=ORIENTED_EDGE('',*,*,#8962,.F.);
#13036=ORIENTED_EDGE('',*,*,#8963,.F.);
#13037=ORIENTED_EDGE('',*,*,#8949,.T.);
#13038=ORIENTED_EDGE('',*,*,#8955,.T.);
#13039=ORIENTED_EDGE('',*,*,#8952,.T.);
#13040=ORIENTED_EDGE('',*,*,#8939,.T.);
#13041=ORIENTED_EDGE('',*,*,#8943,.T.);
#13042=ORIENTED_EDGE('',*,*,#8946,.T.);
#13043=ORIENTED_EDGE('',*,*,#8964,.T.);
#13044=ORIENTED_EDGE('',*,*,#8963,.T.);
#13045=ORIENTED_EDGE('',*,*,#8961,.T.);
#13046=ORIENTED_EDGE('',*,*,#8964,.F.);
#13900=PLANE('',#15975);
#13901=PLANE('',#15982);
#13902=PLANE('',#15983);
#13903=PLANE('',#15984);
#13904=PLANE('',#15985);
#13905=PLANE('',#15986);
#13906=PLANE('',#15987);
#13907=PLANE('',#15988);
#13908=PLANE('',#15989);
#13909=PLANE('',#15994);
#14624=ADVANCED_FACE('',(#2056),#851,.T.);
#14625=ADVANCED_FACE('',(#2057),#852,.T.);
#14626=ADVANCED_FACE('',(#2058),#853,.T.);
#14627=ADVANCED_FACE('',(#2059),#854,.T.);
#14628=ADVANCED_FACE('',(#2060),#855,.T.);
#14629=ADVANCED_FACE('',(#2061),#856,.T.);
#14630=ADVANCED_FACE('',(#2062),#857,.T.);
#14631=ADVANCED_FACE('',(#2063),#858,.T.);
#14632=ADVANCED_FACE('',(#2064),#859,.T.);
#14633=ADVANCED_FACE('',(#2065),#860,.T.);
#14634=ADVANCED_FACE('',(#2066),#861,.T.);
#14635=ADVANCED_FACE('',(#2067),#862,.T.);
#14636=ADVANCED_FACE('',(#2068),#863,.T.);
#14637=ADVANCED_FACE('',(#2069),#864,.T.);
#14638=ADVANCED_FACE('',(#2070),#865,.T.);
#14639=ADVANCED_FACE('',(#2071),#866,.T.);
#14640=ADVANCED_FACE('',(#2072),#867,.T.);
#14641=ADVANCED_FACE('',(#2073),#868,.T.);
#14642=ADVANCED_FACE('',(#2074),#869,.T.);
#14643=ADVANCED_FACE('',(#2075),#870,.T.);
#14644=ADVANCED_FACE('',(#2076),#871,.T.);
#14645=ADVANCED_FACE('',(#2077),#872,.T.);
#14646=ADVANCED_FACE('',(#2078),#873,.T.);
#14647=ADVANCED_FACE('',(#2079),#874,.T.);
#14648=ADVANCED_FACE('',(#2080),#875,.T.);
#14649=ADVANCED_FACE('',(#2081),#876,.T.);
#14650=ADVANCED_FACE('',(#2082),#877,.T.);
#14651=ADVANCED_FACE('',(#2083),#878,.T.);
#14652=ADVANCED_FACE('',(#2084),#879,.T.);
#14653=ADVANCED_FACE('',(#2085),#880,.T.);
#14654=ADVANCED_FACE('',(#2086),#881,.T.);
#14655=ADVANCED_FACE('',(#2087),#882,.T.);
#14656=ADVANCED_FACE('',(#2088),#883,.T.);
#14657=ADVANCED_FACE('',(#2089),#884,.T.);
#14658=ADVANCED_FACE('',(#2090),#885,.T.);
#14659=ADVANCED_FACE('',(#2091),#886,.T.);
#14660=ADVANCED_FACE('',(#2092),#887,.T.);
#14661=ADVANCED_FACE('',(#2093),#888,.T.);
#14662=ADVANCED_FACE('',(#2094),#889,.T.);
#14663=ADVANCED_FACE('',(#2095),#890,.T.);
#14664=ADVANCED_FACE('',(#2096),#891,.T.);
#14665=ADVANCED_FACE('',(#2097),#892,.T.);
#14666=ADVANCED_FACE('',(#2098),#893,.T.);
#14667=ADVANCED_FACE('',(#2099),#894,.T.);
#14668=ADVANCED_FACE('',(#2100),#895,.T.);
#14669=ADVANCED_FACE('',(#2101),#896,.T.);
#14670=ADVANCED_FACE('',(#2102),#897,.T.);
#14671=ADVANCED_FACE('',(#2103),#898,.T.);
#14672=ADVANCED_FACE('',(#2104),#899,.T.);
#14673=ADVANCED_FACE('',(#2105),#900,.T.);
#14674=ADVANCED_FACE('',(#2106),#901,.T.);
#14675=ADVANCED_FACE('',(#2107),#902,.T.);
#14676=ADVANCED_FACE('',(#2108),#903,.T.);
#14677=ADVANCED_FACE('',(#2109),#904,.T.);
#14678=ADVANCED_FACE('',(#2110),#905,.T.);
#14679=ADVANCED_FACE('',(#2111),#906,.T.);
#14680=ADVANCED_FACE('',(#2112),#116,.F.);
#14681=ADVANCED_FACE('',(#2113),#13900,.T.);
#14682=ADVANCED_FACE('',(#2114),#907,.T.);
#14683=ADVANCED_FACE('',(#2115),#117,.F.);
#14684=ADVANCED_FACE('',(#2116),#1358,.F.);
#14685=ADVANCED_FACE('',(#2117),#13901,.F.);
#14686=ADVANCED_FACE('',(#2118),#13902,.F.);
#14687=ADVANCED_FACE('',(#2119),#13903,.F.);
#14688=ADVANCED_FACE('',(#2120),#13904,.F.);
#14689=ADVANCED_FACE('',(#2121),#13905,.F.);
#14690=ADVANCED_FACE('',(#2122),#13906,.F.);
#14691=ADVANCED_FACE('',(#2123,#682),#13907,.F.);
#14692=ADVANCED_FACE('',(#2124),#13908,.T.);
#14693=ADVANCED_FACE('',(#2125),#1359,.T.);
#14694=ADVANCED_FACE('',(#2126),#908,.T.);
#14695=ADVANCED_FACE('',(#2127,#683),#13909,.T.);
#14696=ADVANCED_FACE('',(#2128),#909,.T.);
#14697=ADVANCED_FACE('',(#2129),#103,.F.);
#14785=CLOSED_SHELL('',(#14624,#14625,#14626,#14627,#14628,#14629,#14630,
#14631,#14632,#14633,#14634,#14635,#14636,#14637,#14638,#14639,#14640,#14641,
#14642,#14643,#14644,#14645,#14646,#14647,#14648,#14649,#14650,#14651,#14652,
#14653,#14654,#14655,#14656,#14657,#14658,#14659,#14660,#14661,#14662,#14663,
#14664,#14665,#14666,#14667,#14668,#14669,#14670,#14671,#14672,#14673,#14674,
#14675,#14676,#14677,#14678,#14679,#14680,#14681,#14682,#14683,#14684,#14685,
#14686,#14687,#14688,#14689,#14690,#14691,#14692,#14693,#14694,#14695,#14696,
#14697));
#15916=AXIS2_PLACEMENT_3D('',#30246,#19188,#19189);
#15917=AXIS2_PLACEMENT_3D('',#30247,#19190,#19191);
#15918=AXIS2_PLACEMENT_3D('',#30263,#19193,#19194);
#15919=AXIS2_PLACEMENT_3D('',#30271,#19195,#19196);
#15920=AXIS2_PLACEMENT_3D('',#30319,#19198,#19199);
#15921=AXIS2_PLACEMENT_3D('',#30367,#19201,#19202);
#15922=AXIS2_PLACEMENT_3D('',#30421,#19204,#19205);
#15923=AXIS2_PLACEMENT_3D('',#30469,#19207,#19208);
#15924=AXIS2_PLACEMENT_3D('',#30517,#19210,#19211);
#15925=AXIS2_PLACEMENT_3D('',#30565,#19213,#19214);
#15926=AXIS2_PLACEMENT_3D('',#30619,#19216,#19217);
#15927=AXIS2_PLACEMENT_3D('',#30667,#19219,#19220);
#15928=AXIS2_PLACEMENT_3D('',#30715,#19222,#19223);
#15929=AXIS2_PLACEMENT_3D('',#30769,#19225,#19226);
#15930=AXIS2_PLACEMENT_3D('',#30817,#19228,#19229);
#15931=AXIS2_PLACEMENT_3D('',#30865,#19231,#19232);
#15932=AXIS2_PLACEMENT_3D('',#30919,#19234,#19235);
#15933=AXIS2_PLACEMENT_3D('',#30967,#19237,#19238);
#15934=AXIS2_PLACEMENT_3D('',#31015,#19240,#19241);
#15935=AXIS2_PLACEMENT_3D('',#31063,#19243,#19244);
#15936=AXIS2_PLACEMENT_3D('',#31117,#19246,#19247);
#15937=AXIS2_PLACEMENT_3D('',#31165,#19249,#19250);
#15938=AXIS2_PLACEMENT_3D('',#31213,#19252,#19253);
#15939=AXIS2_PLACEMENT_3D('',#31267,#19255,#19256);
#15940=AXIS2_PLACEMENT_3D('',#31315,#19258,#19259);
#15941=AXIS2_PLACEMENT_3D('',#31363,#19261,#19262);
#15942=AXIS2_PLACEMENT_3D('',#31417,#19264,#19265);
#15943=AXIS2_PLACEMENT_3D('',#31465,#19267,#19268);
#15944=AXIS2_PLACEMENT_3D('',#31513,#19270,#19271);
#15945=AXIS2_PLACEMENT_3D('',#31567,#19273,#19274);
#15946=AXIS2_PLACEMENT_3D('',#31615,#19276,#19277);
#15947=AXIS2_PLACEMENT_3D('',#31627,#19279,#19280);
#15948=AXIS2_PLACEMENT_3D('',#31633,#19281,#19282);
#15949=AXIS2_PLACEMENT_3D('',#31657,#19284,#19285);
#15950=AXIS2_PLACEMENT_3D('',#31682,#19287,#19288);
#15951=AXIS2_PLACEMENT_3D('',#31707,#19290,#19291);
#15952=AXIS2_PLACEMENT_3D('',#31731,#19293,#19294);
#15953=AXIS2_PLACEMENT_3D('',#31756,#19296,#19297);
#15954=AXIS2_PLACEMENT_3D('',#31781,#19299,#19300);
#15955=AXIS2_PLACEMENT_3D('',#31805,#19302,#19303);
#15956=AXIS2_PLACEMENT_3D('',#31830,#19305,#19306);
#15957=AXIS2_PLACEMENT_3D('',#31855,#19308,#19309);
#15958=AXIS2_PLACEMENT_3D('',#31879,#19311,#19312);
#15959=AXIS2_PLACEMENT_3D('',#31904,#19314,#19315);
#15960=AXIS2_PLACEMENT_3D('',#31929,#19317,#19318);
#15961=AXIS2_PLACEMENT_3D('',#31953,#19320,#19321);
#15962=AXIS2_PLACEMENT_3D('',#31977,#19323,#19324);
#15963=AXIS2_PLACEMENT_3D('',#32002,#19326,#19327);
#15964=AXIS2_PLACEMENT_3D('',#32027,#19329,#19330);
#15965=AXIS2_PLACEMENT_3D('',#32051,#19332,#19333);
#15966=AXIS2_PLACEMENT_3D('',#32076,#19335,#19336);
#15967=AXIS2_PLACEMENT_3D('',#32101,#19338,#19339);
#15968=AXIS2_PLACEMENT_3D('',#32125,#19341,#19342);
#15969=AXIS2_PLACEMENT_3D('',#32150,#19344,#19345);
#15970=AXIS2_PLACEMENT_3D('',#32175,#19347,#19348);
#15971=AXIS2_PLACEMENT_3D('',#32199,#19350,#19351);
#15972=AXIS2_PLACEMENT_3D('',#32223,#19353,#19354);
#15973=AXIS2_PLACEMENT_3D('',#32248,#19356,#19357);
#15974=AXIS2_PLACEMENT_3D('',#32273,#19359,#19360);
#15975=AXIS2_PLACEMENT_3D('',#33228,#19362,#19363);
#15976=AXIS2_PLACEMENT_3D('',#33230,#19364,#19365);
#15977=AXIS2_PLACEMENT_3D('',#33231,#19366,#19367);
#15978=AXIS2_PLACEMENT_3D('',#33318,#19368,#19369);
#15979=AXIS2_PLACEMENT_3D('',#33319,#19370,#19371);
#15980=AXIS2_PLACEMENT_3D('',#34161,#19372,#19373);
#15981=AXIS2_PLACEMENT_3D('',#34165,#19375,#19376);
#15982=AXIS2_PLACEMENT_3D('',#34166,#19377,#19378);
#15983=AXIS2_PLACEMENT_3D('',#34180,#19382,#19383);
#15984=AXIS2_PLACEMENT_3D('',#34191,#19386,#19387);
#15985=AXIS2_PLACEMENT_3D('',#34202,#19390,#19391);
#15986=AXIS2_PLACEMENT_3D('',#34213,#19394,#19395);
#15987=AXIS2_PLACEMENT_3D('',#34224,#19398,#19399);
#15988=AXIS2_PLACEMENT_3D('',#34232,#19401,#19402);
#15989=AXIS2_PLACEMENT_3D('',#34233,#19403,#19404);
#15990=AXIS2_PLACEMENT_3D('',#34235,#19405,#19406);
#15991=AXIS2_PLACEMENT_3D('',#34236,#19407,#19408);
#15992=AXIS2_PLACEMENT_3D('',#34238,#19410,#19411);
#15993=AXIS2_PLACEMENT_3D('',#34239,#19412,#19413);
#15994=AXIS2_PLACEMENT_3D('',#34240,#19414,#19415);
#15995=AXIS2_PLACEMENT_3D('',#34242,#19416,#19417);
#15996=AXIS2_PLACEMENT_3D('',#34243,#19418,#19419);
#15997=AXIS2_PLACEMENT_3D('',#34246,#19420,#19421);
#15998=AXIS2_PLACEMENT_3D('',#34248,#19423,#19424);
#19188=DIRECTION('axis',(0.,0.,1.));
#19189=DIRECTION('refdir',(1.,0.,0.));
#19190=DIRECTION('center_axis',(1.,0.,0.));
#19191=DIRECTION('ref_axis',(0.,1.,0.));
#19192=DIRECTION('',(-1.,0.,0.));
#19193=DIRECTION('center_axis',(1.,0.,0.));
#19194=DIRECTION('ref_axis',(0.,1.,0.));
#19195=DIRECTION('center_axis',(1.,0.,0.));
#19196=DIRECTION('ref_axis',(0.,1.,0.));
#19197=DIRECTION('',(-1.,0.,0.));
#19198=DIRECTION('center_axis',(1.,0.,0.));
#19199=DIRECTION('ref_axis',(0.,1.,0.));
#19200=DIRECTION('',(-1.,0.,0.));
#19201=DIRECTION('center_axis',(1.,0.,0.));
#19202=DIRECTION('ref_axis',(0.,1.,0.));
#19203=DIRECTION('',(-1.,0.,0.));
#19204=DIRECTION('center_axis',(1.,0.,0.));
#19205=DIRECTION('ref_axis',(0.,1.,0.));
#19206=DIRECTION('',(-1.,0.,0.));
#19207=DIRECTION('center_axis',(1.,0.,0.));
#19208=DIRECTION('ref_axis',(0.,1.,0.));
#19209=DIRECTION('',(-1.,0.,0.));
#19210=DIRECTION('center_axis',(1.,0.,0.));
#19211=DIRECTION('ref_axis',(0.,1.,0.));
#19212=DIRECTION('',(-1.,0.,0.));
#19213=DIRECTION('center_axis',(1.,0.,0.));
#19214=DIRECTION('ref_axis',(0.,1.,0.));
#19215=DIRECTION('',(-1.,0.,0.));
#19216=DIRECTION('center_axis',(1.,0.,0.));
#19217=DIRECTION('ref_axis',(0.,1.,0.));
#19218=DIRECTION('',(-1.,0.,0.));
#19219=DIRECTION('center_axis',(1.,0.,0.));
#19220=DIRECTION('ref_axis',(0.,1.,0.));
#19221=DIRECTION('',(-1.,0.,0.));
#19222=DIRECTION('center_axis',(1.,0.,0.));
#19223=DIRECTION('ref_axis',(0.,1.,0.));
#19224=DIRECTION('',(-1.,0.,0.));
#19225=DIRECTION('center_axis',(1.,0.,0.));
#19226=DIRECTION('ref_axis',(0.,1.,0.));
#19227=DIRECTION('',(-1.,0.,0.));
#19228=DIRECTION('center_axis',(1.,0.,0.));
#19229=DIRECTION('ref_axis',(0.,1.,0.));
#19230=DIRECTION('',(-1.,0.,0.));
#19231=DIRECTION('center_axis',(1.,0.,0.));
#19232=DIRECTION('ref_axis',(0.,1.,0.));
#19233=DIRECTION('',(-1.,0.,0.));
#19234=DIRECTION('center_axis',(1.,0.,0.));
#19235=DIRECTION('ref_axis',(0.,1.,0.));
#19236=DIRECTION('',(-1.,0.,0.));
#19237=DIRECTION('center_axis',(1.,0.,0.));
#19238=DIRECTION('ref_axis',(0.,1.,0.));
#19239=DIRECTION('',(-1.,0.,0.));
#19240=DIRECTION('center_axis',(1.,0.,0.));
#19241=DIRECTION('ref_axis',(0.,1.,0.));
#19242=DIRECTION('',(-1.,0.,0.));
#19243=DIRECTION('center_axis',(1.,0.,0.));
#19244=DIRECTION('ref_axis',(0.,1.,0.));
#19245=DIRECTION('',(-1.,0.,0.));
#19246=DIRECTION('center_axis',(1.,0.,0.));
#19247=DIRECTION('ref_axis',(0.,1.,0.));
#19248=DIRECTION('',(-1.,0.,0.));
#19249=DIRECTION('center_axis',(1.,0.,0.));
#19250=DIRECTION('ref_axis',(0.,1.,0.));
#19251=DIRECTION('',(-1.,0.,0.));
#19252=DIRECTION('center_axis',(1.,0.,0.));
#19253=DIRECTION('ref_axis',(0.,1.,0.));
#19254=DIRECTION('',(-1.,0.,0.));
#19255=DIRECTION('center_axis',(1.,0.,0.));
#19256=DIRECTION('ref_axis',(0.,1.,0.));
#19257=DIRECTION('',(-1.,0.,0.));
#19258=DIRECTION('center_axis',(1.,0.,0.));
#19259=DIRECTION('ref_axis',(0.,1.,0.));
#19260=DIRECTION('',(-1.,0.,0.));
#19261=DIRECTION('center_axis',(1.,0.,0.));
#19262=DIRECTION('ref_axis',(0.,1.,0.));
#19263=DIRECTION('',(-1.,0.,0.));
#19264=DIRECTION('center_axis',(1.,0.,0.));
#19265=DIRECTION('ref_axis',(0.,1.,0.));
#19266=DIRECTION('',(-1.,0.,0.));
#19267=DIRECTION('center_axis',(1.,0.,0.));
#19268=DIRECTION('ref_axis',(0.,1.,0.));
#19269=DIRECTION('',(-1.,0.,0.));
#19270=DIRECTION('center_axis',(1.,0.,0.));
#19271=DIRECTION('ref_axis',(0.,1.,0.));
#19272=DIRECTION('',(-1.,0.,0.));
#19273=DIRECTION('center_axis',(1.,0.,0.));
#19274=DIRECTION('ref_axis',(0.,1.,0.));
#19275=DIRECTION('',(-1.,0.,0.));
#19276=DIRECTION('center_axis',(1.,0.,0.));
#19277=DIRECTION('ref_axis',(0.,-0.266010182744204,-0.963970218770474));
#19278=DIRECTION('',(1.,0.,0.));
#19279=DIRECTION('center_axis',(1.,0.,0.));
#19280=DIRECTION('ref_axis',(0.,1.,-1.17958518182489E-13));
#19281=DIRECTION('center_axis',(1.,0.,0.));
#19282=DIRECTION('ref_axis',(0.,1.,-1.17958518182489E-13));
#19283=DIRECTION('',(1.,0.,0.));
#19284=DIRECTION('center_axis',(1.,0.,0.));
#19285=DIRECTION('ref_axis',(0.,1.,-1.17958518182489E-13));
#19286=DIRECTION('',(1.,0.,0.));
#19287=DIRECTION('center_axis',(1.,0.,0.));
#19288=DIRECTION('ref_axis',(0.,1.,-1.17958518182489E-13));
#19289=DIRECTION('',(1.,0.,0.));
#19290=DIRECTION('center_axis',(1.,0.,0.));
#19291=DIRECTION('ref_axis',(0.,1.,-1.17958518182489E-13));
#19292=DIRECTION('',(1.,0.,0.));
#19293=DIRECTION('center_axis',(1.,0.,0.));
#19294=DIRECTION('ref_axis',(0.,1.,-1.17958518182489E-13));
#19295=DIRECTION('',(1.,0.,0.));
#19296=DIRECTION('center_axis',(1.,0.,0.));
#19297=DIRECTION('ref_axis',(0.,1.,-1.17958518182489E-13));
#19298=DIRECTION('',(1.,0.,0.));
#19299=DIRECTION('center_axis',(1.,0.,0.));
#19300=DIRECTION('ref_axis',(0.,1.,-1.17958518182489E-13));
#19301=DIRECTION('',(1.,0.,0.));
#19302=DIRECTION('center_axis',(1.,0.,0.));
#19303=DIRECTION('ref_axis',(0.,1.,-1.17958518182489E-13));
#19304=DIRECTION('',(1.,0.,0.));
#19305=DIRECTION('center_axis',(1.,0.,0.));
#19306=DIRECTION('ref_axis',(0.,1.,-1.17958518182489E-13));
#19307=DIRECTION('',(1.,0.,0.));
#19308=DIRECTION('center_axis',(1.,0.,0.));
#19309=DIRECTION('ref_axis',(0.,1.,-1.17958518182489E-13));
#19310=DIRECTION('',(1.,0.,0.));
#19311=DIRECTION('center_axis',(1.,0.,0.));
#19312=DIRECTION('ref_axis',(0.,1.,-1.17958518182489E-13));
#19313=DIRECTION('',(1.,0.,0.));
#19314=DIRECTION('center_axis',(1.,0.,0.));
#19315=DIRECTION('ref_axis',(0.,1.,-1.17958518182489E-13));
#19316=DIRECTION('',(1.,0.,0.));
#19317=DIRECTION('center_axis',(1.,0.,0.));
#19318=DIRECTION('ref_axis',(0.,1.,-1.17958518182489E-13));
#19319=DIRECTION('',(1.,0.,0.));
#19320=DIRECTION('center_axis',(1.,0.,0.));
#19321=DIRECTION('ref_axis',(0.,1.,-1.17958518182489E-13));
#19322=DIRECTION('',(1.,0.,0.));
#19323=DIRECTION('center_axis',(1.,0.,0.));
#19324=DIRECTION('ref_axis',(0.,1.,-1.17958518182489E-13));
#19325=DIRECTION('',(1.,0.,0.));
#19326=DIRECTION('center_axis',(1.,0.,0.));
#19327=DIRECTION('ref_axis',(0.,1.,-1.17958518182489E-13));
#19328=DIRECTION('',(1.,0.,0.));
#19329=DIRECTION('center_axis',(1.,0.,0.));
#19330=DIRECTION('ref_axis',(0.,1.,-1.17958518182489E-13));
#19331=DIRECTION('',(1.,0.,0.));
#19332=DIRECTION('center_axis',(1.,0.,0.));
#19333=DIRECTION('ref_axis',(0.,1.,-1.17958518182489E-13));
#19334=DIRECTION('',(1.,0.,0.));
#19335=DIRECTION('center_axis',(1.,0.,0.));
#19336=DIRECTION('ref_axis',(0.,1.,-1.17958518182489E-13));
#19337=DIRECTION('',(1.,0.,0.));
#19338=DIRECTION('center_axis',(1.,0.,0.));
#19339=DIRECTION('ref_axis',(0.,1.,-1.17958518182489E-13));
#19340=DIRECTION('',(1.,0.,0.));
#19341=DIRECTION('center_axis',(1.,0.,0.));
#19342=DIRECTION('ref_axis',(0.,1.,-1.17958518182489E-13));
#19343=DIRECTION('',(1.,0.,0.));
#19344=DIRECTION('center_axis',(1.,0.,0.));
#19345=DIRECTION('ref_axis',(0.,1.,-1.17958518182489E-13));
#19346=DIRECTION('',(1.,0.,0.));
#19347=DIRECTION('center_axis',(1.,0.,0.));
#19348=DIRECTION('ref_axis',(0.,1.,-1.17958518182489E-13));
#19349=DIRECTION('',(1.,0.,0.));
#19350=DIRECTION('center_axis',(1.,0.,0.));
#19351=DIRECTION('ref_axis',(0.,1.,-1.17958518182489E-13));
#19352=DIRECTION('',(1.,0.,0.));
#19353=DIRECTION('center_axis',(1.,0.,0.));
#19354=DIRECTION('ref_axis',(0.,1.,-1.17958518182489E-13));
#19355=DIRECTION('',(1.,0.,0.));
#19356=DIRECTION('center_axis',(1.,0.,0.));
#19357=DIRECTION('ref_axis',(0.,1.,-1.17958518182489E-13));
#19358=DIRECTION('',(1.,0.,0.));
#19359=DIRECTION('center_axis',(1.,0.,0.));
#19360=DIRECTION('ref_axis',(0.,1.,-1.17958518182489E-13));
#19361=DIRECTION('',(1.,0.,0.));
#19362=DIRECTION('center_axis',(1.,0.,0.));
#19363=DIRECTION('ref_axis',(0.,0.,-1.));
#19364=DIRECTION('center_axis',(1.,0.,0.));
#19365=DIRECTION('ref_axis',(0.,1.,0.));
#19366=DIRECTION('center_axis',(1.,0.,0.));
#19367=DIRECTION('ref_axis',(0.,1.,0.));
#19368=DIRECTION('center_axis',(-1.,0.,0.));
#19369=DIRECTION('ref_axis',(0.,1.,-1.17958518182489E-13));
#19370=DIRECTION('center_axis',(1.,0.,0.));
#19371=DIRECTION('ref_axis',(0.,1.,-1.17958518182489E-13));
#19372=DIRECTION('center_axis',(1.,0.,0.));
#19373=DIRECTION('ref_axis',(0.,1.,0.));
#19374=DIRECTION('',(0.520049754552021,-0.854135968561436,-1.04601487993539E-16));
#19375=DIRECTION('center_axis',(-1.,0.,0.));
#19376=DIRECTION('ref_axis',(0.,1.,0.));
#19377=DIRECTION('center_axis',(0.,-0.5,-0.866025403784439));
#19378=DIRECTION('ref_axis',(0.,-0.866025403784439,0.5));
#19379=DIRECTION('',(-1.,0.,0.));
#19380=DIRECTION('',(0.,-0.866025403784439,0.5));
#19381=DIRECTION('',(-1.,0.,0.));
#19382=DIRECTION('center_axis',(0.,-1.,-1.92296268638356E-16));
#19383=DIRECTION('ref_axis',(0.,-1.92296268638356E-16,1.));
#19384=DIRECTION('',(0.,-1.92296268638356E-16,1.));
#19385=DIRECTION('',(-1.,0.,0.));
#19386=DIRECTION('center_axis',(0.,-0.5,0.866025403784439));
#19387=DIRECTION('ref_axis',(0.,0.866025403784439,0.5));
#19388=DIRECTION('',(0.,0.866025403784439,0.5));
#19389=DIRECTION('',(-1.,0.,0.));
#19390=DIRECTION('center_axis',(0.,0.5,0.866025403784439));
#19391=DIRECTION('ref_axis',(0.,0.866025403784439,-0.5));
#19392=DIRECTION('',(0.,0.866025403784439,-0.5));
#19393=DIRECTION('',(-1.,0.,0.));
#19394=DIRECTION('center_axis',(0.,0.5,-0.866025403784439));
#19395=DIRECTION('ref_axis',(0.,-0.866025403784439,-0.5));
#19396=DIRECTION('',(-1.,0.,0.));
#19397=DIRECTION('',(0.,-0.866025403784439,-0.5));
#19398=DIRECTION('center_axis',(0.,1.,-3.84592537276713E-16));
#19399=DIRECTION('ref_axis',(0.,-3.84592537276713E-16,-1.));
#19400=DIRECTION('',(0.,-3.84592537276713E-16,-1.));
#19401=DIRECTION('center_axis',(-1.,0.,0.));
#19402=DIRECTION('ref_axis',(0.,0.,1.));
#19403=DIRECTION('center_axis',(-1.,0.,0.));
#19404=DIRECTION('ref_axis',(0.,0.,1.));
#19405=DIRECTION('center_axis',(1.,0.,0.));
#19406=DIRECTION('ref_axis',(0.,0.,-1.));
#19407=DIRECTION('center_axis',(1.,0.,0.));
#19408=DIRECTION('ref_axis',(0.,1.,0.));
#19409=DIRECTION('',(-0.707106781186546,0.707106781186549,8.65956056235496E-17));
#19410=DIRECTION('center_axis',(1.,0.,0.));
#19411=DIRECTION('ref_axis',(0.,0.93907309915965,-0.343717492186083));
#19412=DIRECTION('center_axis',(1.,0.,0.));
#19413=DIRECTION('ref_axis',(0.,1.,0.));
#19414=DIRECTION('center_axis',(-1.,0.,0.));
#19415=DIRECTION('ref_axis',(0.,0.,1.));
#19416=DIRECTION('center_axis',(1.,0.,0.));
#19417=DIRECTION('ref_axis',(0.,0.,-1.));
#19418=DIRECTION('center_axis',(1.,0.,0.));
#19419=DIRECTION('ref_axis',(0.,1.,0.));
#19420=DIRECTION('center_axis',(1.,0.,0.));
#19421=DIRECTION('ref_axis',(0.,0.,-1.));
#19422=DIRECTION('',(-1.,0.,0.));
#19423=DIRECTION('center_axis',(1.,0.,0.));
#19424=DIRECTION('ref_axis',(0.,0.,-1.));
#30246=CARTESIAN_POINT('',(0.,0.,0.));
#30247=CARTESIAN_POINT('Origin',(-9.8,0.,0.));
#30248=CARTESIAN_POINT('',(-19.4201303078758,-1.95628952807724,0.00129327600707104));
#30249=CARTESIAN_POINT('',(-19.5218696921242,-1.95584467742209,0.00207536885323489));
#30250=CARTESIAN_POINT('',(-9.8,-1.954,-2.39295984553393E-16));
#30251=CARTESIAN_POINT('',(-19.646,0.862546313953447,1.75510541481596));
#30252=CARTESIAN_POINT('Ctrl Pts',(-19.4201303078758,-1.95628952807724,
0.00129327600707104));
#30253=CARTESIAN_POINT('Ctrl Pts',(-19.4240588726576,-1.95677268946339,
0.069961262552598));
#30254=CARTESIAN_POINT('Ctrl Pts',(-19.4279874374395,-1.95347076783648,
0.138579280748551));
#30255=CARTESIAN_POINT('Ctrl Pts',(-19.4319160022213,-1.94623009822624,
0.206775368035542));
#30256=CARTESIAN_POINT('Ctrl Pts',(-19.4689291755589,-1.87801176042438,
0.849288280477544));
#30257=CARTESIAN_POINT('Ctrl Pts',(-19.5059423488964,-1.4601680051776,1.45434823304434));
#30258=CARTESIAN_POINT('Ctrl Pts',(-19.542955522234,-0.883489447908455,
1.7462425910547));
#30259=CARTESIAN_POINT('Ctrl Pts',(-19.5773036814893,-0.348332768864228,
2.01712003793654));
#30260=CARTESIAN_POINT('Ctrl Pts',(-19.6116518407447,0.323609377828236,
2.01830531561287));
#30261=CARTESIAN_POINT('Ctrl Pts',(-19.646,0.8635667682364,1.75638951800437));
#30262=CARTESIAN_POINT('',(-19.646,-0.861525859670563,1.75382131162753));
#30263=CARTESIAN_POINT('Origin',(-19.646,0.,0.));
#30264=CARTESIAN_POINT('Ctrl Pts',(-19.646,-0.861525859670562,1.75382131162753));
#30265=CARTESIAN_POINT('Ctrl Pts',(-19.6089868266624,-1.44419697921243,
1.46759703447886));
#30266=CARTESIAN_POINT('Ctrl Pts',(-19.5719736533249,-1.86803384659668,
0.870718499491397));
#30267=CARTESIAN_POINT('Ctrl Pts',(-19.5349604799873,-1.94348346552551,
0.229996089379168));
#30268=CARTESIAN_POINT('Ctrl Pts',(-19.5305968840329,-1.95237845134348,
0.154459369219161));
#30269=CARTESIAN_POINT('Ctrl Pts',(-19.5262332880786,-1.95643128236097,
0.0783132730520005));
#30270=CARTESIAN_POINT('Ctrl Pts',(-19.5218696921242,-1.95584467742209,
0.00207536885323489));
#30271=CARTESIAN_POINT('Origin',(-9.8,0.,0.));
#30272=CARTESIAN_POINT('',(-18.7201303078758,-1.95122552025463,0.000915013127814612));
#30273=CARTESIAN_POINT('',(-18.8218696921242,-1.95111957186981,0.000817319826409989));
#30274=CARTESIAN_POINT('',(-9.8,-1.954,-2.39295984553393E-16));
#30275=CARTESIAN_POINT('Ctrl Pts',(-18.7201303078758,-1.95122552025463,
0.000915013127814612));
#30276=CARTESIAN_POINT('Ctrl Pts',(-18.7353131659656,-1.95235483286073,
0.268087242358252));
#30277=CARTESIAN_POINT('Ctrl Pts',(-18.7504960240554,-1.90126484018336,
0.534845561933385));
#30278=CARTESIAN_POINT('Ctrl Pts',(-18.7656788821451,-1.79588180634386,
0.778079849513106));
#30279=CARTESIAN_POINT('Ctrl Pts',(-18.8026920554827,-1.53897625698858,
1.37104283412289));
#30280=CARTESIAN_POINT('Ctrl Pts',(-18.8397052288203,-0.959407278208984,
1.8242025460654));
#30281=CARTESIAN_POINT('Ctrl Pts',(-18.8767184021578,-0.321985378344434,
1.93051955012324));
#30282=CARTESIAN_POINT('Ctrl Pts',(-18.9137315754954,0.315436521520117,
2.03683655418109));
#30283=CARTESIAN_POINT('Ctrl Pts',(-18.950744748833,1.01071134246962,1.79631085035426));
#30284=CARTESIAN_POINT('Ctrl Pts',(-18.9877579221705,1.44615311561289,1.31881232311228));
#30285=CARTESIAN_POINT('Ctrl Pts',(-19.0247710955081,1.88159488875616,0.84131379587029));
#30286=CARTESIAN_POINT('Ctrl Pts',(-19.0617842688456,2.05720361409319,0.126842445213142));
#30287=CARTESIAN_POINT('Ctrl Pts',(-19.0987974421832,1.89275097145487,-0.498093241961312));
#30288=CARTESIAN_POINT('Ctrl Pts',(-19.1358106155208,1.72829832881656,-1.12302892913577));
#30289=CARTESIAN_POINT('Ctrl Pts',(-19.1728237888583,1.22378431820289,-1.65842895282753));
#30290=CARTESIAN_POINT('Ctrl Pts',(-19.2098369621959,0.609709882174192,
-1.85976901676034));
#30291=CARTESIAN_POINT('Ctrl Pts',(-19.2468501355335,-0.00436455385450528,
-2.06110908069315));
#30292=CARTESIAN_POINT('Ctrl Pts',(-19.283863308871,-0.727999415298231,
-1.92838918486701));
#30293=CARTESIAN_POINT('Ctrl Pts',(-19.3208764822086,-1.23052038584163,
-1.52204630079534));
#30294=CARTESIAN_POINT('Ctrl Pts',(-19.3539610907643,-1.67970396299246,
-1.15883250293187));
#30295=CARTESIAN_POINT('Ctrl Pts',(-19.3870456993201,-1.95222055983625,
-0.576997672807184));
#30296=CARTESIAN_POINT('Ctrl Pts',(-19.4201303078758,-1.95628952807724,
0.00129327600707104));
#30297=CARTESIAN_POINT('Ctrl Pts',(-19.5218696921242,-1.95584467742209,
0.00207536885323489));
#30298=CARTESIAN_POINT('Ctrl Pts',(-19.489220114741,-1.95145554434339,-0.568356765264027));
#30299=CARTESIAN_POINT('Ctrl Pts',(-19.4565705373578,-1.68733094748134,
-1.14392870557586));
#30300=CARTESIAN_POINT('Ctrl Pts',(-19.4239209599746,-1.24838760910815,
-1.50783684792128));
#30301=CARTESIAN_POINT('Ctrl Pts',(-19.386907786637,-0.750779763288562,
-1.92038108987251));
#30302=CARTESIAN_POINT('Ctrl Pts',(-19.3498946132995,-0.0285017011759892,
-2.06090328853796));
#30303=CARTESIAN_POINT('Ctrl Pts',(-19.3128814399619,0.587948268210155,
-1.86661002179603));
#30304=CARTESIAN_POINT('Ctrl Pts',(-19.2758682666244,1.2043982375963,-1.6723167550541));
#30305=CARTESIAN_POINT('Ctrl Pts',(-19.2388550932868,1.71502011425601,-1.14320802290478));
#30306=CARTESIAN_POINT('Ctrl Pts',(-19.2018419199492,1.8867513877996,-0.520323693783771));
#30307=CARTESIAN_POINT('Ctrl Pts',(-19.1648287466117,2.0584826613432,0.102560635337238));
#30308=CARTESIAN_POINT('Ctrl Pts',(-19.1278155732741,1.89132333177067,0.819220561429935));
#30309=CARTESIAN_POINT('Ctrl Pts',(-19.0908023999365,1.46152107494396,1.30183002295279));
#30310=CARTESIAN_POINT('Ctrl Pts',(-19.053789226599,1.03171881811726,1.78443948447564));
#30311=CARTESIAN_POINT('Ctrl Pts',(-19.0167760532614,0.339273634036384,
2.03299848142864));
#30312=CARTESIAN_POINT('Ctrl Pts',(-18.9797628799238,-0.299358392794465,
1.93413318743984));
#30313=CARTESIAN_POINT('Ctrl Pts',(-18.9427497065863,-0.937990419625319,
1.83526789345104));
#30314=CARTESIAN_POINT('Ctrl Pts',(-18.9057365332487,-1.52280928920615,
1.38897830852044));
#30315=CARTESIAN_POINT('Ctrl Pts',(-18.8687233599112,-1.78663886004406,
0.799077292011544));
#30316=CARTESIAN_POINT('Ctrl Pts',(-18.8531054706488,-1.89796303600405,
0.550165677016122));
#30317=CARTESIAN_POINT('Ctrl Pts',(-18.8374875813865,-1.95213637563171,
0.275684631968902));
#30318=CARTESIAN_POINT('Ctrl Pts',(-18.8218696921242,-1.95111957186981,
0.000817319826409989));
#30319=CARTESIAN_POINT('Origin',(-9.8,0.,0.));
#30320=CARTESIAN_POINT('',(-18.0201303078758,-1.95299307732975,-0.00171153559867271));
#30321=CARTESIAN_POINT('',(-18.1218696921242,-1.95320927907148,-0.00174204714352619));
#30322=CARTESIAN_POINT('',(-9.8,-1.954,-2.39295984553393E-16));
#30323=CARTESIAN_POINT('Ctrl Pts',(-18.0201303078758,-1.95299307732975,
-0.00171153559867271));
#30324=CARTESIAN_POINT('Ctrl Pts',(-18.0465674592735,-1.94907576194016,
0.462441490461123));
#30325=CARTESIAN_POINT('Ctrl Pts',(-18.0730046106712,-1.78336958701272,
0.929108469286399));
#30326=CARTESIAN_POINT('Ctrl Pts',(-18.099441762069,-1.48183519126904,1.27857813100852));
#30327=CARTESIAN_POINT('Ctrl Pts',(-18.1364549354065,-1.05967379085981,
1.76785100957778));
#30328=CARTESIAN_POINT('Ctrl Pts',(-18.1734681087441,-0.371272370021996,
2.02740273070118));
#30329=CARTESIAN_POINT('Ctrl Pts',(-18.2104812820817,0.268828848722206,
1.93864079577349));
#30330=CARTESIAN_POINT('Ctrl Pts',(-18.2474944554192,0.908930067466409,
1.84987886084581));
#30331=CARTESIAN_POINT('Ctrl Pts',(-18.2845076287568,1.50073108411699,1.41280326986704));
#30332=CARTESIAN_POINT('Ctrl Pts',(-18.3215208020944,1.77382959268256,0.827119374505746));
#30333=CARTESIAN_POINT('Ctrl Pts',(-18.3585339754319,2.04692810124813,0.24143547914445));
#30334=CARTESIAN_POINT('Ctrl Pts',(-18.3955471487695,2.00132410172869,-0.492856720599384));
#30335=CARTESIAN_POINT('Ctrl Pts',(-18.4325603221071,1.65785490807018,-1.04024761341585));
#30336=CARTESIAN_POINT('Ctrl Pts',(-18.4695734954446,1.31438571441166,-1.58763850623231));
#30337=CARTESIAN_POINT('Ctrl Pts',(-18.5065866687822,0.673051326614071,
-1.94812809212141));
#30338=CARTESIAN_POINT('Ctrl Pts',(-18.5435998421197,0.0268860436523521,
-1.95700588033934));
#30339=CARTESIAN_POINT('Ctrl Pts',(-18.5806130154573,-0.619279239309369,
-1.96588366855727));
#30340=CARTESIAN_POINT('Ctrl Pts',(-18.6176261887949,-1.27027541743522,
-1.62314965910403));
#30341=CARTESIAN_POINT('Ctrl Pts',(-18.6546393621324,-1.62865244653266,
-1.08539952573888));
#30342=CARTESIAN_POINT('Ctrl Pts',(-18.6764696773802,-1.84002269169937,
-0.768235287243793));
#30343=CARTESIAN_POINT('Ctrl Pts',(-18.698299992628,-1.94960176469699,-0.3832322900387));
#30344=CARTESIAN_POINT('Ctrl Pts',(-18.7201303078758,-1.95122552025463,
0.000915013127814612));
#30345=CARTESIAN_POINT('Ctrl Pts',(-18.8218696921242,-1.95111957186981,
0.000817319826409989));
#30346=CARTESIAN_POINT('Ctrl Pts',(-18.800474408049,-1.94972663041856,-0.375729352231495));
#30347=CARTESIAN_POINT('Ctrl Pts',(-18.7790791239737,-1.84475916201458,
-0.753000926042014));
#30348=CARTESIAN_POINT('Ctrl Pts',(-18.7576838398985,-1.64125793500757,
-1.06625371430635));
#30349=CARTESIAN_POINT('Ctrl Pts',(-18.7206706665609,-1.28920716703816,
-1.60817125602816));
#30350=CARTESIAN_POINT('Ctrl Pts',(-18.6836574932233,-0.642265359004347,
-1.95849389138462));
#30351=CARTESIAN_POINT('Ctrl Pts',(-18.6466443198858,0.00396079527596547,
-1.95718277265247));
#30352=CARTESIAN_POINT('Ctrl Pts',(-18.6096311465482,0.650186949556277,
-1.95587165392032));
#30353=CARTESIAN_POINT('Ctrl Pts',(-18.5726179732106,1.29569745008309,-1.60292678109958));
#30354=CARTESIAN_POINT('Ctrl Pts',(-18.5356047998731,1.64555468172952,-1.05959865244045));
#30355=CARTESIAN_POINT('Ctrl Pts',(-18.4985916265355,1.99541191337596,-0.516270523781318));
#30356=CARTESIAN_POINT('Ctrl Pts',(-18.4615784531979,2.04961587614203,0.2174408607162));
#30357=CARTESIAN_POINT('Ctrl Pts',(-18.4245652798604,1.78339728471467,0.80628459334565));
#30358=CARTESIAN_POINT('Ctrl Pts',(-18.3875521065228,1.51717869328732,1.3951283259751));
#30359=CARTESIAN_POINT('Ctrl Pts',(-18.3505389331852,0.930537547666546,
1.83910440673648));
#30360=CARTESIAN_POINT('Ctrl Pts',(-18.3135257598477,0.291519864690383,
1.93535806385024));
#30361=CARTESIAN_POINT('Ctrl Pts',(-18.2765125865101,-0.34749781828578,
2.03161172096399));
#30362=CARTESIAN_POINT('Ctrl Pts',(-18.2394994131726,-1.03889203861734,
1.78014295443012));
#30363=CARTESIAN_POINT('Ctrl Pts',(-18.202486239835,-1.46675581987468,1.29584920213102));
#30364=CARTESIAN_POINT('Ctrl Pts',(-18.1756140572647,-1.77739207741162,
0.944243842311544));
#30365=CARTESIAN_POINT('Ctrl Pts',(-18.1487418746945,-1.94912136870076,
0.46991636905064));
#30366=CARTESIAN_POINT('Ctrl Pts',(-18.1218696921242,-1.95320927907148,
-0.00174204714352619));
#30367=CARTESIAN_POINT('Origin',(-9.8,0.,0.));
#30368=CARTESIAN_POINT('',(-17.3201303078758,-1.95716036932443,0.000219777629121352));
#30369=CARTESIAN_POINT('',(-17.4218696921242,-1.95710975664994,0.000358848027250084));
#30370=CARTESIAN_POINT('',(-9.8,-1.954,-2.39295984553393E-16));
#30371=CARTESIAN_POINT('Ctrl Pts',(-17.3201303078758,-1.95716036932443,
0.000219777629121352));
#30372=CARTESIAN_POINT('Ctrl Pts',(-17.3208085792439,-1.95717926909536,
0.0120624621000906));
#30373=CARTESIAN_POINT('Ctrl Pts',(-17.321486850612,-1.95708105723414,0.0239048246808731));
#30374=CARTESIAN_POINT('Ctrl Pts',(-17.3221651219801,-1.95686477834934,
0.0357450305932741));
#30375=CARTESIAN_POINT('Ctrl Pts',(-17.3591782953177,-1.94506246996874,
0.68186340501921));
#30376=CARTESIAN_POINT('Ctrl Pts',(-17.3961914686552,-1.58167196389125,
1.32155950228172));
#30377=CARTESIAN_POINT('Ctrl Pts',(-17.4332046419928,-1.03273148765314,
1.66254718585494));
#30378=CARTESIAN_POINT('Ctrl Pts',(-17.4702178153304,-0.483791011415034,
2.00353486942816));
#30379=CARTESIAN_POINT('Ctrl Pts',(-17.507230988668,0.250699434983697,2.04581413931209));
#30380=CARTESIAN_POINT('Ctrl Pts',(-17.5442441620055,0.835140850126002,
1.77006701011294));
#30381=CARTESIAN_POINT('Ctrl Pts',(-17.5812573353431,1.41958226526831,1.4943198809138));
#30382=CARTESIAN_POINT('Ctrl Pts',(-17.6182705086806,1.85397464915419,0.900546352631588));
#30383=CARTESIAN_POINT('Ctrl Pts',(-17.6552836820182,1.93983801723647,0.260049878109278));
#30384=CARTESIAN_POINT('Ctrl Pts',(-17.6922968553558,2.02570138531875,-0.380446596413026));
#30385=CARTESIAN_POINT('Ctrl Pts',(-17.7293100286933,1.76303573759744,-1.06766601717542));
#30386=CARTESIAN_POINT('Ctrl Pts',(-17.7663232020309,1.27185670261682,-1.48760815212437));
#30387=CARTESIAN_POINT('Ctrl Pts',(-17.8033363753685,0.780677667636197,
-1.90755028707332));
#30388=CARTESIAN_POINT('Ctrl Pts',(-17.840349548706,0.0609852453962589,
-2.06021513620881));
#30389=CARTESIAN_POINT('Ctrl Pts',(-17.8773627220436,-0.558382994856356,
-1.875848033151));
#30390=CARTESIAN_POINT('Ctrl Pts',(-17.9143758953811,-1.17775123510897,
-1.69148093009319));
#30391=CARTESIAN_POINT('Ctrl Pts',(-17.9513890687187,-1.69679529337426,
-1.17008187484208));
#30392=CARTESIAN_POINT('Ctrl Pts',(-17.9884022420563,-1.87835663251658,
-0.54988532920897));
#30393=CARTESIAN_POINT('Ctrl Pts',(-17.9989782639961,-1.93023537008609,
-0.372672416017184));
#30394=CARTESIAN_POINT('Ctrl Pts',(-18.0095542859359,-1.95456017557276,
-0.187393136206644));
#30395=CARTESIAN_POINT('Ctrl Pts',(-18.0201303078758,-1.95299307732975,
-0.00171153559867271));
#30396=CARTESIAN_POINT('Ctrl Pts',(-18.1218696921242,-1.95320927907148,
-0.00174204714352619));
#30397=CARTESIAN_POINT('Ctrl Pts',(-18.1117287013569,-1.95475196959239,
-0.179735912414574));
#30398=CARTESIAN_POINT('Ctrl Pts',(-18.1015877105896,-1.93242005916289,
-0.357349664660824));
#30399=CARTESIAN_POINT('Ctrl Pts',(-18.0914467198223,-1.88466923704063,
-0.527844244331786));
#30400=CARTESIAN_POINT('Ctrl Pts',(-18.0544335464847,-1.71038553076609,
-1.15012520043117));
#30401=CARTESIAN_POINT('Ctrl Pts',(-18.0174203731472,-1.19748477603389,
-1.67756837456562));
#30402=CARTESIAN_POINT('Ctrl Pts',(-17.9804071998096,-0.580318741193403,
-1.86917817188516));
#30403=CARTESIAN_POINT('Ctrl Pts',(-17.943394026472,0.0368472936470773,
-2.0607879692047));
#30404=CARTESIAN_POINT('Ctrl Pts',(-17.9063808531345,0.758278608595835,
-1.91656438970933));
#30405=CARTESIAN_POINT('Ctrl Pts',(-17.8693676797969,1.25434321128846,-1.50240489715304));
#30406=CARTESIAN_POINT('Ctrl Pts',(-17.8323545064593,1.75040781398108,-1.08824540459674));
#30407=CARTESIAN_POINT('Ctrl Pts',(-17.7953413331218,2.02110570441758,-0.404149998979508));
#30408=CARTESIAN_POINT('Ctrl Pts',(-17.7583281597842,1.94275115623478,0.237308353210707));
#30409=CARTESIAN_POINT('Ctrl Pts',(-17.7213149864467,1.86439660805198,0.878766705400926));
#30410=CARTESIAN_POINT('Ctrl Pts',(-17.6843018131091,1.43698962124989,1.47758800416414));
#30411=CARTESIAN_POINT('Ctrl Pts',(-17.6472886397715,0.855818482331675,
1.7601624734435));
#30412=CARTESIAN_POINT('Ctrl Pts',(-17.610275466434,0.274647343413464,2.04273694272287));
#30413=CARTESIAN_POINT('Ctrl Pts',(-17.5732622930964,-0.460287947620861,
2.00906458251839));
#30414=CARTESIAN_POINT('Ctrl Pts',(-17.5362491197588,-1.01318514831372,
1.6745307213773));
#30415=CARTESIAN_POINT('Ctrl Pts',(-17.4992359464213,-1.56608234900657,
1.33999686023621));
#30416=CARTESIAN_POINT('Ctrl Pts',(-17.4622227730837,-1.93694145935795,
0.704601498158489));
#30417=CARTESIAN_POINT('Ctrl Pts',(-17.4252095997461,-1.9563117338864,0.0586657258015617));
#30418=CARTESIAN_POINT('Ctrl Pts',(-17.4240962972055,-1.95689436363416,
0.0392369151482447));
#30419=CARTESIAN_POINT('Ctrl Pts',(-17.4229829946649,-1.95715899471935,
0.0197985683844457));
#30420=CARTESIAN_POINT('Ctrl Pts',(-17.4218696921242,-1.95710975664994,
0.000358848027250084));
#30421=CARTESIAN_POINT('Origin',(-9.8,0.,0.));
#30422=CARTESIAN_POINT('',(-16.6201303078758,-1.95236106975453,0.00156080202577326));
#30423=CARTESIAN_POINT('',(-16.7218696921242,-1.95217490710565,0.00149575073417193));
#30424=CARTESIAN_POINT('',(-9.8,-1.954,-2.39295984553393E-16));
#30425=CARTESIAN_POINT('Ctrl Pts',(-16.6201303078758,-1.95236106975453,
0.00156080202577326));
#30426=CARTESIAN_POINT('Ctrl Pts',(-16.6320628725518,-1.95393611722315,
0.211230577376388));
#30427=CARTESIAN_POINT('Ctrl Pts',(-16.6439954372279,-1.92281737418396,
0.420445287656267));
#30428=CARTESIAN_POINT('Ctrl Pts',(-16.655928001904,-1.85702132802313,0.618117508955001));
#30429=CARTESIAN_POINT('Ctrl Pts',(-16.6929411752415,-1.65293104839012,
1.23126953365152));
#30430=CARTESIAN_POINT('Ctrl Pts',(-16.7299543485791,-1.11519135743181,
1.73336492166902));
#30431=CARTESIAN_POINT('Ctrl Pts',(-16.7669675219167,-0.489503073786642,
1.89498923702786));
#30432=CARTESIAN_POINT('Ctrl Pts',(-16.8039806952542,0.136185209858534,
2.0566135523867));
#30433=CARTESIAN_POINT('Ctrl Pts',(-16.8409938685918,0.849822086190574,
1.87776679508686));
#30434=CARTESIAN_POINT('Ctrl Pts',(-16.8780070419294,1.32533684172017,1.44016656101051));
#30435=CARTESIAN_POINT('Ctrl Pts',(-16.9150202152669,1.80085159724978,1.00256632693417));
#30436=CARTESIAN_POINT('Ctrl Pts',(-16.9520333886045,2.03824423197693,0.306212616081319));
#30437=CARTESIAN_POINT('Ctrl Pts',(-16.989046561942,1.92904671630549,-0.330720779401667));
#30438=CARTESIAN_POINT('Ctrl Pts',(-17.0260597352796,1.81984920063405,-0.96765417488465));
#30439=CARTESIAN_POINT('Ctrl Pts',(-17.0630729086172,1.36406153456402,-1.54516725499777));
#30440=CARTESIAN_POINT('Ctrl Pts',(-17.1000860819547,0.769939505430447,
-1.79938618037108));
#30441=CARTESIAN_POINT('Ctrl Pts',(-17.1370992552923,0.175817476296884,
-2.05360510574439));
#30442=CARTESIAN_POINT('Ctrl Pts',(-17.1741124286299,-0.556638915900209,
-1.9845298763779));
#30443=CARTESIAN_POINT('Ctrl Pts',(-17.2111256019674,-1.09276005665691,
-1.62372193589998));
#30444=CARTESIAN_POINT('Ctrl Pts',(-17.2474605039369,-1.61905670556847,
-1.26952584934724));
#30445=CARTESIAN_POINT('Ctrl Pts',(-17.2837954059063,-1.95614791124902,
-0.634191166918971));
#30446=CARTESIAN_POINT('Ctrl Pts',(-17.3201303078758,-1.95716036932443,
0.000219777629121352));
#30447=CARTESIAN_POINT('Ctrl Pts',(-17.4218696921242,-1.95710975664994,
0.000358848027250084));
#30448=CARTESIAN_POINT('Ctrl Pts',(-17.3859698213273,-1.95552201184067,
-0.626499911094741));
#30449=CARTESIAN_POINT('Ctrl Pts',(-17.3500699505304,-1.62756593762931,
-1.25478696406307));
#30450=CARTESIAN_POINT('Ctrl Pts',(-17.3141700797335,-1.11170569044781,
-1.61080964516247));
#30451=CARTESIAN_POINT('Ctrl Pts',(-17.2771569063959,-0.579847933775247,
-1.97787306113345));
#30452=CARTESIAN_POINT('Ctrl Pts',(-17.2401437330583,0.151749018275395,
-2.05552371043926));
#30453=CARTESIAN_POINT('Ctrl Pts',(-17.2031305597207,0.748808243613774,
-1.80828191396906));
#30454=CARTESIAN_POINT('Ctrl Pts',(-17.1661173863832,1.34586746895216,-1.56104011749885));
#30455=CARTESIAN_POINT('Ctrl Pts',(-17.1291042130456,1.80838896757828,-0.988905875252619));
#30456=CARTESIAN_POINT('Ctrl Pts',(-17.0920910397081,1.92504016834594,-0.353295362990227));
#30457=CARTESIAN_POINT('Ctrl Pts',(-17.0550778663705,2.04169136911361,0.282315149272168));
#30458=CARTESIAN_POINT('Ctrl Pts',(-17.0180646930329,1.81247227202281,0.981401931550726));
#30459=CARTESIAN_POINT('Ctrl Pts',(-16.9810515196954,1.34211630309758,1.42454241453319));
#30460=CARTESIAN_POINT('Ctrl Pts',(-16.9440383463578,0.871760334172357,
1.86768289751565));
#30461=CARTESIAN_POINT('Ctrl Pts',(-16.9070251730202,0.160267493412704,
2.05487708120202));
#30462=CARTESIAN_POINT('Ctrl Pts',(-16.8700119996827,-0.467271145973578,
1.9005933125143));
#30463=CARTESIAN_POINT('Ctrl Pts',(-16.8329988263451,-1.09480978535987,
1.74630954382658));
#30464=CARTESIAN_POINT('Ctrl Pts',(-16.7959856530075,-1.63839422337278,
1.25054782276476));
#30465=CARTESIAN_POINT('Ctrl Pts',(-16.75897247967,-1.84965309417818,0.639828644336359));
#30466=CARTESIAN_POINT('Ctrl Pts',(-16.7466048838214,-1.92024321380182,
0.435762705247683));
#30467=CARTESIAN_POINT('Ctrl Pts',(-16.7342372879728,-1.95372925218912,
0.218861789684893));
#30468=CARTESIAN_POINT('Ctrl Pts',(-16.7218696921242,-1.95217490710565,
0.00149575073417193));
#30469=CARTESIAN_POINT('Origin',(-9.8,0.,0.));
#30470=CARTESIAN_POINT('',(-15.9201303078758,-1.9516232757602,-0.00122528121799068));
#30471=CARTESIAN_POINT('',(-16.0218696921242,-1.951775199121,-0.00131382171386765));
#30472=CARTESIAN_POINT('',(-9.8,-1.954,-2.39295984553393E-16));
#30473=CARTESIAN_POINT('Ctrl Pts',(-15.9201303078758,-1.9516232757602,-0.00122528121799068));
#30474=CARTESIAN_POINT('Ctrl Pts',(-15.9433171658598,-1.94927914488889,
0.406583857041756));
#30475=CARTESIAN_POINT('Ctrl Pts',(-15.9665040238438,-1.82458420503018,
0.81570542027797));
#30476=CARTESIAN_POINT('Ctrl Pts',(-15.9896908818278,-1.58792615951522,
1.14415382687092));
#30477=CARTESIAN_POINT('Ctrl Pts',(-16.0267040551654,-1.21014900374817,
1.66845590411029));
#30478=CARTESIAN_POINT('Ctrl Pts',(-16.0637172285029,-0.547070532187443,
1.98718885565735));
#30479=CARTESIAN_POINT('Ctrl Pts',(-16.1007304018405,0.0983393870045533,
1.95471911859019));
#30480=CARTESIAN_POINT('Ctrl Pts',(-16.1377435751781,0.743749306196545,
1.92224938152302));
#30481=CARTESIAN_POINT('Ctrl Pts',(-16.1747567485156,1.37149067301981,1.53857695584164));
#30482=CARTESIAN_POINT('Ctrl Pts',(-16.2117699218532,1.69473963886053,0.979007162429953));
#30483=CARTESIAN_POINT('Ctrl Pts',(-16.2487830951907,2.01798860470126,0.41943736901826));
#30484=CARTESIAN_POINT('Ctrl Pts',(-16.2857962685283,2.03674516955944,-0.316029792123737));
#30485=CARTESIAN_POINT('Ctrl Pts',(-16.3228094418659,1.74243919547003,-0.89134904369965));
#30486=CARTESIAN_POINT('Ctrl Pts',(-16.3598226152035,1.44813322138062,-1.46666829527556));
#30487=CARTESIAN_POINT('Ctrl Pts',(-16.396835788541,0.840764708343617,-1.88183963728539));
#30488=CARTESIAN_POINT('Ctrl Pts',(-16.4338489618786,0.197848861895412,
-1.94716545148987));
#30489=CARTESIAN_POINT('Ctrl Pts',(-16.4708621352161,-0.445066984552789,
-2.01249126569435));
#30490=CARTESIAN_POINT('Ctrl Pts',(-16.5078753085537,-1.12353016441219,
-1.72797155209348));
#30491=CARTESIAN_POINT('Ctrl Pts',(-16.5448884818913,-1.52754132018803,
-1.22360736460528));
#30492=CARTESIAN_POINT('Ctrl Pts',(-16.5699690905528,-1.8013045449859,-0.881843617576629));
#30493=CARTESIAN_POINT('Ctrl Pts',(-16.5950496992143,-1.94905053675042,
-0.439136208756951));
#30494=CARTESIAN_POINT('Ctrl Pts',(-16.6201303078758,-1.95236106975453,
0.00156080202577326));
#30495=CARTESIAN_POINT('Ctrl Pts',(-16.7218696921242,-1.95217490710565,
0.00149575073417193));
#30496=CARTESIAN_POINT('Ctrl Pts',(-16.6972241146353,-1.94907747954834,
-0.431661317302269));
#30497=CARTESIAN_POINT('Ctrl Pts',(-16.6725785371463,-1.80683227309339,
-0.866665422383789));
#30498=CARTESIAN_POINT('Ctrl Pts',(-16.6479329596573,-1.54177007931888,
-1.20562941457546));
#30499=CARTESIAN_POINT('Ctrl Pts',(-16.6109197863197,-1.14369489005632,
-1.71469165926392));
#30500=CARTESIAN_POINT('Ctrl Pts',(-16.5739066129822,-0.468611207933312,
-2.00713951284586));
#30501=CARTESIAN_POINT('Ctrl Pts',(-16.5368934396446,0.175025749589254,
-1.9493494427573));
#30502=CARTESIAN_POINT('Ctrl Pts',(-16.499880266307,0.818662707111826,-1.89155937266874));
#30503=CARTESIAN_POINT('Ctrl Pts',(-16.4628670929695,1.43085294003395,-1.48353137890967));
#30504=CARTESIAN_POINT('Ctrl Pts',(-16.4258539196319,1.73187813124758,-0.91169918362098));
#30505=CARTESIAN_POINT('Ctrl Pts',(-16.3888407462943,2.0329033224612,-0.33986698833229));
#30506=CARTESIAN_POINT('Ctrl Pts',(-16.3518275729568,2.02276347196631,0.395769408486024));
#30507=CARTESIAN_POINT('Ctrl Pts',(-16.3148143996192,1.70609161990569,0.959087403412657));
#30508=CARTESIAN_POINT('Ctrl Pts',(-16.2778012262816,1.38941976784508,1.52240539833928));
#30509=CARTESIAN_POINT('Ctrl Pts',(-16.2407880529441,0.766215914218737,
1.91340499137424));
#30510=CARTESIAN_POINT('Ctrl Pts',(-16.2037748796065,0.121230654114145,
1.95343297592505));
#30511=CARTESIAN_POINT('Ctrl Pts',(-16.166761706269,-0.523754605990456,
1.99346096047586));
#30512=CARTESIAN_POINT('Ctrl Pts',(-16.1297485329314,-1.19052127257331,
1.68251733654252));
#30513=CARTESIAN_POINT('Ctrl Pts',(-16.0927353595938,-1.57441428935352,
1.1626766138498));
#30514=CARTESIAN_POINT('Ctrl Pts',(-16.0691134704373,-1.81941566244965,
0.830913113905955));
#30515=CARTESIAN_POINT('Ctrl Pts',(-16.0454915812807,-1.94920201372017,
0.41406539417118));
#30516=CARTESIAN_POINT('Ctrl Pts',(-16.0218696921242,-1.951775199121,-0.00131382171386765));
#30517=CARTESIAN_POINT('Origin',(-9.8,0.,0.));
#30518=CARTESIAN_POINT('',(-15.2201303078758,-1.95678697592279,-0.000800724488720095));
#30519=CARTESIAN_POINT('',(-15.3218696921242,-1.95690589693301,-0.000674027605478421));
#30520=CARTESIAN_POINT('',(-9.8,-1.954,-2.39295984553393E-16));
#30521=CARTESIAN_POINT('Ctrl Pts',(-15.2201303078758,-1.95678697592279,
-0.000800724488720095));
#30522=CARTESIAN_POINT('Ctrl Pts',(-15.2545714591677,-1.95366270876428,
0.600851523163264));
#30523=CARTESIAN_POINT('Ctrl Pts',(-15.2890126104597,-1.65520957823559,
1.20518249057995));
#30524=CARTESIAN_POINT('Ctrl Pts',(-15.3234537617516,-1.17410501132559,
1.56591024327599));
#30525=CARTESIAN_POINT('Ctrl Pts',(-15.3604669350892,-0.657072157877076,
1.95357669278071));
#30526=CARTESIAN_POINT('Ctrl Pts',(-15.3974801084268,0.0709111245972353,
2.05989740706708));
#30527=CARTESIAN_POINT('Ctrl Pts',(-15.4344932817643,0.677219048087142,
1.83629295825163));
#30528=CARTESIAN_POINT('Ctrl Pts',(-15.4715064551019,1.28352697157704,1.61268850943619));
#30529=CARTESIAN_POINT('Ctrl Pts',(-15.5085196284395,1.76815953608255,1.05915889751893));
#30530=CARTESIAN_POINT('Ctrl Pts',(-15.545532801777,1.90968131507004,0.428619577818016));
#30531=CARTESIAN_POINT('Ctrl Pts',(-15.5825459751146,2.05120309405753,-0.201919741882898));
#30532=CARTESIAN_POINT('Ctrl Pts',(-15.6195591484522,1.84961408752702,-0.909468769367463));
#30533=CARTESIAN_POINT('Ctrl Pts',(-15.6565723217897,1.39702314435684,-1.37073841477789));
#30534=CARTESIAN_POINT('Ctrl Pts',(-15.6935854951273,0.944432201186666,
-1.83200806018831));
#30535=CARTESIAN_POINT('Ctrl Pts',(-15.7305986684648,0.240839321376827,
-2.0469983235246));
#30536=CARTESIAN_POINT('Ctrl Pts',(-15.7676118418024,-0.392274024660755,
-1.91747713342123));
#30537=CARTESIAN_POINT('Ctrl Pts',(-15.80462501514,-1.02538737069834,-1.78795594331785));
#30538=CARTESIAN_POINT('Ctrl Pts',(-15.8416381884775,-1.58802118296367,
-1.31392329977481));
#30539=CARTESIAN_POINT('Ctrl Pts',(-15.8786513618151,-1.82310016910965,
-0.71197137653746));
#30540=CARTESIAN_POINT('Ctrl Pts',(-15.8924776771687,-1.91091420671742,
-0.487111512660019));
#30541=CARTESIAN_POINT('Ctrl Pts',(-15.9063039925222,-1.95302108018369,
-0.244401728562753));
#30542=CARTESIAN_POINT('Ctrl Pts',(-15.9201303078758,-1.9516232757602,-0.00122528121799068));
#30543=CARTESIAN_POINT('Ctrl Pts',(-16.0218696921242,-1.951775199121,-0.00131382171386765));
#30544=CARTESIAN_POINT('Ctrl Pts',(-16.0084784079432,-1.95323394176112,
-0.236792918493611));
#30545=CARTESIAN_POINT('Ctrl Pts',(-15.9950871237622,-1.91380926057871,
-0.471800071470502));
#30546=CARTESIAN_POINT('Ctrl Pts',(-15.9816958395811,-1.8313152224601,-0.690566303043669));
#30547=CARTESIAN_POINT('Ctrl Pts',(-15.9446826662436,-1.60330377180891,
-1.29523067579235));
#30548=CARTESIAN_POINT('Ctrl Pts',(-15.907669492906,-1.04626150352895,-1.77582159983761));
#30549=CARTESIAN_POINT('Ctrl Pts',(-15.8706563195684,-0.414708854972982,
-1.91275033094355));
#30550=CARTESIAN_POINT('Ctrl Pts',(-15.8336431462309,0.216843793582987,
-2.0496790620495));
#30551=CARTESIAN_POINT('Ctrl Pts',(-15.7966299728933,0.922906822414965,
-1.84294560021614));
#30552=CARTESIAN_POINT('Ctrl Pts',(-15.7596167995557,1.38087011532323,-1.38700936821731));
#30553=CARTESIAN_POINT('Ctrl Pts',(-15.7226036262182,1.83883340823148,-0.931073136218487));
#30554=CARTESIAN_POINT('Ctrl Pts',(-15.6855904528806,2.04869696521603,-0.225934134054202));
#30555=CARTESIAN_POINT('Ctrl Pts',(-15.648577279543,1.9145711790607,0.406219722841795));
#30556=CARTESIAN_POINT('Ctrl Pts',(-15.6115641062055,1.78044539290536,1.0383735797378));
#30557=CARTESIAN_POINT('Ctrl Pts',(-15.5745509328679,1.30233026361014,1.59754229136552));
#30558=CARTESIAN_POINT('Ctrl Pts',(-15.5375377595304,0.698683310008129,
1.82823381853421));
#30559=CARTESIAN_POINT('Ctrl Pts',(-15.5005245861928,0.0950363564061148,
2.05892534570289));
#30560=CARTESIAN_POINT('Ctrl Pts',(-15.4635114128552,-0.634142421502691,
1.96113968841256));
#30561=CARTESIAN_POINT('Ctrl Pts',(-15.4264982395177,-1.15568099705043,
1.5795564871103));
#30562=CARTESIAN_POINT('Ctrl Pts',(-15.3916220570532,-1.64710804539289,
1.22000435596431));
#30563=CARTESIAN_POINT('Ctrl Pts',(-15.3567458745887,-1.95417934548115,
0.608479302503191));
#30564=CARTESIAN_POINT('Ctrl Pts',(-15.3218696921242,-1.95690589693301,
-0.000674027605478421));
#30565=CARTESIAN_POINT('Origin',(-9.8,0.,0.));
#30566=CARTESIAN_POINT('',(-14.5201303078758,-1.95396550297987,0.00177712178281789));
#30567=CARTESIAN_POINT('',(-14.6218696921242,-1.95373627769492,0.00177775396232179));
#30568=CARTESIAN_POINT('',(-9.8,-1.954,-2.39295984553393E-16));
#30569=CARTESIAN_POINT('Ctrl Pts',(-14.5201303078758,-1.95396550297987,
0.00177712178281789));
#30570=CARTESIAN_POINT('Ctrl Pts',(-14.5288125791381,-1.95535803437996,
0.154017333838736));
#30571=CARTESIAN_POINT('Ctrl Pts',(-14.5374948504005,-1.93906235797112,
0.305962769432957));
#30572=CARTESIAN_POINT('Ctrl Pts',(-14.5461771216628,-1.90394399117853,
0.453425568392138));
#30573=CARTESIAN_POINT('Ctrl Pts',(-14.5831902950004,-1.75423176057083,
1.08207053625807));
#30574=CARTESIAN_POINT('Ctrl Pts',(-14.6202034683379,-1.26243956445243,
1.62924892552931));
#30575=CARTESIAN_POINT('Ctrl Pts',(-14.6572166416755,-0.65327416561486,
1.84494724373267));
#30576=CARTESIAN_POINT('Ctrl Pts',(-14.6942298150131,-0.0441087667772883,
2.06064556193603));
#30577=CARTESIAN_POINT('Ctrl Pts',(-14.7312429883506,0.682429834779477,
1.9448638090715));
#30578=CARTESIAN_POINT('Ctrl Pts',(-14.7682561616882,1.1943759460504,1.55050429445157));
#30579=CARTESIAN_POINT('Ctrl Pts',(-14.8052693350257,1.70632205732133,1.15614477983164));
#30580=CARTESIAN_POINT('Ctrl Pts',(-14.8422825083633,2.00367567830644,0.48320750345631));
#30581=CARTESIAN_POINT('Ctrl Pts',(-14.8792956817009,1.95057176254247,-0.160833040102267));
#30582=CARTESIAN_POINT('Ctrl Pts',(-14.9163088550384,1.89746784677849,-0.804873583660848));
#30583=CARTESIAN_POINT('Ctrl Pts',(-14.953322028376,1.49390639426542,-1.42001739440267));
#30584=CARTESIAN_POINT('Ctrl Pts',(-14.9903352017136,0.924280301631946,
-1.72519662404948));
#30585=CARTESIAN_POINT('Ctrl Pts',(-15.0273483750511,0.35465420899847,-2.03037585369629));
#30586=CARTESIAN_POINT('Ctrl Pts',(-15.0643615483887,-0.381036523755413,
-2.02559050224809));
#30587=CARTESIAN_POINT('Ctrl Pts',(-15.1013747217263,-0.946644466317395,
-1.71302706400314));
#30588=CARTESIAN_POINT('Ctrl Pts',(-15.1383878950638,-1.51225240887937,
-1.4004636257582));
#30589=CARTESIAN_POINT('Ctrl Pts',(-15.1754010684014,-1.90777756124945,
-0.780122100716514));
#30590=CARTESIAN_POINT('Ctrl Pts',(-15.212414241739,-1.95249892522313,-0.135445245834147));
#30591=CARTESIAN_POINT('Ctrl Pts',(-15.2149862637846,-1.95560658456919,
-0.0906470582287079));
#30592=CARTESIAN_POINT('Ctrl Pts',(-15.2175582858302,-1.95702029228147,
-0.045731360855399));
#30593=CARTESIAN_POINT('Ctrl Pts',(-15.2201303078758,-1.95678697592279,
-0.000800724488720095));
#30594=CARTESIAN_POINT('Ctrl Pts',(-15.3218696921242,-1.95690589693301,
-0.000674027605478421));
#30595=CARTESIAN_POINT('Ctrl Pts',(-15.3197327012511,-1.95707296268264,
-0.0379990733749708));
#30596=CARTESIAN_POINT('Ctrl Pts',(-15.3175957103781,-1.95609737832443,
-0.0753152146046056));
#30597=CARTESIAN_POINT('Ctrl Pts',(-15.315458719505,-1.95395154045615,-0.112563939451326));
#30598=CARTESIAN_POINT('Ctrl Pts',(-15.2784455461674,-1.91678513512746,
-0.75772041939657));
#30599=CARTESIAN_POINT('Ctrl Pts',(-15.2414323728298,-1.52855395128338,
-1.38265263397289));
#30600=CARTESIAN_POINT('Ctrl Pts',(-15.2044191994923,-0.96664627044783,
-1.70182027568869));
#30601=CARTESIAN_POINT('Ctrl Pts',(-15.1674060261547,-0.404738589612277,
-2.0209879174045));
#30602=CARTESIAN_POINT('Ctrl Pts',(-15.1303928528172,0.330845588214744,
-2.03439098625978));
#30603=CARTESIAN_POINT('Ctrl Pts',(-15.0933796794796,0.904007519163827,
-1.73590543181679));
#30604=CARTESIAN_POINT('Ctrl Pts',(-15.056366506142,1.4771694501129,-1.43741987737381));
#30605=CARTESIAN_POINT('Ctrl Pts',(-15.0193533328045,1.88790913418403,-0.827045699632558));
#30606=CARTESIAN_POINT('Ctrl Pts',(-14.9823401594669,1.94855383991442,-0.183671434552528));
#30607=CARTESIAN_POINT('Ctrl Pts',(-14.9453269861293,2.0091985456448,0.459702830527515));
#30608=CARTESIAN_POINT('Ctrl Pts',(-14.9083138127918,1.71974827303444,1.13607718294633));
#30609=CARTESIAN_POINT('Ctrl Pts',(-14.8713006394542,1.21245691765294,1.53640667980563));
#30610=CARTESIAN_POINT('Ctrl Pts',(-14.8342874661166,0.705165562271449,
1.93673617666491));
#30611=CARTESIAN_POINT('Ctrl Pts',(-14.7972742927791,-0.0199668758811834,
2.06102081796467));
#30612=CARTESIAN_POINT('Ctrl Pts',(-14.7602611194415,-0.631617199612173,
1.85247320522319));
#30613=CARTESIAN_POINT('Ctrl Pts',(-14.7232479461039,-1.24326752334318,
1.64392559248171));
#30614=CARTESIAN_POINT('Ctrl Pts',(-14.6862347727664,-1.74143573265255,
1.10254572569898));
#30615=CARTESIAN_POINT('Ctrl Pts',(-14.6492215994288,-1.89850177475563,
0.475697670969221));
#30616=CARTESIAN_POINT('Ctrl Pts',(-14.640104296994,-1.93719120554397,0.321288773262618));
#30617=CARTESIAN_POINT('Ctrl Pts',(-14.6309869945591,-1.95518377170558,
0.161693970317362));
#30618=CARTESIAN_POINT('Ctrl Pts',(-14.6218696921242,-1.95373627769492,
0.00177775396232179));
#30619=CARTESIAN_POINT('Origin',(-9.8,0.,0.));
#30620=CARTESIAN_POINT('',(-13.8201303078758,-1.95088537187799,-0.000408160563786925));
#30621=CARTESIAN_POINT('',(-13.9218696921242,-1.95094021917743,-0.000529095196661905));
#30622=CARTESIAN_POINT('',(-9.8,-1.954,-2.39295984553393E-16));
#30623=CARTESIAN_POINT('Ctrl Pts',(-13.8201303078758,-1.95088537187799,
-0.000408160563786925));
#30624=CARTESIAN_POINT('Ctrl Pts',(-13.8400668724461,-1.95022879632092,
0.350567026998221));
#30625=CARTESIAN_POINT('Ctrl Pts',(-13.8600034370163,-1.85987981718048,
0.701857479589949));
#30626=CARTESIAN_POINT('Ctrl Pts',(-13.8799400015866,-1.68186073672999,
1.00097049400201));
#30627=CARTESIAN_POINT('Ctrl Pts',(-13.9169531749242,-1.35135990952491,
1.55628792649757));
#30628=CARTESIAN_POINT('Ctrl Pts',(-13.9539663482618,-0.718680622512158,
1.93176185852677));
#30629=CARTESIAN_POINT('Ctrl Pts',(-13.9909795215993,-0.0729029294054372,
1.95583297612569));
#30630=CARTESIAN_POINT('Ctrl Pts',(-14.0279926949369,0.572874763701284,
1.97990409372461));
#30631=CARTESIAN_POINT('Ctrl Pts',(-14.0650058682745,1.23175086290198,1.65257239689324));
#30632=CARTESIAN_POINT('Ctrl Pts',(-14.102019041612,1.60267562299808,1.12340033606203));
#30633=CARTESIAN_POINT('Ctrl Pts',(-14.1390322149496,1.97360038309417,0.594228275230817));
#30634=CARTESIAN_POINT('Ctrl Pts',(-14.1760453882871,2.05657380408567,-0.136784149600244));
#30635=CARTESIAN_POINT('Ctrl Pts',(-14.2130585616247,1.81368416436353,-0.735627092726691));
#30636=CARTESIAN_POINT('Ctrl Pts',(-14.2500717349623,1.57079452464139,-1.33447003585314));
#30637=CARTESIAN_POINT('Ctrl Pts',(-14.2870849082998,1.00204182420563,-1.80114349727497));
#30638=CARTESIAN_POINT('Ctrl Pts',(-14.3240980816374,0.367297161362722,
-1.9224178169356));
#30639=CARTESIAN_POINT('Ctrl Pts',(-14.361111254975,-0.267447501480182,
-2.04369213659623));
#30640=CARTESIAN_POINT('Ctrl Pts',(-14.3981244283125,-0.968184126730219,
-1.81956731449565));
#30641=CARTESIAN_POINT('Ctrl Pts',(-14.4351376016501,-1.41473630680673,
-1.35244913021504));
#30642=CARTESIAN_POINT('Ctrl Pts',(-14.4634685037253,-1.75653964179354,
-0.994904009300521));
#30643=CARTESIAN_POINT('Ctrl Pts',(-14.4917994058005,-1.94942156861746,
-0.494994104241234));
#30644=CARTESIAN_POINT('Ctrl Pts',(-14.5201303078758,-1.95396550297987,
0.00177712178281789));
#30645=CARTESIAN_POINT('Ctrl Pts',(-14.6218696921242,-1.95373627769492,
0.00177775396232179));
#30646=CARTESIAN_POINT('Ctrl Pts',(-14.5939738212215,-1.94930743414802,
-0.487511940940269));
#30647=CARTESIAN_POINT('Ctrl Pts',(-14.5660779503188,-1.76288976123999,
-0.979810559152193));
#30648=CARTESIAN_POINT('Ctrl Pts',(-14.5381820794161,-1.43048209022845,
-1.3357837596151));
#30649=CARTESIAN_POINT('Ctrl Pts',(-14.5011689060785,-0.989432488701429,
-1.80810089279285));
#30650=CARTESIAN_POINT('Ctrl Pts',(-14.464155732741,-0.291369410750597,
-2.04041891647158));
#30651=CARTESIAN_POINT('Ctrl Pts',(-14.4271425594034,0.34475231736069,-1.92658846217614));
#30652=CARTESIAN_POINT('Ctrl Pts',(-14.3901293860659,0.980874045471991,
-1.8127580078807));
#30653=CARTESIAN_POINT('Ctrl Pts',(-14.3531162127283,1.55505442374375,-1.3527790756111));
#30654=CARTESIAN_POINT('Ctrl Pts',(-14.3161030393907,1.80494237162162,-0.756822501013755));
#30655=CARTESIAN_POINT('Ctrl Pts',(-14.2790898660532,2.0548303194995,-0.160865926416412));
#30656=CARTESIAN_POINT('Ctrl Pts',(-14.2420766927156,1.98042583698348,0.571068290508656));
#30657=CARTESIAN_POINT('Ctrl Pts',(-14.205063519378,1.61572537732216,1.10454912430049));
#30658=CARTESIAN_POINT('Ctrl Pts',(-14.1680503460405,1.25102491766083,1.63802995809231));
#30659=CARTESIAN_POINT('Ctrl Pts',(-14.1310371727029,0.596028480854202,
1.9730574087509));
#30660=CARTESIAN_POINT('Ctrl Pts',(-14.0940239993653,-0.0499868601460479,
1.9565527278171));
#30661=CARTESIAN_POINT('Ctrl Pts',(-14.0570108260278,-0.696002201146311,
1.9400480468833));
#30662=CARTESIAN_POINT('Ctrl Pts',(-14.0199976526902,-1.33303644634019,
1.57201123435709));
#30663=CARTESIAN_POINT('Ctrl Pts',(-13.9829844793526,-1.67001970044536,
1.02060347982955));
#30664=CARTESIAN_POINT('Ctrl Pts',(-13.9626128836098,-1.85549114225117,
0.717115428096236));
#30665=CARTESIAN_POINT('Ctrl Pts',(-13.942241287867,-1.95006914783739,0.358079434458608));
#30666=CARTESIAN_POINT('Ctrl Pts',(-13.9218696921242,-1.95094021917743,
-0.000529095196661905));
#30667=CARTESIAN_POINT('Origin',(-9.8,0.,0.));
#30668=CARTESIAN_POINT('',(-13.1201303078758,-1.95545730741116,-0.00153438558903124));
#30669=CARTESIAN_POINT('',(-13.2218696921242,-1.95566871115984,-0.00146207300122905));
#30670=CARTESIAN_POINT('',(-9.8,-1.954,-2.39295984553393E-16));
#30671=CARTESIAN_POINT('Ctrl Pts',(-13.1201303078758,-1.95545730741116,
-0.00153438558903124));
#30672=CARTESIAN_POINT('Ctrl Pts',(-13.151321165754,-1.95075080529458,0.544310729119318));
#30673=CARTESIAN_POINT('Ctrl Pts',(-13.1825120236322,-1.7119678003024,1.09376537173191));
#30674=CARTESIAN_POINT('Ctrl Pts',(-13.2137028815105,-1.30649016387798,
1.45728546253184));
#30675=CARTESIAN_POINT('Ctrl Pts',(-13.250716054848,-0.825323082803425,
1.88866289321973));
#30676=CARTESIAN_POINT('Ctrl Pts',(-13.2877292281856,-0.109420047168152,
2.05821110882994));
#30677=CARTESIAN_POINT('Ctrl Pts',(-13.3247424015232,0.514112789494058,
1.88846114794432));
#30678=CARTESIAN_POINT('Ctrl Pts',(-13.3617555748607,1.13764562615628,1.71871118705871));
#30679=CARTESIAN_POINT('Ctrl Pts',(-13.3987687481983,1.66880826384543,1.20966304967725));
#30680=CARTESIAN_POINT('Ctrl Pts',(-13.4357819215359,1.86490503196531,0.593907980555089));
#30681=CARTESIAN_POINT('Ctrl Pts',(-13.4727950948734,2.06100180008519,-0.02184708856707));
#30682=CARTESIAN_POINT('Ctrl Pts',(-13.509808268211,1.9220326986358,-0.744309089429943));
#30683=CARTESIAN_POINT('Ctrl Pts',(-13.5468214415486,1.51149466221922,-1.24337498515105));
#30684=CARTESIAN_POINT('Ctrl Pts',(-13.5838346148861,1.10095662580263,-1.74244088087216));
#30685=CARTESIAN_POINT('Ctrl Pts',(-13.6208477882237,0.418849654418843,
-2.01811067145151));
#30686=CARTESIAN_POINT('Ctrl Pts',(-13.6578609615612,-0.223161994900548,
-1.94442695713893));
#30687=CARTESIAN_POINT('Ctrl Pts',(-13.6948741348988,-0.86517364421993,
-1.87074324282635));
#30688=CARTESIAN_POINT('Ctrl Pts',(-13.7318873082364,-1.46708997147491,
-1.44770602362185));
#30689=CARTESIAN_POINT('Ctrl Pts',(-13.7689004815739,-1.7538869514037,-0.868606947538646));
#30690=CARTESIAN_POINT('Ctrl Pts',(-13.7859770903412,-1.88620524190027,
-0.601430494723484));
#30691=CARTESIAN_POINT('Ctrl Pts',(-13.8030536991085,-1.95144775983979,
-0.301034978383196));
#30692=CARTESIAN_POINT('Ctrl Pts',(-13.8201303078758,-1.95088537187799,
-0.000408160563786925));
#30693=CARTESIAN_POINT('Ctrl Pts',(-13.9218696921242,-1.95094021917743,
-0.000529095196661905));
#30694=CARTESIAN_POINT('Ctrl Pts',(-13.9052281145295,-1.95165179825443,
-0.29347677331393));
#30695=CARTESIAN_POINT('Ctrl Pts',(-13.8885865369347,-1.88983018220934,
-0.586139193047371));
#30696=CARTESIAN_POINT('Ctrl Pts',(-13.87194495934,-1.76394161972146,-0.848001901607685));
#30697=CARTESIAN_POINT('Ctrl Pts',(-13.8349317860024,-1.48394802187595,
-1.43042083198849));
#30698=CARTESIAN_POINT('Ctrl Pts',(-13.7979186126648,-0.887028563168493,
-1.86047999622125));
#30699=CARTESIAN_POINT('Ctrl Pts',(-13.7609054393273,-0.245924129428696,
-1.94167932096949));
#30700=CARTESIAN_POINT('Ctrl Pts',(-13.7238922659897,0.395180304311114,
-2.02287864571773));
#30701=CARTESIAN_POINT('Ctrl Pts',(-13.6868790926521,1.08046971308327,-1.75521813098144));
#30702=CARTESIAN_POINT('Ctrl Pts',(-13.6498659193146,1.49682573950857,-1.26099562586887));
#30703=CARTESIAN_POINT('Ctrl Pts',(-13.612852745977,1.91318176593387,-0.766773120756301));
#30704=CARTESIAN_POINT('Ctrl Pts',(-13.5758395726394,2.06060441001232,-0.04598862526747));
#30705=CARTESIAN_POINT('Ctrl Pts',(-13.5388263993019,1.87173419476462,0.57202129948511));
#30706=CARTESIAN_POINT('Ctrl Pts',(-13.5018132259643,1.68286397951692,1.1900312242377));
#30707=CARTESIAN_POINT('Ctrl Pts',(-13.4648000526268,1.15770090494307,1.70526657825403));
#30708=CARTESIAN_POINT('Ctrl Pts',(-13.4277868792892,0.536199356973832,
1.8823090905844));
#30709=CARTESIAN_POINT('Ctrl Pts',(-13.3907737059516,-0.085302190995406,
2.05935160291476));
#30710=CARTESIAN_POINT('Ctrl Pts',(-13.3537605326141,-0.803142212360044,
1.89820127355916));
#30711=CARTESIAN_POINT('Ctrl Pts',(-13.3167473592765,-1.28932951759698,
1.47248995173785));
#30712=CARTESIAN_POINT('Ctrl Pts',(-13.2851214702257,-1.70475203846754,
1.10874110727149));
#30713=CARTESIAN_POINT('Ctrl Pts',(-13.253495581175,-1.95104861266841,0.55184050939348));
#30714=CARTESIAN_POINT('Ctrl Pts',(-13.2218696921242,-1.95566871115984,
-0.00146207300122905));
#30715=CARTESIAN_POINT('Origin',(-9.8,0.,0.));
#30716=CARTESIAN_POINT('',(-12.4201303078758,-1.95564737559935,0.00146991064532538));
#30717=CARTESIAN_POINT('',(-12.5218696921242,-1.95543514278731,0.00154130734549634));
#30718=CARTESIAN_POINT('',(-9.8,-1.954,-2.39295984553393E-16));
#30719=CARTESIAN_POINT('Ctrl Pts',(-12.4201303078758,-1.95564737559935,
0.00146991064532538));
#30720=CARTESIAN_POINT('Ctrl Pts',(-12.4255622857244,-1.95644383279381,
0.0965063867288474));
#30721=CARTESIAN_POINT('Ctrl Pts',(-12.430994263573,-1.95011384225001,0.191436345000714));
#30722=CARTESIAN_POINT('Ctrl Pts',(-12.4364262414216,-1.93629099486106,
0.285262424508588));
#30723=CARTESIAN_POINT('Ctrl Pts',(-12.4734394147592,-1.84210293653611,
0.924587738637213));
#30724=CARTESIAN_POINT('Ctrl Pts',(-12.5104525880968,-1.40002315460498,
1.51266020037653));
#30725=CARTESIAN_POINT('Ctrl Pts',(-12.5474657614343,-0.812044111488547,
1.78078124108868));
#30726=CARTESIAN_POINT('Ctrl Pts',(-12.5844789347719,-0.2240650683721,2.04890228180084));
#30727=CARTESIAN_POINT('Ctrl Pts',(-12.6214921081094,0.50981323592966,1.99707190148582));
#30728=CARTESIAN_POINT('Ctrl Pts',(-12.658505281447,1.05427149512405,1.64897212898989));
#30729=CARTESIAN_POINT('Ctrl Pts',(-12.6955184547846,1.59872975431843,1.30087235649397));
#30730=CARTESIAN_POINT('Ctrl Pts',(-12.7325316281221,1.95376796840545,0.656503191817144));
#30731=CARTESIAN_POINT('Ctrl Pts',(-12.7695448014597,1.95716419001697,0.010285957989807));
#30732=CARTESIAN_POINT('Ctrl Pts',(-12.8065579747973,1.9605604116285,-0.635931275837539));
#30733=CARTESIAN_POINT('Ctrl Pts',(-12.8435711481348,1.61231464076452,-1.28399657881539));
#30734=CARTESIAN_POINT('Ctrl Pts',(-12.8805843214724,1.07154526206863,-1.63779981040261));
#30735=CARTESIAN_POINT('Ctrl Pts',(-12.91759749481,0.530775883372733,-1.99160304198983));
#30736=CARTESIAN_POINT('Ctrl Pts',(-12.9546106681475,-0.202517103155076,
-2.05114420218641));
#30737=CARTESIAN_POINT('Ctrl Pts',(-12.9916238414851,-0.793281831135205,
-1.78921809850206));
#30738=CARTESIAN_POINT('Ctrl Pts',(-13.0286370148227,-1.38404655911533,
-1.52729199481771));
#30739=CARTESIAN_POINT('Ctrl Pts',(-13.0656501881602,-1.83228302854778,
-0.943898627252431));
#30740=CARTESIAN_POINT('Ctrl Pts',(-13.1026633614978,-1.93318570000708,
-0.305598620587008));
#30741=CARTESIAN_POINT('Ctrl Pts',(-13.1084856769571,-1.94905808086367,
-0.205191558414774));
#30742=CARTESIAN_POINT('Ctrl Pts',(-13.1143079924164,-1.95633585779087,
-0.103425858474165));
#30743=CARTESIAN_POINT('Ctrl Pts',(-13.1201303078758,-1.95545730741116,
-0.00153438558903124));
#30744=CARTESIAN_POINT('Ctrl Pts',(-13.2218696921242,-1.95566871115984,
-0.00146207300122905));
#30745=CARTESIAN_POINT('Ctrl Pts',(-13.2164824078374,-1.95645571777858,
-0.0957139153194285));
#30746=CARTESIAN_POINT('Ctrl Pts',(-13.2110951235506,-1.95022996916634,
-0.189861353591568));
#30747=CARTESIAN_POINT('Ctrl Pts',(-13.2057078392638,-1.93663285562017,
-0.282931874217572));
#30748=CARTESIAN_POINT('Ctrl Pts',(-13.1686946659262,-1.84321429929716,
-0.922370064064672));
#30749=CARTESIAN_POINT('Ctrl Pts',(-13.1316814925887,-1.4018425975419,-1.51097412947185));
#30750=CARTESIAN_POINT('Ctrl Pts',(-13.0946683192511,-0.814186680996224,
-1.77980260461776));
#30751=CARTESIAN_POINT('Ctrl Pts',(-13.0576551459135,-0.226530764450553,
-2.04863107976367));
#30752=CARTESIAN_POINT('Ctrl Pts',(-13.020641972576,0.507409366885524,-1.99768396464832));
#30753=CARTESIAN_POINT('Ctrl Pts',(-12.9836287992384,1.05228615707883,-1.6502397118407));
#30754=CARTESIAN_POINT('Ctrl Pts',(-12.9466156259009,1.59716294727213,-1.30279545903307));
#30755=CARTESIAN_POINT('Ctrl Pts',(-12.9096024525633,1.95297639632267,-0.658854068533187));
#30756=CARTESIAN_POINT('Ctrl Pts',(-12.8725892792257,1.95715034111747,-0.0126414073408709));
#30757=CARTESIAN_POINT('Ctrl Pts',(-12.8355761058882,1.96132428591228,0.633571253851449));
#30758=CARTESIAN_POINT('Ctrl Pts',(-12.7985629325506,1.61385872645134,1.28205518573619));
#30759=CARTESIAN_POINT('Ctrl Pts',(-12.761549759213,1.07351555782829,1.63650897034401));
#30760=CARTESIAN_POINT('Ctrl Pts',(-12.7245365858755,0.533172389205236,
1.99096275495183));
#30761=CARTESIAN_POINT('Ctrl Pts',(-12.6875234125379,-0.20004838857994,
2.05138639228274));
#30762=CARTESIAN_POINT('Ctrl Pts',(-12.6505102392003,-0.791127902336491,
1.79017147364728));
#30763=CARTESIAN_POINT('Ctrl Pts',(-12.6134970658628,-1.38220741609303,
1.52895655501182));
#30764=CARTESIAN_POINT('Ctrl Pts',(-12.5764838925252,-1.83114566582096,
0.946103080410012));
#30765=CARTESIAN_POINT('Ctrl Pts',(-12.5394707191876,-1.93281645881963,
0.307924989943551));
#30766=CARTESIAN_POINT('Ctrl Pts',(-12.5336037101665,-1.94893243607642,
0.206766502944533));
#30767=CARTESIAN_POINT('Ctrl Pts',(-12.5277367011454,-1.95632302115412,
0.104217937603238));
#30768=CARTESIAN_POINT('Ctrl Pts',(-12.5218696921242,-1.95543514278731,
0.00154130734549634));
#30769=CARTESIAN_POINT('Origin',(-9.8,0.,0.));
#30770=CARTESIAN_POINT('',(-11.7201303078758,-1.95093397599971,0.000516778435547954));
#30771=CARTESIAN_POINT('',(-11.8218696921242,-1.95088048851305,0.000395614960693866));
#30772=CARTESIAN_POINT('',(-9.8,-1.954,-2.39295984553393E-16));
#30773=CARTESIAN_POINT('Ctrl Pts',(-11.7201303078758,-1.95093397599971,
0.000516778435547954));
#30774=CARTESIAN_POINT('Ctrl Pts',(-11.7368165790323,-1.9516307292599,0.294253588167556));
#30775=CARTESIAN_POINT('Ctrl Pts',(-11.7535028501889,-1.88946238212134,
0.587710338684493));
#30776=CARTESIAN_POINT('Ctrl Pts',(-11.7701891213455,-1.76291981471983,
0.850124222972598));
#30777=CARTESIAN_POINT('Ctrl Pts',(-11.807202294683,-1.48222546798021,1.43220577338039));
#30778=CARTESIAN_POINT('Ctrl Pts',(-11.8442154680206,-0.884788847197,1.86154624200128));
#30779=CARTESIAN_POINT('Ctrl Pts',(-11.8812286413582,-0.243587136816991,
1.94197393761962));
#30780=CARTESIAN_POINT('Ctrl Pts',(-11.9182418146957,0.397614573562981,
2.02240163323796));
#30781=CARTESIAN_POINT('Ctrl Pts',(-11.9552549880333,1.08258137353975,1.75391655585379));
#30782=CARTESIAN_POINT('Ctrl Pts',(-11.9922681613709,1.49834231022453,1.25919330883212));
#30783=CARTESIAN_POINT('Ctrl Pts',(-12.0292813347084,1.91410324690933,0.764470061810429));
#30784=CARTESIAN_POINT('Ctrl Pts',(-12.066294508046,2.06065832030212,0.0435086451512185));
#30785=CARTESIAN_POINT('Ctrl Pts',(-12.1033076813835,1.87104445865698,-0.574273542264962));
#30786=CARTESIAN_POINT('Ctrl Pts',(-12.1403208547211,1.68143059701185,-1.19205572968113));
#30787=CARTESIAN_POINT('Ctrl Pts',(-12.1773340280587,1.15564780032879,-1.70665868785428));
#30788=CARTESIAN_POINT('Ctrl Pts',(-12.2143472013962,0.533933614275722,
-1.88295309637894));
#30789=CARTESIAN_POINT('Ctrl Pts',(-12.2513603747338,-0.0877805717773474,
-2.0592475049036));
#30790=CARTESIAN_POINT('Ctrl Pts',(-12.2883735480714,-0.805426147200425,
-1.89723336377978));
#30791=CARTESIAN_POINT('Ctrl Pts',(-12.3253867214089,-1.29110076755259,
-1.4709372099589));
#30792=CARTESIAN_POINT('Ctrl Pts',(-12.3569679168979,-1.70549877091952,
-1.10720341044869));
#30793=CARTESIAN_POINT('Ctrl Pts',(-12.3885491123868,-1.95101682093624,
-0.551066497531743));
#30794=CARTESIAN_POINT('Ctrl Pts',(-12.4201303078758,-1.95564737559935,
0.00146991064532538));
#30795=CARTESIAN_POINT('Ctrl Pts',(-12.5218696921242,-1.95543514278731,
0.00154130734549634));
#30796=CARTESIAN_POINT('Ctrl Pts',(-12.4907235278078,-1.95072166690785,
-0.543537656389124));
#30797=CARTESIAN_POINT('Ctrl Pts',(-12.4595773634914,-1.71270248299415,
-1.09222577733106));
#30798=CARTESIAN_POINT('Ctrl Pts',(-12.428431199175,-1.30824303327262,-1.45571200064073));
#30799=CARTESIAN_POINT('Ctrl Pts',(-12.3914180258374,-0.827595478457534,
-1.88766819442741));
#30800=CARTESIAN_POINT('Ctrl Pts',(-12.3544048524998,-0.111897032557945,
-2.05807787566966));
#30801=CARTESIAN_POINT('Ctrl Pts',(-12.3173916791623,0.511839630816549,
-1.88907846720071));
#30802=CARTESIAN_POINT('Ctrl Pts',(-12.2803785058247,1.13557629419105,-1.72007905873176));
#30803=CARTESIAN_POINT('Ctrl Pts',(-12.2433653324871,1.66735117504045,-1.21167056055161));
#30804=CARTESIAN_POINT('Ctrl Pts',(-12.2063521591496,1.86418886026822,-0.596151957279062));
#30805=CARTESIAN_POINT('Ctrl Pts',(-12.169338985812,2.061026545496,0.0193666459934833));
#30806=CARTESIAN_POINT('Ctrl Pts',(-12.1323258124744,1.92292703510214,0.741995354358439));
#30807=CARTESIAN_POINT('Ctrl Pts',(-12.0953126391369,1.51298993531999,1.2415549599338));
#30808=CARTESIAN_POINT('Ctrl Pts',(-12.0582994657993,1.10305283553785,1.74111456550915));
#30809=CARTESIAN_POINT('Ctrl Pts',(-12.0212862924617,0.421278146367432,
2.01760506829494));
#30810=CARTESIAN_POINT('Ctrl Pts',(-11.9842731191242,-0.220821699570658,
1.94469407360503));
#30811=CARTESIAN_POINT('Ctrl Pts',(-11.9472599457866,-0.862921545508766,
1.87178307891512));
#30812=CARTESIAN_POINT('Ctrl Pts',(-11.9102467724491,-1.46534654821454,
1.4494705867495));
#30813=CARTESIAN_POINT('Ctrl Pts',(-11.8732335991115,-1.75284026146716,
0.870717107156824));
#30814=CARTESIAN_POINT('Ctrl Pts',(-11.8561122967824,-1.8858271506868,0.603001253459379));
#30815=CARTESIAN_POINT('Ctrl Pts',(-11.8389909944533,-1.95142694075535,
0.30181110017949));
#30816=CARTESIAN_POINT('Ctrl Pts',(-11.8218696921242,-1.95088048851305,
0.000395614960693866));
#30817=CARTESIAN_POINT('Origin',(-9.8,0.,0.));
#30818=CARTESIAN_POINT('',(-11.0201303078758,-1.95375977033508,-0.00177812828496077));
#30819=CARTESIAN_POINT('',(-11.1218696921242,-1.95398910254737,-0.00177651513874471));
#30820=CARTESIAN_POINT('',(-9.8,-1.954,-2.39295984553393E-16));
#30821=CARTESIAN_POINT('Ctrl Pts',(-11.0201303078758,-1.95375977033508,
-0.00177812828496077));
#30822=CARTESIAN_POINT('Ctrl Pts',(-11.0480708723403,-1.94931821586781,
0.488280492828455));
#30823=CARTESIAN_POINT('Ctrl Pts',(-11.0760114368048,-1.762242579831,0.981361839095669));
#30824=CARTESIAN_POINT('Ctrl Pts',(-11.1039520012693,-1.42887346982972,
1.33750442049114));
#30825=CARTESIAN_POINT('Ctrl Pts',(-11.1409651746069,-0.987255739825101,
1.8092904187597));
#30826=CARTESIAN_POINT('Ctrl Pts',(-11.1779783479444,-0.288913552828485,
2.04076815788204));
#30827=CARTESIAN_POINT('Ctrl Pts',(-11.214991521282,0.347070736053018,1.92617220720064));
#30828=CARTESIAN_POINT('Ctrl Pts',(-11.2520046946196,0.983055024934531,
1.81157625651923));
#30829=CARTESIAN_POINT('Ctrl Pts',(-11.2890178679571,1.55668141570094,1.35090661603405));
#30830=CARTESIAN_POINT('Ctrl Pts',(-11.3260310412947,1.80585195247114,0.754649715677886));
#30831=CARTESIAN_POINT('Ctrl Pts',(-11.3630442146323,2.05502248924135,0.158392815321727));
#30832=CARTESIAN_POINT('Ctrl Pts',(-11.4000573879698,1.97973717201537,-0.573451344905431));
#30833=CARTESIAN_POINT('Ctrl Pts',(-11.4370705613074,1.61439491979416,-1.10649288771296));
#30834=CARTESIAN_POINT('Ctrl Pts',(-11.474083734645,1.24905266757295,-1.6395344305205));
#30835=CARTESIAN_POINT('Ctrl Pts',(-11.5110969079825,0.59365348035652,-1.97377335590839));
#30836=CARTESIAN_POINT('Ctrl Pts',(-11.5481100813201,-0.0523415465836445,
-1.95649120369037));
#30837=CARTESIAN_POINT('Ctrl Pts',(-11.5851232546576,-0.698336573523782,
-1.93920905147235));
#30838=CARTESIAN_POINT('Ctrl Pts',(-11.6221364279952,-1.33492744018764,
-1.57040582164844));
#30839=CARTESIAN_POINT('Ctrl Pts',(-11.6591496013328,-1.67124683717155,
-1.01859289063916));
#30840=CARTESIAN_POINT('Ctrl Pts',(-11.6794765035138,-1.85594679309579,
-0.71554815117469));
#30841=CARTESIAN_POINT('Ctrl Pts',(-11.6998034056948,-1.95008520426206,
-0.357307887264606));
#30842=CARTESIAN_POINT('Ctrl Pts',(-11.7201303078758,-1.95093397599971,
0.000516778435547954));
#30843=CARTESIAN_POINT('Ctrl Pts',(-11.8218696921242,-1.95088048851305,
0.000395614960693866));
#30844=CARTESIAN_POINT('Ctrl Pts',(-11.8019778211157,-1.95024560938371,
-0.34979491591636));
#30845=CARTESIAN_POINT('Ctrl Pts',(-11.7820859501073,-1.86032483576546,
-0.700289605624201));
#30846=CARTESIAN_POINT('Ctrl Pts',(-11.7621940790988,-1.68306414685726,
-0.998945614375208));
#30847=CARTESIAN_POINT('Ctrl Pts',(-11.7251809057612,-1.35323189519527,
-1.55466038929485));
#30848=CARTESIAN_POINT('Ctrl Pts',(-11.6881677324237,-0.721004968071823,
-1.93089547211442));
#30849=CARTESIAN_POINT('Ctrl Pts',(-11.6511545590861,-0.0752567296127299,
-1.95574376838169));
#30850=CARTESIAN_POINT('Ctrl Pts',(-11.6141413857485,0.570491508846364,
-1.98059206464896));
#30851=CARTESIAN_POINT('Ctrl Pts',(-11.577128212411,1.22976105864111,-1.65405357436393));
#30852=CARTESIAN_POINT('Ctrl Pts',(-11.5401150390734,1.60132240146957,-1.12532832074356));
#30853=CARTESIAN_POINT('Ctrl Pts',(-11.5031018657358,1.97288374429803,-0.596603067123194));
#30854=CARTESIAN_POINT('Ctrl Pts',(-11.4660886923983,2.0567368801602,0.134308949832498));
#30855=CARTESIAN_POINT('Ctrl Pts',(-11.4290755190607,1.81456813336496,0.733443762187807));
#30856=CARTESIAN_POINT('Ctrl Pts',(-11.3920623457231,1.57239938656973,1.33257857454311));
#30857=CARTESIAN_POINT('Ctrl Pts',(-11.3550491723856,1.00420875711708,1.79993618229802));
#30858=CARTESIAN_POINT('Ctrl Pts',(-11.318035999048,0.369610525185732,1.9219743293259));
#30859=CARTESIAN_POINT('Ctrl Pts',(-11.2810228257105,-0.264987706745639,
2.04401247635378));
#30860=CARTESIAN_POINT('Ctrl Pts',(-11.2440096523729,-0.965993541155731,
1.82073116265462));
#30861=CARTESIAN_POINT('Ctrl Pts',(-11.2069964790353,-1.41310756501697,
1.35415075697192));
#30862=CARTESIAN_POINT('Ctrl Pts',(-11.1786208833983,-1.75588084276393,
0.996453868810782));
#30863=CARTESIAN_POINT('Ctrl Pts',(-11.1502452877613,-1.94943446818612,
0.495762979235285));
#30864=CARTESIAN_POINT('Ctrl Pts',(-11.1218696921242,-1.95398910254737,
-0.00177651513874471));
#30865=CARTESIAN_POINT('Origin',(-9.8,0.,0.));
#30866=CARTESIAN_POINT('',(-10.3201303078758,-1.9568945579723,0.000687273504990336));
#30867=CARTESIAN_POINT('',(-10.4218696921242,-1.95677370715668,0.000813444693687295));
#30868=CARTESIAN_POINT('',(-9.8,-1.954,-2.39295984553393E-16));
#30869=CARTESIAN_POINT('Ctrl Pts',(-10.3201303078758,-1.9568945579723,0.000687273504990337));
#30870=CARTESIAN_POINT('Ctrl Pts',(-10.3223119923107,-1.95706803944366,
0.0387935361464464));
#30871=CARTESIAN_POINT('Ctrl Pts',(-10.3244936767456,-1.95605118783441,
0.0768903607640225));
#30872=CARTESIAN_POINT('Ctrl Pts',(-10.3266753611805,-1.95381470630591,
0.114915451699472));
#30873=CARTESIAN_POINT('Ctrl Pts',(-10.363688534518,-1.91587187774813,0.760026751691749));
#30874=CARTESIAN_POINT('Ctrl Pts',(-10.4007017078556,-1.52688885554805,
1.38449129214901));
#30875=CARTESIAN_POINT('Ctrl Pts',(-10.4377148811932,-0.964597446735795,
1.70298245245432));
#30876=CARTESIAN_POINT('Ctrl Pts',(-10.4747280545307,-0.402306037923545,
2.02147361275964));
#30877=CARTESIAN_POINT('Ctrl Pts',(-10.5117412278683,0.333293757500867,
2.03399139291301));
#30878=CARTESIAN_POINT('Ctrl Pts',(-10.5487544012059,0.906096059768414,
1.73481624332052));
#30879=CARTESIAN_POINT('Ctrl Pts',(-10.5857675745434,1.47889836203597,1.43564109372802));
#30880=CARTESIAN_POINT('Ctrl Pts',(-10.622780747881,1.88890317114665,0.824773014389662));
#30881=CARTESIAN_POINT('Ctrl Pts',(-10.6597939212185,1.94877353033013,0.181326211842671));
#30882=CARTESIAN_POINT('Ctrl Pts',(-10.6968070945561,2.00864388951361,-0.462120590704301));
#30883=CARTESIAN_POINT('Ctrl Pts',(-10.7338202678937,1.71837979876989,-1.13814611645991));
#30884=CARTESIAN_POINT('Ctrl Pts',(-10.7708334412312,1.21060699860575,-1.53786480632835));
#30885=CARTESIAN_POINT('Ctrl Pts',(-10.8078466145688,0.702834198441578,
-1.93758349619681));
#30886=CARTESIAN_POINT('Ctrl Pts',(-10.8448597879064,-0.0224473111430409,
-2.06099535017809));
#30887=CARTESIAN_POINT('Ctrl Pts',(-10.8818729612439,-0.63384622012401,
-1.85171175857666));
#30888=CARTESIAN_POINT('Ctrl Pts',(-10.9188861345815,-1.24524512910496,
-1.64242816697523));
#30889=CARTESIAN_POINT('Ctrl Pts',(-10.9558993079191,-1.74276143748226,
-1.10044912979111));
#30890=CARTESIAN_POINT('Ctrl Pts',(-10.9929124812566,-1.89907295516461,
-0.473412482491661));
#30891=CARTESIAN_POINT('Ctrl Pts',(-11.0019850901297,-1.93738778025002,
-0.319714278932262));
#30892=CARTESIAN_POINT('Ctrl Pts',(-11.0110576990027,-1.95520199196668,
-0.160905557506181));
#30893=CARTESIAN_POINT('Ctrl Pts',(-11.0201303078758,-1.95375977033508,
-0.00177812828496077));
#30894=CARTESIAN_POINT('Ctrl Pts',(-11.1218696921242,-1.95398910254737,
-0.00177651513874471));
#30895=CARTESIAN_POINT('Ctrl Pts',(-11.1132321144237,-1.95537554069288,
-0.153228350607148));
#30896=CARTESIAN_POINT('Ctrl Pts',(-11.1045945367232,-1.93924926518043,
-0.304388176676578));
#30897=CARTESIAN_POINT('Ctrl Pts',(-11.0959569590226,-1.90448826142854,
-0.45113382160585));
#30898=CARTESIAN_POINT('Ctrl Pts',(-11.0589437856851,-1.75553272066649,
-1.07995849683472));
#30899=CARTESIAN_POINT('Ctrl Pts',(-11.0219306123475,-1.26439942583,-1.62772834962624));
#30900=CARTESIAN_POINT('Ctrl Pts',(-10.9849174390099,-0.655494078459054,
-1.84415963951631));
#30901=CARTESIAN_POINT('Ctrl Pts',(-10.9479042656724,-0.0465887310881076,
-2.06059092940637));
#30902=CARTESIAN_POINT('Ctrl Pts',(-10.9108910923348,0.680088668817298,
-1.94568365639498));
#30903=CARTESIAN_POINT('Ctrl Pts',(-10.8738779189972,1.19250900933691,-1.55194056766556));
#30904=CARTESIAN_POINT('Ctrl Pts',(-10.8368647456597,1.70492934985651,-1.15819747893615));
#30905=CARTESIAN_POINT('Ctrl Pts',(-10.7998515723221,2.00309263099032,-0.485618574488742));
#30906=CARTESIAN_POINT('Ctrl Pts',(-10.7628383989846,1.95076386117954,0.158485396272577));
#30907=CARTESIAN_POINT('Ctrl Pts',(-10.725825225647,1.89843509136877,0.802589367033887));
#30908=CARTESIAN_POINT('Ctrl Pts',(-10.6888120523094,1.4956142706134,1.4182184041091));
#30909=CARTESIAN_POINT('Ctrl Pts',(-10.6517988789719,0.926355890488103,
1.72408295249208));
#30910=CARTESIAN_POINT('Ctrl Pts',(-10.6147857056343,0.357097510362794,
2.02994750087506));
#30911=CARTESIAN_POINT('Ctrl Pts',(-10.5777725322967,-0.378598429132457,
2.02604756056581));
#30912=CARTESIAN_POINT('Ctrl Pts',(-10.5407593589592,-0.944582118652054,
1.7141650690755));
#30913=CARTESIAN_POINT('Ctrl Pts',(-10.5037461856216,-1.51056580817164,
1.40228257758519));
#30914=CARTESIAN_POINT('Ctrl Pts',(-10.466733012284,-1.90683724771558,0.782417534913847));
#30915=CARTESIAN_POINT('Ctrl Pts',(-10.4297198389465,-1.95233444998628,
0.137794986529184));
#30916=CARTESIAN_POINT('Ctrl Pts',(-10.4271031233391,-1.95555095990802,
0.092222188221208));
#30917=CARTESIAN_POINT('Ctrl Pts',(-10.4244864077316,-1.95701428341649,
0.0465256507156762));
#30918=CARTESIAN_POINT('Ctrl Pts',(-10.4218696921242,-1.95677370715668,
0.000813444693687295));
#30919=CARTESIAN_POINT('Origin',(-9.8,0.,0.));
#30920=CARTESIAN_POINT('',(-9.62013030787576,-1.951759122336,0.00130501714239645));
#30921=CARTESIAN_POINT('',(-9.72186969212421,-1.95160825484864,0.00121583516621696));
#30922=CARTESIAN_POINT('',(-9.8,-1.954,-2.39295984553393E-16));
#30923=CARTESIAN_POINT('Ctrl Pts',(-9.62013030787576,-1.951759122336,0.00130501714239645));
#30924=CARTESIAN_POINT('Ctrl Pts',(-9.63356628561861,-1.95321216672716,
0.23757493874278));
#30925=CARTESIAN_POINT('Ctrl Pts',(-9.64700226336145,-1.91351631519969,
0.473373218815082));
#30926=CARTESIAN_POINT('Ctrl Pts',(-9.6604382411043,-1.8304828450213,0.692769818698314));
#30927=CARTESIAN_POINT('Ctrl Pts',(-9.69745141444186,-1.60174383671438,
1.29715935674101));
#30928=CARTESIAN_POINT('Ctrl Pts',(-9.73446458777943,-1.04412356331037,
1.77707954233155));
#30929=CARTESIAN_POINT('Ctrl Pts',(-9.77147776111699,-0.412406560823673,
1.91324810105907));
#30930=CARTESIAN_POINT('Ctrl Pts',(-9.80849093445456,0.21931044166301,2.04941665978659));
#30931=CARTESIAN_POINT('Ctrl Pts',(-9.84550410779212,0.925124173232371,
1.8418335916511));
#30932=CARTESIAN_POINT('Ctrl Pts',(-9.88251728112969,1.38253842510649,1.38534651647905));
#30933=CARTESIAN_POINT('Ctrl Pts',(-9.91953045446725,1.83995267698061,0.928859441306994));
#30934=CARTESIAN_POINT('Ctrl Pts',(-9.95654362780481,2.04896744915949,0.223468359098379));
#30935=CARTESIAN_POINT('Ctrl Pts',(-9.99355680114238,1.91408095612756,-0.408523635798906));
#30936=CARTESIAN_POINT('Ctrl Pts',(-10.0305699744799,1.77919446309564,-1.04051563069619));
#30937=CARTESIAN_POINT('Ctrl Pts',(-10.0675831478175,1.30040670485291,-1.59910853828215));
#30938=CARTESIAN_POINT('Ctrl Pts',(-10.1045963211551,0.696482533847406,
-1.82907341232167));
#30939=CARTESIAN_POINT('Ctrl Pts',(-10.1416094944926,0.0925583628419107,
-2.0590382863612));
#30940=CARTESIAN_POINT('Ctrl Pts',(-10.1786226678302,-0.636502220926357,
-1.96037512685431));
#30941=CARTESIAN_POINT('Ctrl Pts',(-10.2156358411678,-1.15758119535276,
-1.57816451733723));
#30942=CARTESIAN_POINT('Ctrl Pts',(-10.2504673300704,-1.64794597303924,
-1.21848272289988));
#30943=CARTESIAN_POINT('Ctrl Pts',(-10.2852988189731,-1.95412485496321,
-0.607694875208273));
#30944=CARTESIAN_POINT('Ctrl Pts',(-10.3201303078758,-1.9568945579723,0.000687273504990337));
#30945=CARTESIAN_POINT('Ctrl Pts',(-10.4218696921242,-1.95677370715668,
0.000813444693687295));
#30946=CARTESIAN_POINT('Ctrl Pts',(-10.3874732343941,-1.95361135694641,
-0.600068805456268));
#30947=CARTESIAN_POINT('Ctrl Pts',(-10.3530767766639,-1.65603502305887,
-1.20365839229021));
#30948=CARTESIAN_POINT('Ctrl Pts',(-10.3186803189338,-1.17598871060954,
-1.56449602602075));
#30949=CARTESIAN_POINT('Ctrl Pts',(-10.2816671455962,-0.659422803964663,
-1.95278443608801));
#30950=CARTESIAN_POINT('Ctrl Pts',(-10.2446539722586,0.0684319743225153,
-2.05998120212456));
#30951=CARTESIAN_POINT('Ctrl Pts',(-10.2076407989211,0.675008551610066,
-1.83710661589606));
#30952=CARTESIAN_POINT('Ctrl Pts',(-10.1706276255835,1.28158512889762,-1.61423202966757));
#30953=CARTESIAN_POINT('Ctrl Pts',(-10.133614452246,1.76688350518553,-1.06128609117405));
#30954=CARTESIAN_POINT('Ctrl Pts',(-10.0966012789084,1.90916403518392,-0.430917567147205));
#30955=CARTESIAN_POINT('Ctrl Pts',(-10.0595881055708,2.05144456518231,0.199450956879657));
#30956=CARTESIAN_POINT('Ctrl Pts',(-10.0225749322333,1.85070724889113,0.907242066439859));
#30957=CARTESIAN_POINT('Ctrl Pts',(-9.9855617588957,1.39867178595441,1.36905606097446));
#30958=CARTESIAN_POINT('Ctrl Pts',(-9.94854858555813,0.946636323017702,
1.83087005550905));
#30959=CARTESIAN_POINT('Ctrl Pts',(-9.91153541222057,0.243302713435483,
2.04670693501808));
#30960=CARTESIAN_POINT('Ctrl Pts',(-9.87452223888301,-0.389966036589458,
1.91794779731423));
#30961=CARTESIAN_POINT('Ctrl Pts',(-9.83750906554544,-1.02323478661442,
1.78918865961037));
#30962=CARTESIAN_POINT('Ctrl Pts',(-9.80049589220787,-1.58643867708208,
1.31583350469361));
#30963=CARTESIAN_POINT('Ctrl Pts',(-9.76348271887031,-1.82224193890655,
0.71416495223856));
#30964=CARTESIAN_POINT('Ctrl Pts',(-9.74961170995494,-1.91061126399005,
0.488684424560365));
#30965=CARTESIAN_POINT('Ctrl Pts',(-9.73574070103958,-1.95299910665996,
0.245183038899142));
#30966=CARTESIAN_POINT('Ctrl Pts',(-9.72186969212421,-1.95160825484864,
0.00121583516621696));
#30967=CARTESIAN_POINT('Origin',(-9.8,0.,0.));
#30968=CARTESIAN_POINT('',(-8.92013030787576,-1.95219365985136,-0.00150278625351857));
#30969=CARTESIAN_POINT('',(-9.02186969212422,-1.95238063947443,-0.00156704507775435));
#30970=CARTESIAN_POINT('',(-9.8,-1.954,-2.39295984553393E-16));
#30971=CARTESIAN_POINT('Ctrl Pts',(-8.92013030787576,-1.95219365985136,
-0.00150278625351857));
#30972=CARTESIAN_POINT('Ctrl Pts',(-8.94482057892656,-1.94907401794518,
0.432429328865723));
#30973=CARTESIAN_POINT('Ctrl Pts',(-8.96951084997735,-1.80626939344938,
0.868225234004993));
#30974=CARTESIAN_POINT('Ctrl Pts',(-8.99420112102815,-1.54031802273755,
1.20748410194356));
#30975=CARTESIAN_POINT('Ctrl Pts',(-9.03121429436571,-1.1416304521042,1.71606690605629));
#30976=CARTESIAN_POINT('Ctrl Pts',(-9.06822746770327,-0.466195278319233,
2.00770208888324));
#30977=CARTESIAN_POINT('Ctrl Pts',(-9.10524064104083,0.177371679629828,
1.94913743868457));
#30978=CARTESIAN_POINT('Ctrl Pts',(-9.1422538143784,0.82093863757888,1.89057278848591));
#30979=CARTESIAN_POINT('Ctrl Pts',(-9.17926698771596,1.43263737969203,1.48180830526165));
#30980=CARTESIAN_POINT('Ctrl Pts',(-9.21628016105352,1.73297415794162,0.909614223461296));
#30981=CARTESIAN_POINT('Ctrl Pts',(-9.25329333439109,2.0333109361912,0.337420141660943));
#30982=CARTESIAN_POINT('Ctrl Pts',(-9.29030650772865,2.02228575057723,-0.398203538715502));
#30983=CARTESIAN_POINT('Ctrl Pts',(-9.32731968106622,1.70493616328153,-0.961140024528901));
#30984=CARTESIAN_POINT('Ctrl Pts',(-9.36433285440378,1.38758657598583,-1.52407651034231));
#30985=CARTESIAN_POINT('Ctrl Pts',(-9.40134602774135,0.763912587008396,
-1.91432580159266));
#30986=CARTESIAN_POINT('Ctrl Pts',(-9.43835920107891,0.118879602889872,
-1.95357751513302));
#30987=CARTESIAN_POINT('Ctrl Pts',(-9.47537237441648,-0.526153381228652,
-1.99282922867337));
#30988=CARTESIAN_POINT('Ctrl Pts',(-9.51238554775404,-1.19254536048827,
-1.68108336450373));
#30989=CARTESIAN_POINT('Ctrl Pts',(-9.54939872109161,-1.57581247851316,
-1.16078098717147));
#30990=CARTESIAN_POINT('Ctrl Pts',(-9.57297591668632,-1.81995160498805,
-0.829351125514365));
#30991=CARTESIAN_POINT('Ctrl Pts',(-9.59655311228104,-1.94920934795607,
-0.41329690177544));
#30992=CARTESIAN_POINT('Ctrl Pts',(-9.62013030787576,-1.951759122336,0.00130501714239645));
#30993=CARTESIAN_POINT('Ctrl Pts',(-9.72186969212421,-1.95160825484864,
0.00121583516621696));
#30994=CARTESIAN_POINT('Ctrl Pts',(-9.69872752770202,-1.94928778043318,
-0.405815057601631));
#30995=CARTESIAN_POINT('Ctrl Pts',(-9.67558536327982,-1.82510913530187,
-0.814142556830142));
#30996=CARTESIAN_POINT('Ctrl Pts',(-9.65244319885762,-1.58930196205156,
-1.14224189046578));
#30997=CARTESIAN_POINT('Ctrl Pts',(-9.61543002552006,-1.21215609019086,
-1.66699823072174));
#30998=CARTESIAN_POINT('Ctrl Pts',(-9.57841685218249,-0.549461713288179,
-1.98652896124034));
#30999=CARTESIAN_POINT('Ctrl Pts',(-9.54140367884493,0.0959867987391138,
-1.95483600268248));
#31000=CARTESIAN_POINT('Ctrl Pts',(-9.50439050550736,0.741435310766425,
-1.92314304412462));
#31001=CARTESIAN_POINT('Ctrl Pts',(-9.4673773321698,1.36963795791836,-1.54022639649028));
#31002=CARTESIAN_POINT('Ctrl Pts',(-9.43036415883223,1.69356012611861,-0.981046055053941));
#31003=CARTESIAN_POINT('Ctrl Pts',(-9.39335098549467,2.01748229431886,-0.421865713617614));
#31004=CARTESIAN_POINT('Ctrl Pts',(-9.3563378121571,2.03712398356746,0.313578321620689));
#31005=CARTESIAN_POINT('Ctrl Pts',(-9.31932463881954,1.74351063013272,0.889251339909027));
#31006=CARTESIAN_POINT('Ctrl Pts',(-9.28231146548198,1.44989727669798,1.46492435819737));
#31007=CARTESIAN_POINT('Ctrl Pts',(-9.24529829214442,0.843028880579888,
1.88082635953573));
#31008=CARTESIAN_POINT('Ctrl Pts',(-9.20828511880685,0.20019213686734,1.94692587718493));
#31009=CARTESIAN_POINT('Ctrl Pts',(-9.17127194546928,-0.442644606845208,
2.01302539483412));
#31010=CARTESIAN_POINT('Ctrl Pts',(-9.13425877213171,-1.12144969815222,
1.72932242879415));
#31011=CARTESIAN_POINT('Ctrl Pts',(-9.09724559879415,-1.52606755541189,
1.22544484952811));
#31012=CARTESIAN_POINT('Ctrl Pts',(-9.07212029657084,-1.80073046679972,
0.883402400285829));
#31013=CARTESIAN_POINT('Ctrl Pts',(-9.04699499434753,-1.94904863493835,
0.439904078837482));
#31014=CARTESIAN_POINT('Ctrl Pts',(-9.02186969212422,-1.95238063947443,
-0.00156704507775435));
#31015=CARTESIAN_POINT('Origin',(-9.8,0.,0.));
#31016=CARTESIAN_POINT('',(-8.22013030787576,-1.95711605195191,-0.000344670306376693));
#31017=CARTESIAN_POINT('',(-8.32186969212422,-1.95716419186761,-0.000205378326722651));
#31018=CARTESIAN_POINT('',(-9.8,-1.954,-2.39295984553393E-16));
#31019=CARTESIAN_POINT('Ctrl Pts',(-8.22013030787576,-1.95711605195191,
-0.000344670306376693));
#31020=CARTESIAN_POINT('Ctrl Pts',(-8.2560748722345,-1.95558481932104,0.627289137352789));
#31021=CARTESIAN_POINT('Ctrl Pts',(-8.29201943659324,-1.62669741337902,
1.25630241576526));
#31022=CARTESIAN_POINT('Ctrl Pts',(-8.32796400095198,-1.1097662979966,1.61214646711999));
#31023=CARTESIAN_POINT('Ctrl Pts',(-8.36497717428955,-0.577467150167943,
1.9785695352224));
#31024=CARTESIAN_POINT('Ctrl Pts',(-8.40199034762711,0.154222745866834,
2.05533964587135));
#31025=CARTESIAN_POINT('Ctrl Pts',(-8.43900352096467,0.750983998293585,
1.80737945709348));
#31026=CARTESIAN_POINT('Ctrl Pts',(-8.47601669430224,1.34774525072034,1.55941926831562));
#31027=CARTESIAN_POINT('Ctrl Pts',(-8.51302986763981,1.80957785953908,0.986728780110945));
#31028=CARTESIAN_POINT('Ctrl Pts',(-8.55004304097737,1.92546401824878,0.350978321333127));
#31029=CARTESIAN_POINT('Ctrl Pts',(-8.58705621431494,2.04135017695848,-0.284772137444683));
#31030=CARTESIAN_POINT('Ctrl Pts',(-8.62406938765249,1.81128988555918,-0.983582566795618));
#31031=CARTESIAN_POINT('Ctrl Pts',(-8.66108256099005,1.34040092293233,-1.42615666510335));
#31032=CARTESIAN_POINT('Ctrl Pts',(-8.69809573432762,0.869511960305483,
-1.86873076341109));
#31033=CARTESIAN_POINT('Ctrl Pts',(-8.73510890766519,0.157794326451077,
-2.05506853067559));
#31034=CARTESIAN_POINT('Ctrl Pts',(-8.77212208100276,-0.469558193964634,
-1.90002962347886));
#31035=CARTESIAN_POINT('Ctrl Pts',(-8.80913525434033,-1.09691071438035,
-1.74499071628214));
#31036=CARTESIAN_POINT('Ctrl Pts',(-8.84614842767788,-1.63989812135737,
-1.24857513462419));
#31037=CARTESIAN_POINT('Ctrl Pts',(-8.88316160101544,-1.85042184110501,
-0.637602131095955));
#31038=CARTESIAN_POINT('Ctrl Pts',(-8.89548450330222,-1.92051210880072,
-0.434189131252125));
#31039=CARTESIAN_POINT('Ctrl Pts',(-8.90780740558899,-1.95375067161119,
-0.218078094102745));
#31040=CARTESIAN_POINT('Ctrl Pts',(-8.92013030787576,-1.95219365985136,
-0.00150278625351857));
#31041=CARTESIAN_POINT('Ctrl Pts',(-9.02186969212422,-1.95238063947443,
-0.00156704507775435));
#31042=CARTESIAN_POINT('Ctrl Pts',(-9.00998182100997,-1.95395715545522,
-0.210446197062624));
#31043=CARTESIAN_POINT('Ctrl Pts',(-8.99809394989571,-1.92307638969601,
-0.418871531111766));
#31044=CARTESIAN_POINT('Ctrl Pts',(-8.98620607878146,-1.85776384109645,
-0.615882110172357));
#31045=CARTESIAN_POINT('Ctrl Pts',(-8.9491929054439,-1.65441164630902,-1.22927929811467));
#31046=CARTESIAN_POINT('Ctrl Pts',(-8.91217973210633,-1.11727663352183,
-1.73202148150718));
#31047=CARTESIAN_POINT('Ctrl Pts',(-8.87516655876876,-0.491783335409503,
-1.89439869455437));
#31048=CARTESIAN_POINT('Ctrl Pts',(-8.8381533854312,0.133709962702829,-2.05677590760156));
#31049=CARTESIAN_POINT('Ctrl Pts',(-8.80114021209364,0.84756154614031,-1.8787881503034));
#31050=CARTESIAN_POINT('Ctrl Pts',(-8.76412703875608,1.32360259869579,-1.44176052922861));
#31051=CARTESIAN_POINT('Ctrl Pts',(-8.72711386541851,1.79964365125125,-1.00473290815384));
#31052=CARTESIAN_POINT('Ctrl Pts',(-8.69010069208094,2.03787417292474,-0.308665423302459));
#31053=CARTESIAN_POINT('Ctrl Pts',(-8.65308751874338,1.9294432918523,0.328398913582165));
#31054=CARTESIAN_POINT('Ctrl Pts',(-8.61607434540581,1.82101241077986,0.965463250466808));
#31055=CARTESIAN_POINT('Ctrl Pts',(-8.57906117206825,1.36592012696147,1.54352443938468));
#31056=CARTESIAN_POINT('Ctrl Pts',(-8.54204799873069,0.772104497721655,
1.79845820288207));
#31057=CARTESIAN_POINT('Ctrl Pts',(-8.50503482539313,0.178288868481854,
2.05339196637945));
#31058=CARTESIAN_POINT('Ctrl Pts',(-8.46802165205556,-0.554250106179376,
1.98519830445635));
#31059=CARTESIAN_POINT('Ctrl Pts',(-8.431008478718,-1.09080507849613,1.62503585918676));
#31060=CARTESIAN_POINT('Ctrl Pts',(-8.39462888318673,-1.61817550132231,
1.27103854139505));
#31061=CARTESIAN_POINT('Ctrl Pts',(-8.35824928765548,-1.95621405916918,
0.634982516742313));
#31062=CARTESIAN_POINT('Ctrl Pts',(-8.32186969212422,-1.95716419186761,
-0.000205378326722651));
#31063=CARTESIAN_POINT('Origin',(-9.8,0.,0.));
#31064=CARTESIAN_POINT('',(-7.52013030787576,-1.95318687626922,0.00173935763946309));
#31065=CARTESIAN_POINT('',(-7.62186969212422,-1.95297113082797,0.00170789938961151));
#31066=CARTESIAN_POINT('',(-9.8,-1.954,-2.39295984553393E-16));
#31067=CARTESIAN_POINT('Ctrl Pts',(-7.52013030787576,-1.95318687626922,
0.00173935763946309));
#31068=CARTESIAN_POINT('Ctrl Pts',(-7.53031599220489,-1.95473250819494,
0.180522821393295));
#31069=CARTESIAN_POINT('Ctrl Pts',(-7.54050167653401,-1.93219994537477,
0.35892380617724));
#31070=CARTESIAN_POINT('Ctrl Pts',(-7.55068736086313,-1.88403259827928,
0.530111909164095));
#31071=CARTESIAN_POINT('Ctrl Pts',(-7.5877005342007,-1.70900004183546,1.15218252557468));
#31072=CARTESIAN_POINT('Ctrl Pts',(-7.62471370753826,-1.19546498257306,
1.67900839505789));
#31073=CARTESIAN_POINT('Ctrl Pts',(-7.66172688087582,-0.578068802883992,
1.86987537733102));
#31074=CARTESIAN_POINT('Ctrl Pts',(-7.69874005421339,0.0393273768050723,
2.06074235960415));
#31075=CARTESIAN_POINT('Ctrl Pts',(-7.73575322755095,0.760584676920769,
1.91565045466718));
#31076=CARTESIAN_POINT('Ctrl Pts',(-7.77276640088852,1.2561505052749,1.50089419204492));
#31077=CARTESIAN_POINT('Ctrl Pts',(-7.80977957422608,1.75171633362902,1.08613792942266));
#31078=CARTESIAN_POINT('Ctrl Pts',(-7.84679274756365,2.02159069022158,0.401717309115094));
#31079=CARTESIAN_POINT('Ctrl Pts',(-7.88380592090121,1.94246419050154,-0.239646273152209));
#31080=CARTESIAN_POINT('Ctrl Pts',(-7.92081909423877,1.8633376907815,-0.881009855419512));
#31081=CARTESIAN_POINT('Ctrl Pts',(-7.95783226757634,1.43521033474888,-1.47931639964656));
#31082=CARTESIAN_POINT('Ctrl Pts',(-7.9948454409139,0.85369952543667,-1.76119124114497));
#31083=CARTESIAN_POINT('Ctrl Pts',(-8.03185861425147,0.272188716124462,
-2.04306608264338));
#31084=CARTESIAN_POINT('Ctrl Pts',(-8.06887178758903,-0.462705546467319,
-2.00850922141314));
#31085=CARTESIAN_POINT('Ctrl Pts',(-8.1058849609266,-1.01519975043176,-1.67331017278323));
#31086=CARTESIAN_POINT('Ctrl Pts',(-8.14289813426416,-1.56769395439621,
-1.33811112415332));
#31087=CARTESIAN_POINT('Ctrl Pts',(-8.17991130760172,-1.9377880997333,-0.702269888123714));
#31088=CARTESIAN_POINT('Ctrl Pts',(-8.21692448093929,-1.95638097259055,
-0.0563112573309762));
#31089=CARTESIAN_POINT('Ctrl Pts',(-8.21799308991811,-1.95691776825236,
-0.0376617568809991));
#31090=CARTESIAN_POINT('Ctrl Pts',(-8.21906169889694,-1.95716157452165,
-0.0190038232059452));
#31091=CARTESIAN_POINT('Ctrl Pts',(-8.22013030787576,-1.95711605195191,
-0.000344670306376693));
#31092=CARTESIAN_POINT('Ctrl Pts',(-8.32186969212422,-1.95716419186761,
-0.000205378326722651));
#31093=CARTESIAN_POINT('Ctrl Pts',(-8.32123611431791,-1.95718073913763,
-0.0112676495606919));
#31094=CARTESIAN_POINT('Ctrl Pts',(-8.32060253651161,-1.95709504471771,
-0.0223296574838229));
#31095=CARTESIAN_POINT('Ctrl Pts',(-8.3199689587053,-1.9569063281076,-0.0333899075806545));
#31096=CARTESIAN_POINT('Ctrl Pts',(-8.28295578536774,-1.94588163543001,
-0.679522000462429));
#31097=CARTESIAN_POINT('Ctrl Pts',(-8.24594261203017,-1.5832612801025,-1.31965495760991));
#31098=CARTESIAN_POINT('Ctrl Pts',(-8.20892943869261,-1.03473159633512,
-1.66130303872038));
#31099=CARTESIAN_POINT('Ctrl Pts',(-8.17191626535504,-0.486201912567732,
-2.00295111983086));
#31100=CARTESIAN_POINT('Ctrl Pts',(-8.13490309201748,0.248237099639521,
-2.04611432490435));
#31101=CARTESIAN_POINT('Ctrl Pts',(-8.09788991867992,0.833009938675487,
-1.77107077921343));
#31102=CARTESIAN_POINT('Ctrl Pts',(-8.06087674534235,1.41778277771143,-1.49602723352252));
#31103=CARTESIAN_POINT('Ctrl Pts',(-8.02386357200479,1.85288944357609,-0.902776937067218));
#31104=CARTESIAN_POINT('Ctrl Pts',(-7.98685039866722,1.93952358853328,-0.262384283902055));
#31105=CARTESIAN_POINT('Ctrl Pts',(-7.94983722532966,2.02615773349047,0.378008369263136));
#31106=CARTESIAN_POINT('Ctrl Pts',(-7.91282405199209,1.76431935754017,1.06554337913819));
#31107=CARTESIAN_POINT('Ctrl Pts',(-7.87581087865453,1.2736460927936,1.48607634165523));
#31108=CARTESIAN_POINT('Ctrl Pts',(-7.83879770531696,0.782972828047029,
1.90660930417227));
#31109=CARTESIAN_POINT('Ctrl Pts',(-7.8017845319794,0.0634646745041936,
2.06014021933127));
#31110=CARTESIAN_POINT('Ctrl Pts',(-7.76477135864184,-0.556124985286757,
1.87651865529112));
#31111=CARTESIAN_POINT('Ctrl Pts',(-7.72775818530427,-1.17571464507769,
1.69289709125098));
#31112=CARTESIAN_POINT('Ctrl Pts',(-7.69074501196671,-1.69538581111674,
1.17212304801169));
#31113=CARTESIAN_POINT('Ctrl Pts',(-7.65373183862915,-1.87769342762954,
0.552145501432933));
#31114=CARTESIAN_POINT('Ctrl Pts',(-7.6431111231275,-1.93000554124126,0.374246538823964));
#31115=CARTESIAN_POINT('Ctrl Pts',(-7.63249040762586,-1.95454016061155,
0.188179459811748));
#31116=CARTESIAN_POINT('Ctrl Pts',(-7.62186969212422,-1.95297113082797,
0.00170789938961151));
#31117=CARTESIAN_POINT('Origin',(-9.8,0.,0.));
#31118=CARTESIAN_POINT('',(-6.82013030787576,-1.95113452083004,-0.00081409372327923));
#31119=CARTESIAN_POINT('',(-6.92186969212421,-1.95123700580418,-0.00092379545748507));
#31120=CARTESIAN_POINT('',(-9.8,-1.954,-2.39295984553393E-16));
#31121=CARTESIAN_POINT('Ctrl Pts',(-6.82013030787576,-1.95113452083004,
-0.00081409372327923));
#31122=CARTESIAN_POINT('Ctrl Pts',(-6.84157028551283,-1.94971586311403,
0.376507668247613));
#31123=CARTESIAN_POINT('Ctrl Pts',(-6.8630102631499,-1.84427610108052,0.754562607390817));
#31124=CARTESIAN_POINT('Ctrl Pts',(-6.88445024078697,-1.6399706578755,1.06821987854747));
#31125=CARTESIAN_POINT('Ctrl Pts',(-6.92146341412454,-1.28726540271326,
1.60970602850668));
#31126=CARTESIAN_POINT('Ctrl Pts',(-6.9584765874621,-0.639908041877813,
1.95926603940694));
#31127=CARTESIAN_POINT('Ctrl Pts',(-6.99548976079966,0.00631475279928184,
1.95718103187049));
#31128=CARTESIAN_POINT('Ctrl Pts',(-7.03250293413723,0.652537547476377,
1.95509602433404));
#31129=CARTESIAN_POINT('Ctrl Pts',(-7.0695161074748,1.29762577599512,1.60136599836088));
#31130=CARTESIAN_POINT('Ctrl Pts',(-7.10652928081236,1.64682956495479,1.05761517179331));
#31131=CARTESIAN_POINT('Ctrl Pts',(-7.14354245414993,1.99603335391445,0.513864345225741));
#31132=CARTESIAN_POINT('Ctrl Pts',(-7.18055562748749,2.04935270331504,-0.219907281936231));
#31133=CARTESIAN_POINT('Ctrl Pts',(-7.21756880082505,1.78242525341901,-0.80842914568362));
#31134=CARTESIAN_POINT('Ctrl Pts',(-7.25458197416262,1.51549780352297,-1.39695100943101));
#31135=CARTESIAN_POINT('Ctrl Pts',(-7.29159514750018,0.928323554330306,
-1.84022310976382));
#31136=CARTESIAN_POINT('Ctrl Pts',(-7.32860832083775,0.289190668548784,
-1.93570819723451));
#31137=CARTESIAN_POINT('Ctrl Pts',(-7.36562149417531,-0.349942217232729,
-2.0311932847052));
#31138=CARTESIAN_POINT('Ctrl Pts',(-7.40263466751287,-1.0410337396031,-1.77889135931378));
#31139=CARTESIAN_POINT('Ctrl Pts',(-7.43964784085044,-1.46831447397569,
-1.29408271494911));
#31140=CARTESIAN_POINT('Ctrl Pts',(-7.46647532985888,-1.77801148645166,
-0.942688943351297));
#31141=CARTESIAN_POINT('Ctrl Pts',(-7.49330281886732,-1.949115925103,-0.469148140320112));
#31142=CARTESIAN_POINT('Ctrl Pts',(-7.52013030787576,-1.95318687626922,
0.00173935763946309));
#31143=CARTESIAN_POINT('Ctrl Pts',(-7.62186969212422,-1.95297113082797,
0.00170789938961151));
#31144=CARTESIAN_POINT('Ctrl Pts',(-7.5954772342883,-1.94907209479786,-0.461673573852895));
#31145=CARTESIAN_POINT('Ctrl Pts',(-7.56908477645237,-1.7839773984951,-0.927552806989296));
#31146=CARTESIAN_POINT('Ctrl Pts',(-7.54269231861645,-1.48337286251048,
-1.27679372401467));
#31147=CARTESIAN_POINT('Ctrl Pts',(-7.50567914527889,-1.06180061389208,
-1.76657435296526));
#31148=CARTESIAN_POINT('Ctrl Pts',(-7.46866597194132,-0.373712049668737,
-2.02695456094817));
#31149=CARTESIAN_POINT('Ctrl Pts',(-7.43165279860376,0.266495499333949,
-1.93896297327993));
#31150=CARTESIAN_POINT('Ctrl Pts',(-7.39463962526619,0.906703048336636,
-1.85097138561169));
#31151=CARTESIAN_POINT('Ctrl Pts',(-7.35762645192863,1.49902958211867,-1.41460800229227));
#31152=CARTESIAN_POINT('Ctrl Pts',(-7.32061327859106,1.77283278676735,-0.829253382916534));
#31153=CARTESIAN_POINT('Ctrl Pts',(-7.2836001052535,2.04663599141603,-0.243898763540787));
#31154=CARTESIAN_POINT('Ctrl Pts',(-7.24658693191593,2.00191586693137,0.490447091891285));
#31155=CARTESIAN_POINT('Ctrl Pts',(-7.20957375857837,1.65910566639037,1.03825124640771));
#31156=CARTESIAN_POINT('Ctrl Pts',(-7.17256058524081,1.31629546584938,1.58605540092411));
#31157=CARTESIAN_POINT('Ctrl Pts',(-7.13554741190325,0.675395189252069,
1.94731785452487));
#31158=CARTESIAN_POINT('Ctrl Pts',(-7.09853423856568,0.0292411759365463,
1.95697271737387));
#31159=CARTESIAN_POINT('Ctrl Pts',(-7.06152106522812,-0.616912837378986,
1.96662758022286));
#31160=CARTESIAN_POINT('Ctrl Pts',(-7.02450789189055,-1.26832058741274,
1.62467485232006));
#31161=CARTESIAN_POINT('Ctrl Pts',(-6.98749471855299,-1.62734472261113,
1.08735753857942));
#31162=CARTESIAN_POINT('Ctrl Pts',(-6.96561970974339,-1.83953015315215,
0.769799763556305));
#31163=CARTESIAN_POINT('Ctrl Pts',(-6.9437447009338,-1.9495894566979,0.384003457058415));
#31164=CARTESIAN_POINT('Ctrl Pts',(-6.92186969212421,-1.95123700580418,
-0.00092379545748507));
#31165=CARTESIAN_POINT('Origin',(-9.8,0.,0.));
#31166=CARTESIAN_POINT('',(-6.12013030787576,-1.95615215220637,-0.00124808176673152));
#31167=CARTESIAN_POINT('',(-6.22186969212422,-1.95633073565045,-0.00114711649101067));
#31168=CARTESIAN_POINT('',(-9.8,-1.954,-2.39295984553393E-16));
#31169=CARTESIAN_POINT('Ctrl Pts',(-6.12013030787576,-1.95615215220637,
-0.00124808176673152));
#31170=CARTESIAN_POINT('Ctrl Pts',(-6.15282457882078,-1.95189699829043,
0.570376831194111));
#31171=CARTESIAN_POINT('Ctrl Pts',(-6.1855188497658,-1.68653473202121,1.14544077592247));
#31172=CARTESIAN_POINT('Ctrl Pts',(-6.21821312071081,-1.24643932389106,
1.50896868074674));
#31173=CARTESIAN_POINT('Ctrl Pts',(-6.25522629404838,-0.748207457715437,
1.9205185017209));
#31174=CARTESIAN_POINT('Ctrl Pts',(-6.29223946738595,-0.0260289193145019,
2.0609532286281));
#31175=CARTESIAN_POINT('Ctrl Pts',(-6.32925264072351,0.590122772410065,
1.86610626200643));
#31176=CARTESIAN_POINT('Ctrl Pts',(-6.36626581406107,1.20627446413461,1.67125929538477));
#31177=CARTESIAN_POINT('Ctrl Pts',(-6.40327898739864,1.71639930918277,1.14113063523426));
#31178=CARTESIAN_POINT('Ctrl Pts',(-6.4402921607362,1.88741409994161,0.517943513289022));
#31179=CARTESIAN_POINT('Ctrl Pts',(-6.47730533407376,2.05842889070045,-0.105243608656232));
#31180=CARTESIAN_POINT('Ctrl Pts',(-6.51431850741133,1.89033362716994,-0.821489192396225));
#31181=CARTESIAN_POINT('Ctrl Pts',(-6.55133168074889,1.45993339655288,-1.30353056935621));
#31182=CARTESIAN_POINT('Ctrl Pts',(-6.58834485408646,1.02953316593581,-1.78557194631621));
#31183=CARTESIAN_POINT('Ctrl Pts',(-6.62535802742402,0.336827968232211,
-2.03340911649619));
#31184=CARTESIAN_POINT('Ctrl Pts',(-6.66237120076159,-0.301675461043669,
-1.93380179538148));
#31185=CARTESIAN_POINT('Ctrl Pts',(-6.69938437409915,-0.940178890319522,
-1.83419447426678));
#31186=CARTESIAN_POINT('Ctrl Pts',(-6.73639754743671,-1.52448055116765,
-1.38714266185739));
#31187=CARTESIAN_POINT('Ctrl Pts',(-6.77341072077428,-1.7876048068472,-0.796910611143644));
#31188=CARTESIAN_POINT('Ctrl Pts',(-6.78898391647477,-1.89831364799068,
-0.548572022321792));
#31189=CARTESIAN_POINT('Ctrl Pts',(-6.80455711217527,-1.95216498059159,
-0.274886471068856));
#31190=CARTESIAN_POINT('Ctrl Pts',(-6.82013030787576,-1.95113452083004,
-0.00081409372327923));
#31191=CARTESIAN_POINT('Ctrl Pts',(-6.92186969212421,-1.95123700580418,
-0.00092379545748507));
#31192=CARTESIAN_POINT('Ctrl Pts',(-6.90673152759624,-1.9523771593765,-0.267305040402738));
#31193=CARTESIAN_POINT('Ctrl Pts',(-6.89159336306826,-1.90159831025379,
-0.5332700904781));
#31194=CARTESIAN_POINT('Ctrl Pts',(-6.87645519854029,-1.79681729382257,
-0.775915507987771));
#31195=CARTESIAN_POINT('Ctrl Pts',(-6.83944202520273,-1.54062520947259,
-1.3691893412358));
#31196=CARTESIAN_POINT('Ctrl Pts',(-6.80242885186517,-0.961600520409613,
-1.82305510815339));
#31197=CARTESIAN_POINT('Ctrl Pts',(-6.7654156785276,-0.324307740838284,
-1.93013516421731));
#31198=CARTESIAN_POINT('Ctrl Pts',(-6.72840250519004,0.312985038733054,
-2.03721522028122));
#31199=CARTESIAN_POINT('Ctrl Pts',(-6.69138933185246,1.00854590881273,-1.79750956549147));
#31200=CARTESIAN_POINT('Ctrl Pts',(-6.6543761585149,1.44456333706317,-1.32054308075455));
#31201=CARTESIAN_POINT('Ctrl Pts',(-6.61736298517734,1.8805807653136,-0.843576596017644));
#31202=CARTESIAN_POINT('Ctrl Pts',(-6.58034981183978,2.05705475173479,-0.129349281333571));
#31203=CARTESIAN_POINT('Ctrl Pts',(-6.54333663850222,1.8933518529362,0.49579837020592));
#31204=CARTESIAN_POINT('Ctrl Pts',(-6.50632346516465,1.72964895413761,1.12094602174541));
#31205=CARTESIAN_POINT('Ctrl Pts',(-6.46931029182709,1.22576917011926,1.65701401014033));
#31206=CARTESIAN_POINT('Ctrl Pts',(-6.43229711848952,0.611942252382899,
1.85906534114978));
#31207=CARTESIAN_POINT('Ctrl Pts',(-6.39528394515195,-0.00188466535346488,
2.06111667215922));
#31208=CARTESIAN_POINT('Ctrl Pts',(-6.35827077181439,-0.725658716807819,
1.92915134578318));
#31209=CARTESIAN_POINT('Ctrl Pts',(-6.32125759847683,-1.22867737075161,
1.5234661734081));
#31210=CARTESIAN_POINT('Ctrl Pts',(-6.28812829635929,-1.67891320449861,
1.1603504114159));
#31211=CARTESIAN_POINT('Ctrl Pts',(-6.25499899424176,-1.95229162706735,
0.577944956408698));
#31212=CARTESIAN_POINT('Ctrl Pts',(-6.22186969212422,-1.95633073565045,
-0.00114711649101067));
#31213=CARTESIAN_POINT('Origin',(-9.8,0.,0.));
#31214=CARTESIAN_POINT('',(-5.42013030787576,-1.9548899834603,0.00167775959234333));
#31215=CARTESIAN_POINT('',(-5.52186969212422,-1.95466140916787,0.00171701382729193));
#31216=CARTESIAN_POINT('',(-9.8,-1.954,-2.39295984553393E-16));
#31217=CARTESIAN_POINT('Ctrl Pts',(-5.42013030787576,-1.9548899834603,0.00167775959234333));
#31218=CARTESIAN_POINT('Ctrl Pts',(-5.42706569879116,-1.95599264273273,
0.123139444923241));
#31219=CARTESIAN_POINT('Ctrl Pts',(-5.43400108970656,-1.94564168131635,
0.244413763388184));
#31220=CARTESIAN_POINT('Ctrl Pts',(-5.44093648062196,-1.92315912390066,
0.363395723384609));
#31221=CARTESIAN_POINT('Ctrl Pts',(-5.47794965395953,-1.80317298254976,
0.998385151249712));
#31222=CARTESIAN_POINT('Ctrl Pts',(-5.51496282729709,-1.33765450945819,
1.56808358468529));
#31223=CARTESIAN_POINT('Ctrl Pts',(-5.55197600063466,-0.739305634289906,
1.81218780669216));
#31224=CARTESIAN_POINT('Ctrl Pts',(-5.58898917397222,-0.140956759121668,
2.05629202869902));
#31225=CARTESIAN_POINT('Ctrl Pts',(-5.62600234730978,0.590222518123277,
1.97480203927722));
#31226=CARTESIAN_POINT('Ctrl Pts',(-5.66301552064735,1.12014611452871,1.60495175931328));
#31227=CARTESIAN_POINT('Ctrl Pts',(-5.70002869398491,1.65006971093417,1.23510147934933));
#31228=CARTESIAN_POINT('Ctrl Pts',(-5.73704186732248,1.97873762650011,0.576890908843235));
#31229=CARTESIAN_POINT('Ctrl Pts',(-5.77405504066004,1.95597687368593,-0.0689342964159252));
#31230=CARTESIAN_POINT('Ctrl Pts',(-5.81106821399761,1.93321612087176,-0.714759501675086));
#31231=CARTESIAN_POINT('Ctrl Pts',(-5.84808138733517,1.55902669967746,-1.3481993416873));
#31232=CARTESIAN_POINT('Ctrl Pts',(-5.88509456067273,1.0043810130225,-1.67982625538966));
#31233=CARTESIAN_POINT('Ctrl Pts',(-5.9221077340103,0.449735326367551,-2.01145316909202));
#31234=CARTESIAN_POINT('Ctrl Pts',(-5.95912090734786,-0.285366625748073,
-2.04126715648452));
#31235=CARTESIAN_POINT('Ctrl Pts',(-5.99613408068543,-0.865046435156475,
-1.75564578791954));
#31236=CARTESIAN_POINT('Ctrl Pts',(-6.03314725402299,-1.44472624456488,
-1.47002441935456));
#31237=CARTESIAN_POINT('Ctrl Pts',(-6.07016042736056,-1.86898391126608,
-0.868967694832093));
#31238=CARTESIAN_POINT('Ctrl Pts',(-6.10717360069812,-1.94397014764153,
-0.227106875050304));
#31239=CARTESIAN_POINT('Ctrl Pts',(-6.11149250309067,-1.95271995768177,
-0.15221099392832));
#31240=CARTESIAN_POINT('Ctrl Pts',(-6.11581140548321,-1.95671425663314,
-0.0767595439546405));
#31241=CARTESIAN_POINT('Ctrl Pts',(-6.12013030787576,-1.95615215220637,
-0.00124808176673152));
#31242=CARTESIAN_POINT('Ctrl Pts',(-6.22186969212422,-1.95633073565045,
-0.00114711649101067));
#31243=CARTESIAN_POINT('Ctrl Pts',(-6.21798582090419,-1.95680425536194,
-0.0690362325279791));
#31244=CARTESIAN_POINT('Ctrl Pts',(-6.21410194968416,-1.95357604440152,
-0.136879810288365));
#31245=CARTESIAN_POINT('Ctrl Pts',(-6.21021807846414,-1.9464970931316,-0.204319184968079));
#31246=CARTESIAN_POINT('Ctrl Pts',(-6.17320490512657,-1.8790349051346,-0.847014352595043));
#31247=CARTESIAN_POINT('Ctrl Pts',(-6.136191731789,-1.46184727270742,-1.45299966947487));
#31248=CARTESIAN_POINT('Ctrl Pts',(-6.09917855845144,-0.885553085493417,
-1.7453919318276));
#31249=CARTESIAN_POINT('Ctrl Pts',(-6.06216538511387,-0.309258898279408,
-2.03778419418034));
#31250=CARTESIAN_POINT('Ctrl Pts',(-6.02515221177631,0.426141843721427,
-2.01658340200595));
#31251=CARTESIAN_POINT('Ctrl Pts',(-5.98813903843875,0.984634211045441,
-1.69147649506422));
#31252=CARTESIAN_POINT('Ctrl Pts',(-5.95112586510119,1.54312657836945,-1.36636958812248));
#31253=CARTESIAN_POINT('Ctrl Pts',(-5.91411269176361,1.92471057101666,-0.73735656641337));
#31254=CARTESIAN_POINT('Ctrl Pts',(-5.87709951842605,1.95503510249651,-0.0918423155320038));
#31255=CARTESIAN_POINT('Ctrl Pts',(-5.84008634508848,1.98535963397635,0.553671935349372));
#31256=CARTESIAN_POINT('Ctrl Pts',(-5.80307317175093,1.66442470428883,1.21568741540301));
#31257=CARTESIAN_POINT('Ctrl Pts',(-5.76605999841336,1.13886999109862,1.59171995221861));
#31258=CARTESIAN_POINT('Ctrl Pts',(-5.7290468250758,0.613315277908424,1.96775248903421));
#31259=CARTESIAN_POINT('Ctrl Pts',(-5.69203365173823,-0.11685921878447,
2.05780208261176));
#31260=CARTESIAN_POINT('Ctrl Pts',(-5.65502047840067,-0.718026514412586,
1.82072380868607));
#31261=CARTESIAN_POINT('Ctrl Pts',(-5.6180073050631,-1.31919381004069,1.58364553476039));
#31262=CARTESIAN_POINT('Ctrl Pts',(-5.58099413172554,-1.79135390460403,
1.01943939333149));
#31263=CARTESIAN_POINT('Ctrl Pts',(-5.54398095838797,-1.91877021829093,
0.385899096028444));
#31264=CARTESIAN_POINT('Ctrl Pts',(-5.53661053630006,-1.94414259055943,
0.259742406942544));
#31265=CARTESIAN_POINT('Ctrl Pts',(-5.52924011421213,-1.95584496273636,
0.130836435723866));
#31266=CARTESIAN_POINT('Ctrl Pts',(-5.52186969212422,-1.95466140916787,
0.00171701382729193));
#31267=CARTESIAN_POINT('Origin',(-9.8,0.,0.));
#31268=CARTESIAN_POINT('',(-4.72013030787576,-1.95081049221722,9.12023351157254E-5));
#31269=CARTESIAN_POINT('',(-4.82186969212422,-1.95080680701216,-3.40121725118189E-5));
#31270=CARTESIAN_POINT('',(-9.8,-1.954,-2.39295984553393E-16));
#31271=CARTESIAN_POINT('Ctrl Pts',(-4.72013030787576,-1.95081049221722,
9.12023351157254E-5));
#31272=CARTESIAN_POINT('Ctrl Pts',(-4.73831999209911,-1.95094405902827,
0.3203439412756));
#31273=CARTESIAN_POINT('Ctrl Pts',(-4.75650967632245,-1.8764768769041,0.640538180196498));
#31274=CARTESIAN_POINT('Ctrl Pts',(-4.7746993605458,-1.72706848364466,0.9207778887538));
#31275=CARTESIAN_POINT('Ctrl Pts',(-4.81171253388337,-1.42304568204481,
1.49102203271679));
#31276=CARTESIAN_POINT('Ctrl Pts',(-4.84872570722094,-0.808721983960032,
1.89583081204337));
#31277=CARTESIAN_POINT('Ctrl Pts',(-4.8857388805585,-0.164790516675161,
1.9502414089621));
#31278=CARTESIAN_POINT('Ctrl Pts',(-4.92275205389606,0.479140950609711,
2.00465200588084));
#31279=CARTESIAN_POINT('Ctrl Pts',(-4.95976522723362,1.15268018709468,1.70866442039174));
#31280=CARTESIAN_POINT('Ctrl Pts',(-4.99677840057119,1.54807765417753,1.19751953815074));
#31281=CARTESIAN_POINT('Ctrl Pts',(-5.03379157390875,1.94347512126036,0.686374655909763));
#31282=CARTESIAN_POINT('Ctrl Pts',(-5.07080474724632,2.0607308189411,-0.0399275230830835));
#31283=CARTESIAN_POINT('Ctrl Pts',(-5.10781792058388,1.84626897181572,-0.649529330613395));
#31284=CARTESIAN_POINT('Ctrl Pts',(-5.14483109392145,1.63180712469032,-1.25913113814376));
#31285=CARTESIAN_POINT('Ctrl Pts',(-5.18184426725901,1.08562773275873,-1.75203257421157));
#31286=CARTESIAN_POINT('Ctrl Pts',(-5.21885744059658,0.457287832576391,
-1.90302004871051));
#31287=CARTESIAN_POINT('Ctrl Pts',(-5.25587061393414,-0.171052067605934,
-2.05400752320944));
#31288=CARTESIAN_POINT('Ctrl Pts',(-5.2928837872717,-0.881552476039011,
-1.86308103613953));
#31289=CARTESIAN_POINT('Ctrl Pts',(-5.32989696060927,-1.34957577545042,
-1.41747758145727));
#31290=CARTESIAN_POINT('Ctrl Pts',(-5.35997474303143,-1.72990260773292,
-1.05536964668869));
#31291=CARTESIAN_POINT('Ctrl Pts',(-5.39005252545359,-1.95010791045442,
-0.525083916652837));
#31292=CARTESIAN_POINT('Ctrl Pts',(-5.42013030787576,-1.9548899834603,0.00167775959234333));
#31293=CARTESIAN_POINT('Ctrl Pts',(-5.52186969212422,-1.95466140916787,
0.00171701382729193));
#31294=CARTESIAN_POINT('Ctrl Pts',(-5.49222694087457,-1.94990133116922,
-0.517582269052512));
#31295=CARTESIAN_POINT('Ctrl Pts',(-5.46258418962493,-1.73670755972907,
-1.04033418033024));
#31296=CARTESIAN_POINT('Ctrl Pts',(-5.43294143837528,-1.36608778935965,
-1.40157105231175));
#31297=CARTESIAN_POINT('Ctrl Pts',(-5.39592826503772,-0.903316513931034,
-1.85262645017167));
#31298=CARTESIAN_POINT('Ctrl Pts',(-5.35891509170015,-0.195101430263383,
-2.05186279271431));
#31299=CARTESIAN_POINT('Ctrl Pts',(-5.32190191836259,0.43496404135903,-1.90824619628611));
#31300=CARTESIAN_POINT('Ctrl Pts',(-5.28488874502503,1.06502951298146,-1.76462959985791));
#31301=CARTESIAN_POINT('Ctrl Pts',(-5.24787557168746,1.61694537255866,-1.2781600644588));
#31302=CARTESIAN_POINT('Ctrl Pts',(-5.2108623983499,1.83853351088562,-0.671112354428362));
#31303=CARTESIAN_POINT('Ctrl Pts',(-5.17384922501233,2.06012164921258,-0.0640646443979367));
#31304=CARTESIAN_POINT('Ctrl Pts',(-5.13683605167477,1.95138206628935,0.66356124026384));
#31305=CARTESIAN_POINT('Ctrl Pts',(-5.0998228783372,1.56199940505829,1.17930281162784));
#31306=CARTESIAN_POINT('Ctrl Pts',(-5.06280970499964,1.17261674382722,1.69504438299186));
#31307=CARTESIAN_POINT('Ctrl Pts',(-5.02579653166207,0.502591004288316,
1.99890164105808));
#31308=CARTESIAN_POINT('Ctrl Pts',(-4.98878335832451,-0.141933641066262,
1.9520379362219));
#31309=CARTESIAN_POINT('Ctrl Pts',(-4.95177018498695,-0.78645828642084,
1.90517423138573));
#31310=CARTESIAN_POINT('Ctrl Pts',(-4.91475701164938,-1.40548183759107,
1.50758956364717));
#31311=CARTESIAN_POINT('Ctrl Pts',(-4.87774383831182,-1.71616373839683,
0.940945952713336));
#31312=CARTESIAN_POINT('Ctrl Pts',(-4.85911912291595,-1.87249624002759,
0.655815686030199));
#31313=CARTESIAN_POINT('Ctrl Pts',(-4.84049440752008,-1.95075610609356,
0.32787940450784));
#31314=CARTESIAN_POINT('Ctrl Pts',(-4.82186969212422,-1.95080709904697,
-3.40090619142402E-5));
#31315=CARTESIAN_POINT('Origin',(-9.8,0.,0.));
#31316=CARTESIAN_POINT('',(-4.02013030787576,-1.9545563311611,-0.00173175715877188));
#31317=CARTESIAN_POINT('',(-4.12186969212422,-1.95478583214071,-0.00169688232281055));
#31318=CARTESIAN_POINT('',(-9.8,-1.954,-2.39295984553393E-16));
#31319=CARTESIAN_POINT('Ctrl Pts',(-4.02013030787576,-1.9545563311611,-0.00173175715877189));
#31320=CARTESIAN_POINT('Ctrl Pts',(-4.04957428540706,-1.94981507723237,
0.514156697093934));
#31321=CARTESIAN_POINT('Ctrl Pts',(-4.07901826293835,-1.73977891611187,
1.03345910076901));
#31322=CARTESIAN_POINT('Ctrl Pts',(-4.10846224046964,-1.37357022290306,
1.39423897175874));
#31323=CARTESIAN_POINT('Ctrl Pts',(-4.14547541380721,-0.913219856684524,
1.84776492243762));
#31324=CARTESIAN_POINT('Ctrl Pts',(-4.18248858714477,-0.206081319881922,
2.05078916635255));
#31325=CARTESIAN_POINT('Ctrl Pts',(-4.21950176048234,0.424743856605548,
1.91054707450309));
#31326=CARTESIAN_POINT('Ctrl Pts',(-4.2565149338199,1.055569033093,1.77030498265363));
#31327=CARTESIAN_POINT('Ctrl Pts',(-4.29352810715747,1.61008084926532,1.28679655503981));
#31328=CARTESIAN_POINT('Ctrl Pts',(-4.33054128049503,1.83491506688298,0.68094358425817));
#31329=CARTESIAN_POINT('Ctrl Pts',(-4.3675544538326,2.05974928450064,0.0750906134765319));
#31330=CARTESIAN_POINT('Ctrl Pts',(-4.40456762717016,1.95490590356363,-0.653106900472918));
#31331=CARTESIAN_POINT('Ctrl Pts',(-4.44158080050773,1.56828933759538,-1.17092528420956));
#31332=CARTESIAN_POINT('Ctrl Pts',(-4.47859397384529,1.18167277162715,-1.68874366794618));
#31333=CARTESIAN_POINT('Ctrl Pts',(-4.51560714718285,0.513283020627696,
-1.99618292147001));
#31334=CARTESIAN_POINT('Ctrl Pts',(-4.55262032052042,-0.131483249055789,
-1.95276973113429));
#31335=CARTESIAN_POINT('Ctrl Pts',(-4.58963349385798,-0.776249518739292,
-1.90935654079856));
#31336=CARTESIAN_POINT('Ctrl Pts',(-4.62664666719555,-1.39739230710683,
-1.51509090660327));
#31337=CARTESIAN_POINT('Ctrl Pts',(-4.66365984053311,-1.71110274873313,
-0.950118335205926));
#31338=CARTESIAN_POINT('Ctrl Pts',(-4.68248332964733,-1.87064392152352,
-0.662794820668581));
#31339=CARTESIAN_POINT('Ctrl Pts',(-4.70130681876154,-1.95067227137827,
-0.331320485257933));
#31340=CARTESIAN_POINT('Ctrl Pts',(-4.72013030787576,-1.95081049221722,
9.12023351157254E-5));
#31341=CARTESIAN_POINT('Ctrl Pts',(-4.82186969212422,-1.95080709904697,
-3.40090619142402E-5));
#31342=CARTESIAN_POINT('Ctrl Pts',(-4.80348123418252,-1.95085744514672,
-0.323787789228885));
#31343=CARTESIAN_POINT('Ctrl Pts',(-4.78509277624082,-1.87467051708849,
-0.647519277930666));
#31344=CARTESIAN_POINT('Ctrl Pts',(-4.76670431829912,-1.72211519641974,
-0.930008878009234));
#31345=CARTESIAN_POINT('Ctrl Pts',(-4.72969114496156,-1.41504450319559,
-1.49861754366889));
#31346=CARTESIAN_POINT('Ctrl Pts',(-4.69267797162399,-0.798562866305986,
-1.9001323208591));
#31347=CARTESIAN_POINT('Ctrl Pts',(-4.65566479828643,-0.154349405589037,
-1.9510954676566));
#31348=CARTESIAN_POINT('Ctrl Pts',(-4.61865162494886,0.489864055127912,
-2.00205861445409));
#31349=CARTESIAN_POINT('Ctrl Pts',(-4.5816384516113,1.16180933967221,-1.70247013085888));
#31350=CARTESIAN_POINT('Ctrl Pts',(-4.54462527827373,1.55446520847415,-1.18921620345471));
#31351=CARTESIAN_POINT('Ctrl Pts',(-4.50761210493617,1.94712107727608,-0.675962276050554));
#31352=CARTESIAN_POINT('Ctrl Pts',(-4.47059893159861,2.06048753033567,0.0509570951625461));
#31353=CARTESIAN_POINT('Ctrl Pts',(-4.43358575826104,1.84276584274993,0.659402238174801));
#31354=CARTESIAN_POINT('Ctrl Pts',(-4.39657258492348,1.62504415516418,1.26784738118709));
#31355=CARTESIAN_POINT('Ctrl Pts',(-4.35955941158591,1.07623432693307,1.75781829599852));
#31356=CARTESIAN_POINT('Ctrl Pts',(-4.32254623824835,0.447095277907961,
1.90544038883094));
#31357=CARTESIAN_POINT('Ctrl Pts',(-4.28553306491079,-0.182043771117111,
2.05306248166334));
#31358=CARTESIAN_POINT('Ctrl Pts',(-4.24851989157322,-0.891512040936168,
1.85833575251678));
#31359=CARTESIAN_POINT('Ctrl Pts',(-4.21150671823566,-1.35714351290836,
1.41023357933592));
#31360=CARTESIAN_POINT('Ctrl Pts',(-4.18162770953184,-1.73302608522773,
1.0485015924414));
#31361=CARTESIAN_POINT('Ctrl Pts',(-4.15174870082803,-1.95001045891771,
0.52165547187433));
#31362=CARTESIAN_POINT('Ctrl Pts',(-4.12186969212422,-1.95478583214071,
-0.00169688232281055));
#31363=CARTESIAN_POINT('Origin',(-9.8,0.,0.));
#31364=CARTESIAN_POINT('',(-3.32013030787577,-1.95640828841667,0.00109851928146481));
#31365=CARTESIAN_POINT('',(-3.42186969212422,-1.95623519870294,0.0012028883663872));
#31366=CARTESIAN_POINT('',(-9.8,-1.954,-2.39295984553393E-16));
#31367=CARTESIAN_POINT('Ctrl Pts',(-3.32013030787577,-1.95640828841667,
0.00109851928146481));
#31368=CARTESIAN_POINT('Ctrl Pts',(-3.32381540537744,-1.95684244368226,
0.0655064059659674));
#31369=CARTESIAN_POINT('Ctrl Pts',(-3.32750050287912,-1.95393695034547,
0.12987464599085));
#31370=CARTESIAN_POINT('Ctrl Pts',(-3.3311856003808,-1.94756288843026,0.193897558538627));
#31371=CARTESIAN_POINT('Ctrl Pts',(-3.36819877371836,-1.8835417170977,0.836944630869362));
#31372=CARTESIAN_POINT('Ctrl Pts',(-3.40521194705592,-1.46960361082938,
1.44515429704656));
#31373=CARTESIAN_POINT('Ctrl Pts',(-3.44222512039348,-0.894882705104787,
1.74062701683428));
#31374=CARTESIAN_POINT('Ctrl Pts',(-3.47923829373105,-0.320161799380146,
2.03609973662201));
#31375=CARTESIAN_POINT('Ctrl Pts',(-3.51625146706862,0.415341905800802,
2.0188355100202));
#31376=CARTESIAN_POINT('Ctrl Pts',(-3.55326464040618,0.975566435643367,
1.69672260468841));
#31377=CARTESIAN_POINT('Ctrl Pts',(-3.59027781374375,1.53579096548592,1.37460969935663));
#31378=CARTESIAN_POINT('Ctrl Pts',(-3.62729098708131,1.92073631999009,0.747648115294896));
#31379=CARTESIAN_POINT('Ctrl Pts',(-3.66430416041887,1.95451555921865,0.102305407415552));
#31380=CARTESIAN_POINT('Ctrl Pts',(-3.70131733375644,1.98829479844721,-0.543037300463793));
#31381=CARTESIAN_POINT('Ctrl Pts',(-3.738330507094,1.67090792240016,-1.20676113216074));
#31382=CARTESIAN_POINT('Ctrl Pts',(-3.77534368043157,1.14737345319091,-1.58560134539902));
#31383=CARTESIAN_POINT('Ctrl Pts',(-3.81235685376913,0.623838983981661,
-1.9644415586373));
#31384=CARTESIAN_POINT('Ctrl Pts',(-3.8493700271067,-0.105843078389784,
-2.05839815341691));
#31385=CARTESIAN_POINT('Ctrl Pts',(-3.88638320044426,-0.708270749513731,
-1.82454104174156));
#31386=CARTESIAN_POINT('Ctrl Pts',(-3.92339637378182,-1.31069842063764,
-1.59068393006623));
#31387=CARTESIAN_POINT('Ctrl Pts',(-3.96040954711939,-1.78587170051407,
-1.02901311193597));
#31388=CARTESIAN_POINT('Ctrl Pts',(-3.99742272045695,-1.91667724263507,
-0.396163874149472));
#31389=CARTESIAN_POINT('Ctrl Pts',(-4.00499191626322,-1.94342698256765,
-0.266746173241493));
#31390=CARTESIAN_POINT('Ctrl Pts',(-4.01256111206949,-1.95577517054229,
-0.13435177156693));
#31391=CARTESIAN_POINT('Ctrl Pts',(-4.02013030787576,-1.9545563311611,-0.00173175715877189));
#31392=CARTESIAN_POINT('Ctrl Pts',(-4.12186969212422,-1.95478583214071,
-0.00169688232281055));
#31393=CARTESIAN_POINT('Ctrl Pts',(-4.11473552749047,-1.95592604060941,
-0.126656913404005));
#31394=CARTESIAN_POINT('Ctrl Pts',(-4.10760136285672,-1.94496813473903,
-0.251417763560148));
#31395=CARTESIAN_POINT('Ctrl Pts',(-4.10046719822296,-1.9211864330455,-0.373684295091019));
#31396=CARTESIAN_POINT('Ctrl Pts',(-4.0634540248854,-1.79780320708513,-1.00802237912193));
#31397=CARTESIAN_POINT('Ctrl Pts',(-4.02644085154783,-1.32924208103907,
-1.57522092996857));
#31398=CARTESIAN_POINT('Ctrl Pts',(-3.98942767821027,-0.729595215447372,
-1.81611896210353));
#31399=CARTESIAN_POINT('Ctrl Pts',(-3.95241450487271,-0.129948349855691,
-2.05701699423849));
#31400=CARTESIAN_POINT('Ctrl Pts',(-3.91540133153514,0.600784255281619,
-1.97161450766178));
#31401=CARTESIAN_POINT('Ctrl Pts',(-3.87838815819758,1.12872060780878,-1.5989330981701));
#31402=CARTESIAN_POINT('Ctrl Pts',(-3.84137498486002,1.65665696033596,-1.22625168867841));
#31403=CARTESIAN_POINT('Ctrl Pts',(-3.80436181152245,1.98179706025298,-0.566291356271734));
#31404=CARTESIAN_POINT('Ctrl Pts',(-3.76734863818489,1.95557982854599,0.0794027524685451));
#31405=CARTESIAN_POINT('Ctrl Pts',(-3.73033546484732,1.92936259683899,0.725096861208825));
#31406=CARTESIAN_POINT('Ctrl Pts',(-3.69332229150975,1.55178803350799,1.3565247462827));
#31407=CARTESIAN_POINT('Ctrl Pts',(-3.65630911817219,0.995375260466554,
1.68517813710198));
#31408=CARTESIAN_POINT('Ctrl Pts',(-3.61929594483462,0.438962487425118,
2.01383152792126));
#31409=CARTESIAN_POINT('Ctrl Pts',(-3.58228277149706,-0.296288495326749,
2.03971042448594));
#31410=CARTESIAN_POINT('Ctrl Pts',(-3.5452695981595,-0.874431185429084,
1.7509903954239));
#31411=CARTESIAN_POINT('Ctrl Pts',(-3.50825642482194,-1.45257387553142,
1.46227036636187));
#31412=CARTESIAN_POINT('Ctrl Pts',(-3.47124325148437,-1.87360827298422,
0.858951411673132));
#31413=CARTESIAN_POINT('Ctrl Pts',(-3.4342300781468,-1.94515784716871,0.216698436799811));
#31414=CARTESIAN_POINT('Ctrl Pts',(-3.43010994947261,-1.95312240209988,
0.145205920507576));
#31415=CARTESIAN_POINT('Ctrl Pts',(-3.42598982079841,-1.95675646506019,
0.0732309699275622));
#31416=CARTESIAN_POINT('Ctrl Pts',(-3.42186969212422,-1.95623519870294,
0.0012028883663872));
#31417=CARTESIAN_POINT('Origin',(-9.8,0.,0.));
#31418=CARTESIAN_POINT('',(-2.62013030787576,-1.95128826882871,0.000972458038924484));
#31419=CARTESIAN_POINT('',(-2.72186969212422,-1.95117967829402,0.000864741168076029));
#31420=CARTESIAN_POINT('',(-9.8,-1.954,-2.39295984553393E-16));
#31421=CARTESIAN_POINT('Ctrl Pts',(-2.62013030787576,-1.95128826882871,
0.000972458038924484));
#31422=CARTESIAN_POINT('Ctrl Pts',(-2.63506969868539,-1.95247456011625,
0.263838687422591));
#31423=CARTESIAN_POINT('Ctrl Pts',(-2.65000908949501,-1.90306670254861,
0.526277490250255));
#31424=CARTESIAN_POINT('Ctrl Pts',(-2.66494848030464,-1.8009447216931,0.766286875754349));
#31425=CARTESIAN_POINT('Ctrl Pts',(-2.7019616536422,-1.54793182262993,1.3609235046176));
#31426=CARTESIAN_POINT('Ctrl Pts',(-2.73897482697977,-0.97134474800472,
1.81788203573128));
#31427=CARTESIAN_POINT('Ctrl Pts',(-2.77598800031733,-0.334634231049586,
1.92837169641715));
#31428=CARTESIAN_POINT('Ctrl Pts',(-2.81300117365489,0.302076285905531,
2.03886135710302));
#31429=CARTESIAN_POINT('Ctrl Pts',(-2.85001434699246,0.998910245190565,
1.80288214736111));
#31430=CARTESIAN_POINT('Ctrl Pts',(-2.88702752033002,1.4374744217618,1.32825628340228));
#31431=CARTESIAN_POINT('Ctrl Pts',(-2.92404069366758,1.87603859833305,0.85363041944343));
#31432=CARTESIAN_POINT('Ctrl Pts',(-2.96105386700515,2.05633299219049,0.140357901267651));
#31433=CARTESIAN_POINT('Ctrl Pts',(-2.99806704034272,1.89597856231094,-0.485657038177132));
#31434=CARTESIAN_POINT('Ctrl Pts',(-3.03508021368028,1.7356241324314,-1.11167197762192));
#31435=CARTESIAN_POINT('Ctrl Pts',(-3.07209338701784,1.23462087881487,-1.6504293383357));
#31436=CARTESIAN_POINT('Ctrl Pts',(-3.10910656035541,0.621884225714157,
-1.85576331397781));
#31437=CARTESIAN_POINT('Ctrl Pts',(-3.14611973369297,0.00914757261343817,
-2.06109728961992));
#31438=CARTESIAN_POINT('Ctrl Pts',(-3.18313290703054,-0.715322479971475,
-1.93300788019034));
#31439=CARTESIAN_POINT('Ctrl Pts',(-3.2201460803681,-1.22050538806554,-1.5300209362334));
#31440=CARTESIAN_POINT('Ctrl Pts',(-3.25347415620399,-1.67539138550219,
-1.16715609061264));
#31441=CARTESIAN_POINT('Ctrl Pts',(-3.28680223203988,-1.95248178182908,
-0.581407352238547));
#31442=CARTESIAN_POINT('Ctrl Pts',(-3.32013030787577,-1.95640828841667,
0.00109851928146481));
#31443=CARTESIAN_POINT('Ctrl Pts',(-3.42186969212422,-1.95623519870294,
0.0012028883663872));
#31444=CARTESIAN_POINT('Ctrl Pts',(-3.38897664746085,-1.9520736690697,-0.573833255200393));
#31445=CARTESIAN_POINT('Ctrl Pts',(-3.35608360279748,-1.68306698074724,
-1.15225576891058));
#31446=CARTESIAN_POINT('Ctrl Pts',(-3.32319055813411,-1.23834461947855,
-1.51561864145381));
#31447=CARTESIAN_POINT('Ctrl Pts',(-3.28617738479655,-0.737917066687742,
-1.92449574977619));
#31448=CARTESIAN_POINT('Ctrl Pts',(-3.24916421145898,-0.0149972101899386,
-2.06106297136309));
#31449=CARTESIAN_POINT('Ctrl Pts',(-3.21215103812142,0.60010271245489,-1.86292082425223));
#31450=CARTESIAN_POINT('Ctrl Pts',(-3.17513786478386,1.21520263509974,-1.66477867714137));
#31451=CARTESIAN_POINT('Ctrl Pts',(-3.13812469144629,1.7224826238916,-1.13192716133273));
#31452=CARTESIAN_POINT('Ctrl Pts',(-3.10111151810873,1.89015932601566,-0.507833619577597));
#31453=CARTESIAN_POINT('Ctrl Pts',(-3.06409834477116,2.05783602813972,0.116259922177535));
#31454=CARTESIAN_POINT('Ctrl Pts',(-3.0270851714336,1.88590944359597,0.831595489879161));
#31455=CARTESIAN_POINT('Ctrl Pts',(-2.99007199809603,1.4529352439555,1.31132621409805));
#31456=CARTESIAN_POINT('Ctrl Pts',(-2.95305882475847,1.01996104431503,1.79105693831693));
#31457=CARTESIAN_POINT('Ctrl Pts',(-2.91604565142091,0.325939229577842,
2.03518281905308));
#31458=CARTESIAN_POINT('Ctrl Pts',(-2.87903247808334,-0.312021883881085,
1.93215931200737));
#31459=CARTESIAN_POINT('Ctrl Pts',(-2.84201930474578,-0.949982997340013,
1.82913580496166));
#31460=CARTESIAN_POINT('Ctrl Pts',(-2.80500613140821,-1.53188340952068,
1.3789629101341));
#31461=CARTESIAN_POINT('Ctrl Pts',(-2.76799295807065,-1.79184464801151,
0.787330947038803));
#31462=CARTESIAN_POINT('Ctrl Pts',(-2.7526185360885,-1.89982657496242,0.541580619829814));
#31463=CARTESIAN_POINT('Ctrl Pts',(-2.73724411410636,-1.95226173617185,
0.271423217094667));
#31464=CARTESIAN_POINT('Ctrl Pts',(-2.72186969212422,-1.95117967829402,
0.000864741168076028));
#31465=CARTESIAN_POINT('Origin',(-9.8,0.,0.));
#31466=CARTESIAN_POINT('',(-1.92013030787577,-1.95287461439042,-0.00169055101731763));
#31467=CARTESIAN_POINT('',(-2.02186969212423,-1.95308757850967,-0.00172609056776994));
#31468=CARTESIAN_POINT('',(-9.8,-1.954,-2.39295984553393E-16));
#31469=CARTESIAN_POINT('Ctrl Pts',(-1.92013030787577,-1.95287461439042,
-0.00169055101731763));
#31470=CARTESIAN_POINT('Ctrl Pts',(-1.94632399199334,-1.94905843635623,
0.458258638527069));
#31471=CARTESIAN_POINT('Ctrl Pts',(-1.97251767611091,-1.78666677165177,
0.920633103135576));
#31472=CARTESIAN_POINT('Ctrl Pts',(-1.99871136022848,-1.49018573369743,
1.26883564400827));
#31473=CARTESIAN_POINT('Ctrl Pts',(-2.03572453356604,-1.07124107513584,
1.7608657434801));
#31474=CARTESIAN_POINT('Ctrl Pts',(-2.07273770690361,-0.384556063773794,
2.02492527078759));
#31475=CARTESIAN_POINT('Ctrl Pts',(-2.10975088024117,0.256113305508671,
1.94036168303737));
#31476=CARTESIAN_POINT('Ctrl Pts',(-2.14676405357874,0.896782674791118,
1.85579809528716));
#31477=CARTESIAN_POINT('Ctrl Pts',(-2.1837772269163,1.49143640199399,1.42261139247926));
#31478=CARTESIAN_POINT('Ctrl Pts',(-2.22079040025386,1.76836882853465,0.838730682929604));
#31479=CARTESIAN_POINT('Ctrl Pts',(-2.25780357359143,2.04530125507533,0.254849973379925));
#31480=CARTESIAN_POINT('Ctrl Pts',(-2.29481674692899,2.00451238095378,-0.479724742911528));
#31481=CARTESIAN_POINT('Ctrl Pts',(-2.33182992026656,1.66463922482719,-1.0293559690438));
#31482=CARTESIAN_POINT('Ctrl Pts',(-2.36884309360412,1.32476606870059,-1.57898719517607));
#31483=CARTESIAN_POINT('Ctrl Pts',(-2.40585626694168,0.685808630568944,
-1.94367493114915));
#31484=CARTESIAN_POINT('Ctrl Pts',(-2.44286944027925,0.0397155348038179,
-1.95678822233774));
#31485=CARTESIAN_POINT('Ctrl Pts',(-2.47988261361681,-0.606377560961308,
-1.96990151352634));
#31486=CARTESIAN_POINT('Ctrl Pts',(-2.51689578695438,-1.25960631435991,
-1.63144035993043));
#31487=CARTESIAN_POINT('Ctrl Pts',(-2.55390896029194,-1.62150132930865,
-1.09605241982608));
#31488=CARTESIAN_POINT('Ctrl Pts',(-2.57598274281988,-1.83732697022491,
-0.776759695309758));
#31489=CARTESIAN_POINT('Ctrl Pts',(-2.59805652534782,-1.94953545733662,
-0.387427046016949));
#31490=CARTESIAN_POINT('Ctrl Pts',(-2.62013030787576,-1.95128826882871,
0.000972458038924484));
#31491=CARTESIAN_POINT('Ctrl Pts',(-2.72186969212422,-1.95117967829402,
0.000864741168076028));
#31492=CARTESIAN_POINT('Ctrl Pts',(-2.7002309407688,-1.94965673444626,-0.379933157736906));
#31493=CARTESIAN_POINT('Ctrl Pts',(-2.67859218941338,-1.84212049455112,
-0.761525550296575));
#31494=CARTESIAN_POINT('Ctrl Pts',(-2.65695343805795,-1.63422943147789,
-1.07698255705823));
#31495=CARTESIAN_POINT('Ctrl Pts',(-2.61994026472039,-1.27863091165242,
-1.61657306669692));
#31496=CARTESIAN_POINT('Ctrl Pts',(-2.58292709138282,-0.629411807200471,
-1.9626630546113));
#31497=CARTESIAN_POINT('Ctrl Pts',(-2.54591391804526,0.0167905529389563,
-1.95711914322188));
#31498=CARTESIAN_POINT('Ctrl Pts',(-2.5089007447077,0.662992913078401,-1.95157523183247));
#31499=CARTESIAN_POINT('Ctrl Pts',(-2.47188757137013,1.30617852890533,-1.59439742113925));
#31500=CARTESIAN_POINT('Ctrl Pts',(-2.43487439803257,1.65246685804866,-1.04878527110899));
#31501=CARTESIAN_POINT('Ctrl Pts',(-2.397861224695,1.998755187192,-0.503173121078729));
#31502=CARTESIAN_POINT('Ctrl Pts',(-2.36084805135744,2.04814622965175,0.230873368288563));
#31503=CARTESIAN_POINT('Ctrl Pts',(-2.32383487801987,1.77807252324082,0.817958046205187));
#31504=CARTESIAN_POINT('Ctrl Pts',(-2.28682170468231,1.50799881682989,1.40504272412181));
#31505=CARTESIAN_POINT('Ctrl Pts',(-2.24980853134475,0.918460361548285,
1.84516559058777));
#31506=CARTESIAN_POINT('Ctrl Pts',(-2.21279535800718,0.27882556111846,1.93722832225799));
#31507=CARTESIAN_POINT('Ctrl Pts',(-2.17578218466962,-0.360809239311365,
2.02929105392822));
#31508=CARTESIAN_POINT('Ctrl Pts',(-2.13876901133205,-1.05054038488941,
1.77329365080272));
#31509=CARTESIAN_POINT('Ctrl Pts',(-2.10175583799449,-1.47522003017977,
1.28620492833718));
#31510=CARTESIAN_POINT('Ctrl Pts',(-2.0751271227044,-1.78075107073109,0.935774372349613));
#31511=CARTESIAN_POINT('Ctrl Pts',(-2.04849840741431,-1.9490935021035,0.465732734518825));
#31512=CARTESIAN_POINT('Ctrl Pts',(-2.02186969212423,-1.95308757850967,
-0.00172609056776994));
#31513=CARTESIAN_POINT('Origin',(-9.8,0.,0.));
#31514=CARTESIAN_POINT('',(-1.22013030787577,-1.95717923962325,0.000142060037185308));
#31515=CARTESIAN_POINT('',(-1.32186969212423,-1.95714098413823,0.000281429570410231));
#31516=CARTESIAN_POINT('',(-9.8,-1.954,-2.39295984553393E-16));
#31517=CARTESIAN_POINT('Ctrl Pts',(-1.22013030787577,-1.95717923962325,
0.000142060037185308));
#31518=CARTESIAN_POINT('Ctrl Pts',(-1.22056511196372,-1.95718716035574,
0.00773360395988979));
#31519=CARTESIAN_POINT('Ctrl Pts',(-1.22099991605168,-1.95714681216893,
0.0153250610537409));
#31520=CARTESIAN_POINT('Ctrl Pts',(-1.22143472013963,-1.95705794020611,
0.0229159496253129));
#31521=CARTESIAN_POINT('Ctrl Pts',(-1.25844789347719,-1.94949261721163,
0.669098638040081));
#31522=CARTESIAN_POINT('Ctrl Pts',(-1.29546106681476,-1.59030209252517,
1.31116155718884));
#31523=CARTESIAN_POINT('Ctrl Pts',(-1.33247424015232,-1.04360853567726,
1.65574034778633));
#31524=CARTESIAN_POINT('Ctrl Pts',(-1.36948741348988,-0.496914978829352,
2.00031913838382));
#31525=CARTESIAN_POINT('Ctrl Pts',(-1.40650058682745,0.237281610179996,
2.04741380043005));
#31526=CARTESIAN_POINT('Ctrl Pts',(-1.44351376016501,0.823518058849043,
1.77550443541525));
#31527=CARTESIAN_POINT('Ctrl Pts',(-1.48052693350258,1.40975450751809,1.50359507040046));
#31528=CARTESIAN_POINT('Ctrl Pts',(-1.51754010684014,1.84803081584683,0.91268167832465));
#31529=CARTESIAN_POINT('Ctrl Pts',(-1.55455328017771,1.93809156072536,0.27276177482246));
#31530=CARTESIAN_POINT('Ctrl Pts',(-1.59156645351527,2.02815230560389,-0.367158128679712));
#31531=CARTESIAN_POINT('Ctrl Pts',(-1.62857962685283,1.76999748703222,-1.05608454360826));
#31532=CARTESIAN_POINT('Ctrl Pts',(-1.6655928001904,1.28158209960214,-1.47923777903418));
#31533=CARTESIAN_POINT('Ctrl Pts',(-1.70260597352796,0.793166712172057,
-1.90239101446009));
#31534=CARTESIAN_POINT('Ctrl Pts',(-1.73961914686552,0.0744907558835552,
-2.05977107038337));
#31535=CARTESIAN_POINT('Ctrl Pts',(-1.77663232020309,-0.546072856156742,
-1.87946854374991));
#31536=CARTESIAN_POINT('Ctrl Pts',(-1.81364549354065,-1.16663646819707,
-1.69916601711645));
#31537=CARTESIAN_POINT('Ctrl Pts',(-1.85065866687822,-1.68908773598919,
-1.18118090792619));
#31538=CARTESIAN_POINT('Ctrl Pts',(-1.88767184021578,-1.87471121700467,
-0.562188017512963));
#31539=CARTESIAN_POINT('Ctrl Pts',(-1.89849132943578,-1.9289716618876,-0.381247387429709));
#31540=CARTESIAN_POINT('Ctrl Pts',(-1.90931081865577,-1.95445091411662,
-0.191675864869495));
#31541=CARTESIAN_POINT('Ctrl Pts',(-1.92013030787577,-1.95287461439042,
-0.00169055101731763));
#31542=CARTESIAN_POINT('Ctrl Pts',(-2.02186969212423,-1.95308757850967,
-0.00172609056776994));
#31543=CARTESIAN_POINT('Ctrl Pts',(-2.01148523407675,-1.95464515717716,
-0.184022025807307));
#31544=CARTESIAN_POINT('Ctrl Pts',(-2.00110077602927,-1.93120891772511,
-0.365925171280384));
#31545=CARTESIAN_POINT('Ctrl Pts',(-1.9907163179818,-1.8811681159904,-0.540188658624532));
#31546=CARTESIAN_POINT('Ctrl Pts',(-1.95370314464423,-1.70280841150797,
-1.16131348131528));
#31547=CARTESIAN_POINT('Ctrl Pts',(-1.91668997130667,-1.18646085754039,
-1.6853830848912));
#31548=CARTESIAN_POINT('Ctrl Pts',(-1.8796767979691,-0.568051918879918,
-1.87294268440246));
#31549=CARTESIAN_POINT('Ctrl Pts',(-1.84266362463154,0.05035701978055,-2.06050228391373));
#31550=CARTESIAN_POINT('Ctrl Pts',(-1.80565045129397,0.770827343133897,
-1.91155187936033));
#31551=CARTESIAN_POINT('Ctrl Pts',(-1.76863727795641,1.2641660664822,-1.49414904342711));
#31552=CARTESIAN_POINT('Ctrl Pts',(-1.73162410461884,1.75750478983048,-1.07674620749391));
#31553=CARTESIAN_POINT('Ctrl Pts',(-1.69461093128128,2.02371191317375,-0.39089094018093));
#31554=CARTESIAN_POINT('Ctrl Pts',(-1.65759775794372,1.94115361144894,0.250039929439042));
#31555=CARTESIAN_POINT('Ctrl Pts',(-1.62058458460615,1.85859530972413,0.890970799059033));
#31556=CARTESIAN_POINT('Ctrl Pts',(-1.58357141126859,1.42727158293121,1.48697727098601));
#31557=CARTESIAN_POINT('Ctrl Pts',(-1.54655823793102,0.84426039764207,1.76573546933512));
#31558=CARTESIAN_POINT('Ctrl Pts',(-1.50954506459346,0.261249212352931,
2.04449366768423));
#31559=CARTESIAN_POINT('Ctrl Pts',(-1.47253189125589,-0.473449431432427,
2.00600359245548));
#31560=CARTESIAN_POINT('Ctrl Pts',(-1.43551871791833,-1.02414158702801,
1.66785217850744));
#31561=CARTESIAN_POINT('Ctrl Pts',(-1.39850554458076,-1.57483374262357,
1.32970076455941));
#31562=CARTESIAN_POINT('Ctrl Pts',(-1.3614923712432,-1.94151941002937,0.691888011892126));
#31563=CARTESIAN_POINT('Ctrl Pts',(-1.32447919790564,-1.95665440631073,
0.0458389963489571));
#31564=CARTESIAN_POINT('Ctrl Pts',(-1.32360936264517,-1.95701008922699,
0.0306563961275103));
#31565=CARTESIAN_POINT('Ctrl Pts',(-1.3227395273847,-1.95717161681812,0.0154692471612372));
#31566=CARTESIAN_POINT('Ctrl Pts',(-1.32186969212423,-1.95714098413823,
0.000281429570410231));
#31567=CARTESIAN_POINT('Origin',(-9.8,0.,0.));
#31568=CARTESIAN_POINT('',(-0.520130307875779,-1.95245178959834,0.00157515171675247));
#31569=CARTESIAN_POINT('',(-0.62186969212423,-1.9522756157026,0.00152956335005719));
#31570=CARTESIAN_POINT('',(-9.8,-1.954,-2.39295984553393E-16));
#31571=CARTESIAN_POINT('Ctrl Pts',(-0.520130307875779,-1.95245178959834,
0.00157515171675247));
#31572=CARTESIAN_POINT('Ctrl Pts',(-0.531819405271675,-1.95405741327078,
0.20696418498022));
#31573=CARTESIAN_POINT('Ctrl Pts',(-0.543508502667571,-1.92424637327528,
0.41190437232312));
#31574=CARTESIAN_POINT('Ctrl Pts',(-0.555197600063466,-1.86107514875473,
0.605974135111533));
#31575=CARTESIAN_POINT('Ctrl Pts',(-0.59221077340103,-1.66104537708507,
1.22049016884649));
#31576=CARTESIAN_POINT('Ctrl Pts',(-0.629223946738595,-1.12652869134443,
1.72601355713792));
#31577=CARTESIAN_POINT('Ctrl Pts',(-0.66623712007616,-0.501894415972446,
1.89171586961104));
#31578=CARTESIAN_POINT('Ctrl Pts',(-0.703250293413725,0.122739859399543,
2.05741818208416));
#31579=CARTESIAN_POINT('Ctrl Pts',(-0.740263466751291,0.837491724402904,
1.88329941873898));
#31580=CARTESIAN_POINT('Ctrl Pts',(-0.777276640088856,1.31585516795866,
1.44883687645897));
#31581=CARTESIAN_POINT('Ctrl Pts',(-0.814289813426421,1.79421861151443,
1.01437433417895));
#31582=CARTESIAN_POINT('Ctrl Pts',(-0.851302986763983,2.03619363362259,
0.31956801296412));
#31583=CARTESIAN_POINT('Ctrl Pts',(-0.888316160101548,1.93117947666614,
-0.318073271893728));
#31584=CARTESIAN_POINT('Ctrl Pts',(-0.925329333439112,1.82616531970969,
-0.955714556751558));
#31585=CARTESIAN_POINT('Ctrl Pts',(-0.962342506776676,1.37416198368861,
-1.53619080525239));
#31586=CARTESIAN_POINT('Ctrl Pts',(-0.99935568011424,0.78171662343255,-1.79429636290242));
#31587=CARTESIAN_POINT('Ctrl Pts',(-1.0363688534518,0.189271263176508,-2.05240192055245));
#31588=CARTESIAN_POINT('Ctrl Pts',(-1.07338202678937,-0.543616121314529,
-1.98813678735172));
#31589=CARTESIAN_POINT('Ctrl Pts',(-1.11039520012693,-1.08208975290879,
-1.63085299191098));
#31590=CARTESIAN_POINT('Ctrl Pts',(-1.14697356937655,-1.61423778431377,
-1.27776630903335));
#31591=CARTESIAN_POINT('Ctrl Pts',(-1.18355193862616,-1.95651289934287,
-0.638504871936492));
#31592=CARTESIAN_POINT('Ctrl Pts',(-1.22013030787577,-1.95717923962325,
0.000142060037185308));
#31593=CARTESIAN_POINT('Ctrl Pts',(-1.32186969212423,-1.95714098413823,
0.000281429570410231));
#31594=CARTESIAN_POINT('Ctrl Pts',(-1.28572635404713,-1.95586813701901,
-0.630801777543932));
#31595=CARTESIAN_POINT('Ctrl Pts',(-1.24958301597004,-1.62281842013958,
-1.26303940726775));
#31596=CARTESIAN_POINT('Ctrl Pts',(-1.21343967789294,-1.10112109627574,
-1.61806369501833));
#31597=CARTESIAN_POINT('Ctrl Pts',(-1.17642650455538,-0.566868464802466,
-1.98163209242336));
#31598=CARTESIAN_POINT('Ctrl Pts',(-1.13941333121781,0.165221123300993,
-2.05448360881435));
#31599=CARTESIAN_POINT('Ctrl Pts',(-1.10240015788025,0.760646920128182,
-1.8033332830397));
#31600=CARTESIAN_POINT('Ctrl Pts',(-1.06538698454269,1.35607271695537,-1.55218295726506));
#31601=CARTESIAN_POINT('Ctrl Pts',(-1.02837381120512,1.81483472250629,-0.977030789324784));
#31602=CARTESIAN_POINT('Ctrl Pts',(-0.991360637867557,1.9273157180188,-0.3406682310869));
#31603=CARTESIAN_POINT('Ctrl Pts',(-0.954347464529993,2.03979671353132,
0.295694327150984));
#31604=CARTESIAN_POINT('Ctrl Pts',(-0.917334291192428,1.80599669900544,
0.993267275686475));
#31605=CARTESIAN_POINT('Ctrl Pts',(-0.880321117854863,1.33274677819716,
1.43331278513124));
#31606=CARTESIAN_POINT('Ctrl Pts',(-0.843307944517299,0.85949685738889,
1.87335829457599));
#31607=CARTESIAN_POINT('Ctrl Pts',(-0.806294771179734,0.146797030298244,
2.05587636493003));
#31608=CARTESIAN_POINT('Ctrl Pts',(-0.769281597842171,-0.479718878710562,
1.89748514905269));
#31609=CARTESIAN_POINT('Ctrl Pts',(-0.732268424504606,-1.10623478771939,
1.73909393317535));
#31610=CARTESIAN_POINT('Ctrl Pts',(-0.695255251167042,-1.64656677864637,
1.2397934310666));
#31611=CARTESIAN_POINT('Ctrl Pts',(-0.658242077829478,-1.85381294957979,
0.62769589808096));
#31612=CARTESIAN_POINT('Ctrl Pts',(-0.646117949261062,-1.92169902891681,
0.427195683774921));
#31613=CARTESIAN_POINT('Ctrl Pts',(-0.633993820692646,-1.95384592951114,
0.214592662906205));
#31614=CARTESIAN_POINT('Ctrl Pts',(-0.62186969212423,-1.9522756157026,0.00152956335005719));
#31615=CARTESIAN_POINT('Origin',(-20.9400562256037,0.,0.));
#31616=CARTESIAN_POINT('',(-0.29005622560372,-1.55426753261014,0.00125391427617921));
#31617=CARTESIAN_POINT('',(-0.151943774396314,-1.55328440515865,-0.00159394639174151));
#31618=CARTESIAN_POINT('',(-20.9400562256037,-1.5555,1.83293981223255E-13));
#31619=CARTESIAN_POINT('',(-3.11417115573063E-15,1.33818917000755,-0.797967911694413));
#31620=CARTESIAN_POINT('Ctrl Pts',(-0.29005622560372,-1.55426753261014,
0.00125391427617923));
#31621=CARTESIAN_POINT('Ctrl Pts',(-0.26473214966205,-1.55149841214987,
-0.352967927424292));
#31622=CARTESIAN_POINT('Ctrl Pts',(-0.202394900382818,-1.2557305975322,
-1.22904168662576));
#31623=CARTESIAN_POINT('Ctrl Pts',(-0.105709491848242,0.158347209672706,
-1.81077139712758));
#31624=CARTESIAN_POINT('Ctrl Pts',(-0.0343481592553409,1.09133363889359,
-1.20698403335016));
#31625=CARTESIAN_POINT('Ctrl Pts',(-3.13063377305189E-15,1.3381957767388,
-0.797970124357324));
#31626=CARTESIAN_POINT('',(0.,-0.31962117020207,-1.5223082991164));
#31627=CARTESIAN_POINT('Origin',(0.,0.,0.));
#31628=CARTESIAN_POINT('Ctrl Pts',(-0.151943774396314,-1.55328440515865,
-0.00159394639174141));
#31629=CARTESIAN_POINT('Ctrl Pts',(-0.138309022935107,-1.55435366600215,
-0.192572897595738));
#31630=CARTESIAN_POINT('Ctrl Pts',(-0.0876610981363355,-1.43339236355893,
-0.900161415364349));
#31631=CARTESIAN_POINT('Ctrl Pts',(-0.0370131733375646,-0.825376844998173,
-1.41612072810435));
#31632=CARTESIAN_POINT('Ctrl Pts',(0.,-0.319621170202026,-1.52230829911641));
#31633=CARTESIAN_POINT('Origin',(-20.9400562256037,0.,0.));
#31634=CARTESIAN_POINT('',(-0.990056225603717,-1.55803086347695,0.000113088223220368));
#31635=CARTESIAN_POINT('',(-0.851943774396308,-1.5541272877305,0.00121762323000714));
#31636=CARTESIAN_POINT('',(-20.9400562256037,-1.5555,1.83293981223255E-13));
#31637=CARTESIAN_POINT('Ctrl Pts',(-0.990056225603717,-1.55803086347695,
0.000113088223220355));
#31638=CARTESIAN_POINT('Ctrl Pts',(-0.953477856354101,-1.55750041705627,
-0.508287783161193));
#31639=CARTESIAN_POINT('Ctrl Pts',(-0.879886313766922,-1.00931895110904,
-1.53211702555747));
#31640=CARTESIAN_POINT('Ctrl Pts',(-0.769281597842172,0.734093027864279,
-1.68499263158297));
#31641=CARTESIAN_POINT('Ctrl Pts',(-0.658242077829484,1.81355749436498,
-0.29871196954151));
#31642=CARTESIAN_POINT('Ctrl Pts',(-0.547202557816791,1.23567804673567,
1.36060926789406));
#31643=CARTESIAN_POINT('Ctrl Pts',(-0.436163037804095,-0.47127670149265,
1.77643588465474));
#31644=CARTESIAN_POINT('Ctrl Pts',(-0.350447593733071,-1.4566697208266,
0.844492633449843));
#31645=CARTESIAN_POINT('Ctrl Pts',(-0.301745322999614,-1.55554570437189,
0.164755777756869));
#31646=CARTESIAN_POINT('Ctrl Pts',(-0.29005622560372,-1.55426753261014,
0.00125391427617923));
#31647=CARTESIAN_POINT('Ctrl Pts',(-0.851943774396308,-1.5541272877305,
0.00121762323000714));
#31648=CARTESIAN_POINT('Ctrl Pts',(-0.827054729627156,-1.55156109304348,
-0.346968447042236));
#31649=CARTESIAN_POINT('Ctrl Pts',(-0.765152511520438,-1.26385222212854,
-1.21679022327445));
#31650=CARTESIAN_POINT('Ctrl Pts',(-0.66623712007616,0.17630871353902,-1.82941001051451));
#31651=CARTESIAN_POINT('Ctrl Pts',(-0.555197600063458,1.63206374948406,
-0.84563791873513));
#31652=CARTESIAN_POINT('Ctrl Pts',(-0.444158080050773,1.59603445699364,
0.91144468152982));
#31653=CARTESIAN_POINT('Ctrl Pts',(-0.333118560038075,0.102187466450462,
1.83458816486299));
#31654=CARTESIAN_POINT('Ctrl Pts',(-0.235713791486592,-1.29129161789087,
1.17548693359841));
#31655=CARTESIAN_POINT('Ctrl Pts',(-0.175322196272671,-1.55145102879193,
0.325862443514162));
#31656=CARTESIAN_POINT('Ctrl Pts',(-0.151943774396314,-1.55328440515865,
-0.00159394639174141));
#31657=CARTESIAN_POINT('Origin',(-20.9400562256037,0.,0.));
#31658=CARTESIAN_POINT('',(-1.69005622560371,-1.5546041262458,-0.00134577896985914));
#31659=CARTESIAN_POINT('',(-1.55194377439631,-1.55800040983982,0.000224034645440537));
#31660=CARTESIAN_POINT('',(-20.9400562256037,-1.5555,1.83293981223255E-13));
#31661=CARTESIAN_POINT('Ctrl Pts',(-1.69005622560371,-1.5546041262458,-0.00134577896985951));
#31662=CARTESIAN_POINT('Ctrl Pts',(-1.67923673638372,-1.55585895440554,
-0.152585367351205));
#31663=CARTESIAN_POINT('Ctrl Pts',(-1.63140407382615,-1.46618838413473,
-0.819755125015001));
#31664=CARTESIAN_POINT('Ctrl Pts',(-1.54655823793103,-0.512809661837298,
-1.76498391861309));
#31665=CARTESIAN_POINT('Ctrl Pts',(-1.43551871791833,1.20351651524581,-1.3891323162764));
#31666=CARTESIAN_POINT('Ctrl Pts',(-1.32447919790564,1.82003619839053,0.256146657758448));
#31667=CARTESIAN_POINT('Ctrl Pts',(-1.21343967789295,0.77335431875082,1.66735307747278));
#31668=CARTESIAN_POINT('Ctrl Pts',(-1.10240015788025,-0.980037893435529,
1.55488263712548));
#31669=CARTESIAN_POINT('Ctrl Pts',(-1.02793900711718,-1.55527083732047,
0.526637965405178));
#31670=CARTESIAN_POINT('Ctrl Pts',(-0.990491029691664,-1.55803716885023,
0.00615640786072333));
#31671=CARTESIAN_POINT('Ctrl Pts',(-0.990056225603717,-1.55803086347695,
0.000113088223220355));
#31672=CARTESIAN_POINT('Ctrl Pts',(-1.55194377439631,-1.55800040983982,
0.000224034645440697));
#31673=CARTESIAN_POINT('Ctrl Pts',(-1.51580043631921,-1.55698714796992,
-0.502155662727371));
#31674=CARTESIAN_POINT('Ctrl Pts',(-1.44264392490454,-1.0203518296671,-1.52086555639993));
#31675=CARTESIAN_POINT('Ctrl Pts',(-1.33247424015232,0.714312595491066,
-1.69348504977325));
#31676=CARTESIAN_POINT('Ctrl Pts',(-1.22143472013962,1.8099179685225,-0.319919240308951));
#31677=CARTESIAN_POINT('Ctrl Pts',(-1.11039520012693,1.25156189493757,1.34600919589416));
#31678=CARTESIAN_POINT('Ctrl Pts',(-0.999355680114236,-0.45049222129505,
1.78189485367676));
#31679=CARTESIAN_POINT('Ctrl Pts',(-0.913205204870696,-1.45166145172168,
0.856751964042876));
#31680=CARTESIAN_POINT('Ctrl Pts',(-0.86406790296472,-1.55537735074439,
0.170828499053688));
#31681=CARTESIAN_POINT('Ctrl Pts',(-0.851943774396308,-1.5541272877305,
0.00121762323000714));
#31682=CARTESIAN_POINT('Origin',(-20.9400562256037,0.,0.));
#31683=CARTESIAN_POINT('',(-2.39005622560371,-1.55334130100463,0.000774134329562734));
#31684=CARTESIAN_POINT('',(-2.2519437743963,-1.55477365832743,-0.00137407056183869));
#31685=CARTESIAN_POINT('',(-20.9400562256037,-1.5555,1.83293981223255E-13));
#31686=CARTESIAN_POINT('Ctrl Pts',(-2.39005622560371,-1.55334130100463,
0.000774134329562682));
#31687=CARTESIAN_POINT('Ctrl Pts',(-2.36798244307577,-1.55194595900061,
-0.30841492839256));
#31688=CARTESIAN_POINT('Ctrl Pts',(-2.30889548721026,-1.31284241169292,
-1.1380386041486));
#31689=CARTESIAN_POINT('Ctrl Pts',(-2.21279535800718,0.0372963305200237,
-1.8375937199123));
#31690=CARTESIAN_POINT('Ctrl Pts',(-2.10175583799449,1.56324048867835,-0.966654456903947));
#31691=CARTESIAN_POINT('Ctrl Pts',(-1.9907163179818,1.66065158442465,0.787640790575088));
#31692=CARTESIAN_POINT('Ctrl Pts',(-1.87967679796911,0.2405125782874,1.82216778579164));
#31693=CARTESIAN_POINT('Ctrl Pts',(-1.77945676717641,-1.23962210290448,
1.25299318928825));
#31694=CARTESIAN_POINT('Ctrl Pts',(-1.71624990972128,-1.5515662219816,0.364801080977023));
#31695=CARTESIAN_POINT('Ctrl Pts',(-1.69005622560371,-1.5546041262458,-0.00134577896985951));
#31696=CARTESIAN_POINT('Ctrl Pts',(-2.2519437743963,-1.55477365832743,-0.00137407056183876));
#31697=CARTESIAN_POINT('Ctrl Pts',(-2.24155931634882,-1.55601358341305,
-0.146492457084467));
#31698=CARTESIAN_POINT('Ctrl Pts',(-2.19416168496378,-1.4708593613734,-0.807427026857451));
#31699=CARTESIAN_POINT('Ctrl Pts',(-2.10975088024117,-0.533449971191177,
-1.75885550507193));
#31700=CARTESIAN_POINT('Ctrl Pts',(-1.99871136022847,1.18716147401266,-1.40313541149553));
#31701=CARTESIAN_POINT('Ctrl Pts',(-1.88767184021578,1.82291149503699,0.234809115073605));
#31702=CARTESIAN_POINT('Ctrl Pts',(-1.77663232020309,0.792833618333258,
1.65817871653077));
#31703=CARTESIAN_POINT('Ctrl Pts',(-1.66559280019039,-0.96175759007224,
1.56625756194791));
#31704=CARTESIAN_POINT('Ctrl Pts',(-1.5906966182548,-1.5524246457012,0.538851764154201));
#31705=CARTESIAN_POINT('Ctrl Pts',(-1.55281360965677,-1.55802479527153,
0.0123144390786119));
#31706=CARTESIAN_POINT('Ctrl Pts',(-1.55194377439631,-1.55800040983982,
0.000224034645440697));
#31707=CARTESIAN_POINT('Origin',(-20.9400562256037,0.,0.));
#31708=CARTESIAN_POINT('',(-3.09005622560371,-1.55741714054868,0.000874486562257179));
#31709=CARTESIAN_POINT('',(-2.9519437743963,-1.5532548564925,0.00068838530571283));
#31710=CARTESIAN_POINT('',(-20.9400562256037,-1.5555,1.83293981223255E-13));
#31711=CARTESIAN_POINT('Ctrl Pts',(-3.09005622560371,-1.55741714054868,
0.000874486562257217));
#31712=CARTESIAN_POINT('Ctrl Pts',(-3.05672814976782,-1.55429140820636,
-0.462834767864285));
#31713=CARTESIAN_POINT('Ctrl Pts',(-2.98638690059437,-1.08874094224246,
-1.44697424618156));
#31714=CARTESIAN_POINT('Ctrl Pts',(-2.87903247808334,0.584003181164767,
-1.74272257439688));
#31715=CARTESIAN_POINT('Ctrl Pts',(-2.76799295807065,1.78048817758317,-0.456074046366774));
#31716=CARTESIAN_POINT('Ctrl Pts',(-2.65695343805795,1.34991305530291,1.24734775817125));
#31717=CARTESIAN_POINT('Ctrl Pts',(-2.54591391804527,-0.314250542958959,
1.81090813803855));
#31718=CARTESIAN_POINT('Ctrl Pts',(-2.45694818056051,-1.41750787088368,
0.93655130592161));
#31719=CARTESIAN_POINT('Ctrl Pts',(-2.40499561641333,-1.55428565929415,
0.210031258078886));
#31720=CARTESIAN_POINT('Ctrl Pts',(-2.39005622560371,-1.55334130100463,
0.000774134329562682));
#31721=CARTESIAN_POINT('Ctrl Pts',(-2.9519437743963,-1.5532548564925,0.000688385305712795));
#31722=CARTESIAN_POINT('Ctrl Pts',(-2.93030502304087,-1.55204250277955,
-0.302449348443936));
#31723=CARTESIAN_POINT('Ctrl Pts',(-2.87165309834789,-1.32000917179155,
-1.12581972118214));
#31724=CARTESIAN_POINT('Ctrl Pts',(-2.77598800031732,0.0157677844803547,
-1.83790448190824));
#31725=CARTESIAN_POINT('Ctrl Pts',(-2.66494848030463,1.55180958399743,-0.984900257957451));
#31726=CARTESIAN_POINT('Ctrl Pts',(-2.55390896029194,1.66976418974896,0.768133489551486));
#31727=CARTESIAN_POINT('Ctrl Pts',(-2.44286944027925,0.261841363970268,
1.81922527888795));
#31728=CARTESIAN_POINT('Ctrl Pts',(-2.34221437831403,-1.23131260497695,
1.26503319844093));
#31729=CARTESIAN_POINT('Ctrl Pts',(-2.27857248968638,-1.55159413639811,
0.370750905089191));
#31730=CARTESIAN_POINT('Ctrl Pts',(-2.2519437743963,-1.55477365832743,-0.00137407056183876));
#31731=CARTESIAN_POINT('Origin',(-20.9400562256037,0.,0.));
#31732=CARTESIAN_POINT('',(-3.79005622560371,-1.55594287263106,-0.00137858150463178));
#31733=CARTESIAN_POINT('',(-3.6519437743963,-1.55727935086102,0.000957570549856082));
#31734=CARTESIAN_POINT('',(-20.9400562256037,-1.5555,1.83293981223255E-13));
#31735=CARTESIAN_POINT('Ctrl Pts',(-3.79005622560371,-1.55594287263106,
-0.00137858150463233));
#31736=CARTESIAN_POINT('Ctrl Pts',(-3.78248702979744,-1.55691314113539,
-0.106951986014344));
#31737=CARTESIAN_POINT('Ctrl Pts',(-3.7379046606536,-1.49901533715616,-0.727718784499475));
#31738=CARTESIAN_POINT('Ctrl Pts',(-3.6563091181722,-0.665127613333747,
-1.71340215497423));
#31739=CARTESIAN_POINT('Ctrl Pts',(-3.5452695981595,1.07748310522118,-1.48901707332687));
#31740=CARTESIAN_POINT('Ctrl Pts',(-3.43423007814681,1.83545949062223,0.0960736434662692));
#31741=CARTESIAN_POINT('Ctrl Pts',(-3.32319055813411,0.916141426756487,
1.59336956568948));
#31742=CARTESIAN_POINT('Ctrl Pts',(-3.21215103812143,-0.840372411640004,
1.63459961350804));
#31743=CARTESIAN_POINT('Ctrl Pts',(-3.13443959394462,-1.53221855341299,
0.618052683999356));
#31744=CARTESIAN_POINT('Ctrl Pts',(-3.09374132310538,-1.55776275391389,
0.0521469879633103));
#31745=CARTESIAN_POINT('Ctrl Pts',(-3.09005622560371,-1.55741714054868,
0.000874486562257217));
#31746=CARTESIAN_POINT('Ctrl Pts',(-3.6519437743963,-1.55727935086102,0.000957570549856073));
#31747=CARTESIAN_POINT('Ctrl Pts',(-3.61905072973292,-1.55396652622214,
-0.456805336982523));
#31748=CARTESIAN_POINT('Ctrl Pts',(-3.54914451173199,-1.09885245176768,
-1.43539894970098));
#31749=CARTESIAN_POINT('Ctrl Pts',(-3.44222512039348,0.563548452575144,
-1.74944409679311));
#31750=CARTESIAN_POINT('Ctrl Pts',(-3.3311856003808,1.77502341045502,-0.476899778205122));
#31751=CARTESIAN_POINT('Ctrl Pts',(-3.22014608036809,1.36443210709099,1.23144895602193));
#31752=CARTESIAN_POINT('Ctrl Pts',(-3.10910656035541,-0.293015589158281,
1.81446503711471));
#31753=CARTESIAN_POINT('Ctrl Pts',(-3.01970579169814,-1.41188410329576,
0.948880020508335));
#31754=CARTESIAN_POINT('Ctrl Pts',(-2.96731819637844,-1.55411623880003,
0.21606899395653));
#31755=CARTESIAN_POINT('Ctrl Pts',(-2.9519437743963,-1.5532548564925,0.000688385305712795));
#31756=CARTESIAN_POINT('Origin',(-20.9400562256037,0.,0.));
#31757=CARTESIAN_POINT('',(-4.4900562256037,-1.55296096245849,7.2602473186181E-5));
#31758=CARTESIAN_POINT('',(-4.3519437743963,-1.55612556903524,-0.00135081906484813));
#31759=CARTESIAN_POINT('',(-20.9400562256037,-1.5555,1.83293981223255E-13));
#31760=CARTESIAN_POINT('Ctrl Pts',(-4.4900562256037,-1.55296096245849,7.26024731861723E-5));
#31761=CARTESIAN_POINT('Ctrl Pts',(-4.47123273648949,-1.55285093046517,
-0.263750775239748));
#31762=CARTESIAN_POINT('Ctrl Pts',(-4.4153960740377,-1.36387406460508,-1.04648565772416));
#31763=CARTESIAN_POINT('Ctrl Pts',(-4.32254623824836,-0.123474165349735,
-1.83382000675687));
#31764=CARTESIAN_POINT('Ctrl Pts',(-4.21150671823566,1.4727595977204,-1.09960031557524));
#31765=CARTESIAN_POINT('Ctrl Pts',(-4.10046719822297,1.72314426360711,0.639465036955492));
#31766=CARTESIAN_POINT('Ctrl Pts',(-3.98942767821027,0.398871290133161,
1.79416927311721));
#31767=CARTESIAN_POINT('Ctrl Pts',(-3.88595735400385,-1.17478343605878,
1.34236238614872));
#31768=CARTESIAN_POINT('Ctrl Pts',(-3.819500203135,-1.55216855303728,0.409299254007138));
#31769=CARTESIAN_POINT('Ctrl Pts',(-3.79005622560371,-1.55594287263106,
-0.00137858150463233));
#31770=CARTESIAN_POINT('Ctrl Pts',(-4.3519437743963,-1.55612556903524,-0.00135081906484836));
#31771=CARTESIAN_POINT('Ctrl Pts',(-4.34480960976254,-1.55703324266528,
-0.100826422108305));
#31772=CARTESIAN_POINT('Ctrl Pts',(-4.30066227179122,-1.50305305182904,
-0.715415977812441));
#31773=CARTESIAN_POINT('Ctrl Pts',(-4.21950176048233,-0.685153134847353,
-1.70549309232754));
#31774=CARTESIAN_POINT('Ctrl Pts',(-4.10846224046965,1.0599664669302,-1.50153674452297));
#31775=CARTESIAN_POINT('Ctrl Pts',(-3.99742272045695,1.83645893175252,0.0745660657000111));
#31776=CARTESIAN_POINT('Ctrl Pts',(-3.88638320044426,0.93474362991831,1.5825283101715));
#31777=CARTESIAN_POINT('Ctrl Pts',(-3.77534368043157,-0.821166662308707,
1.64433172410147));
#31778=CARTESIAN_POINT('Ctrl Pts',(-3.69719720508225,-1.52881274645944,
0.630314108528291));
#31779=CARTESIAN_POINT('Ctrl Pts',(-3.65606390307049,-1.55769430982656,
0.0582961994486606));
#31780=CARTESIAN_POINT('Ctrl Pts',(-3.6519437743963,-1.55727935086102,0.000957570549856073));
#31781=CARTESIAN_POINT('Origin',(-20.9400562256037,0.,0.));
#31782=CARTESIAN_POINT('',(-5.1900562256037,-1.55620847966863,0.00133559623655165));
#31783=CARTESIAN_POINT('',(-5.05194377439629,-1.55295797459783,-2.70762857591493E-5));
#31784=CARTESIAN_POINT('',(-20.9400562256037,-1.5555,1.83293981223255E-13));
#31785=CARTESIAN_POINT('Ctrl Pts',(-5.1900562256037,-1.55620847966863,0.00133559623655161));
#31786=CARTESIAN_POINT('Ctrl Pts',(-5.15997844318154,-1.5524016656663,-0.417997969474535));
#31787=CARTESIAN_POINT('Ctrl Pts',(-5.0928874874218,-1.16138848763123,-1.35961338929137));
#31788=CARTESIAN_POINT('Ctrl Pts',(-4.98878335832452,0.429432903867215,
-1.78710074359752));
#31789=CARTESIAN_POINT('Ctrl Pts',(-4.87774383831181,1.73380656428109,-0.6099643303886));
#31790=CARTESIAN_POINT('Ctrl Pts',(-4.76670431829913,1.45377907542383,1.12457462471391));
#31791=CARTESIAN_POINT('Ctrl Pts',(-4.65566479828643,-0.154752576089497,
1.83144569312997));
#31792=CARTESIAN_POINT('Ctrl Pts',(-4.56344876738796,-1.37316082212235,
1.02857522543411));
#31793=CARTESIAN_POINT('Ctrl Pts',(-4.50824590982705,-1.5530672895693,0.255012794603092));
#31794=CARTESIAN_POINT('Ctrl Pts',(-4.4900562256037,-1.55296096245849,7.26024731861723E-5));
#31795=CARTESIAN_POINT('Ctrl Pts',(-5.05194377439629,-1.55295826129353,
-2.70732320311814E-5));
#31796=CARTESIAN_POINT('Ctrl Pts',(-5.03355531645459,-1.55299833977778,
-0.257754302019052));
#31797=CARTESIAN_POINT('Ctrl Pts',(-4.97815368517533,-1.37027115613983,
-1.03419383952361));
#31798=CARTESIAN_POINT('Ctrl Pts',(-4.8857388805585,-0.144947467941284,
-1.83224772825777));
#31799=CARTESIAN_POINT('Ctrl Pts',(-4.7746993605458,1.45977754246094,-1.11677707385809));
#31800=CARTESIAN_POINT('Ctrl Pts',(-4.66365984053311,1.73051682250325,0.619235846185912));
#31801=CARTESIAN_POINT('Ctrl Pts',(-4.55262032052042,0.419861211735448,
1.78937365271996));
#31802=CARTESIAN_POINT('Ctrl Pts',(-4.44871496514148,-1.16561614495599,
1.35420997741823));
#31803=CARTESIAN_POINT('Ctrl Pts',(-4.38182278310011,-1.55232408845772,
0.415268723900115));
#31804=CARTESIAN_POINT('Ctrl Pts',(-4.3519437743963,-1.55612556903524,-0.00135081906484836));
#31805=CARTESIAN_POINT('Origin',(-20.9400562256037,0.,0.));
#31806=CARTESIAN_POINT('',(-5.8900562256037,-1.55721324091966,-0.000993547179071312));
#31807=CARTESIAN_POINT('',(-5.75194377439629,-1.55602652096245,0.00136684493791416));
#31808=CARTESIAN_POINT('',(-20.9400562256037,-1.5555,1.83293981223255E-13));
#31809=CARTESIAN_POINT('Ctrl Pts',(-5.8900562256037,-1.55721324091966,-0.000993547179071299));
#31810=CARTESIAN_POINT('Ctrl Pts',(-5.88573732321115,-1.55766070941293,
-0.061105153849158));
#31811=CARTESIAN_POINT('Ctrl Pts',(-5.84440524748104,-1.52723085673784,
-0.635918540321862));
#31812=CARTESIAN_POINT('Ctrl Pts',(-5.76605999841336,-0.812353568509229,
-1.64870354109554));
#31813=CARTESIAN_POINT('Ctrl Pts',(-5.65502047840067,0.943200812016622,
-1.57750242944403));
#31814=CARTESIAN_POINT('Ctrl Pts',(-5.54398095838797,1.83683179154747,-0.0647352782582765));
#31815=CARTESIAN_POINT('Ctrl Pts',(-5.43294143837528,1.05191427466497,1.50718878892018));
#31816=CARTESIAN_POINT('Ctrl Pts',(-5.32190191836259,-0.694272059656186,
1.70180139671801));
#31817=CARTESIAN_POINT('Ctrl Pts',(-5.24094018077207,-1.50487070765057,
0.709796123886388));
#31818=CARTESIAN_POINT('Ctrl Pts',(-5.1969916165191,-1.55708626190928,0.0980263083819725));
#31819=CARTESIAN_POINT('Ctrl Pts',(-5.1900562256037,-1.55620847966863,0.00133559623655161));
#31820=CARTESIAN_POINT('Ctrl Pts',(-5.75194377439629,-1.55602652096245,
0.00136684493791428));
#31821=CARTESIAN_POINT('Ctrl Pts',(-5.72230102314664,-1.55223721629162,
-0.412026212646332));
#31822=CARTESIAN_POINT('Ctrl Pts',(-5.65564509855944,-1.17060922994658,
-1.34777943804002));
#31823=CARTESIAN_POINT('Ctrl Pts',(-5.55197600063464,0.408468929309301,
-1.79200854907483));
#31824=CARTESIAN_POINT('Ctrl Pts',(-5.44093648062197,1.726542296104,-0.630232660159929));
#31825=CARTESIAN_POINT('Ctrl Pts',(-5.32989696060926,1.46685280597546,1.1074675398269));
#31826=CARTESIAN_POINT('Ctrl Pts',(-5.21885744059658,-0.133287989090187,
1.83313278791599));
#31827=CARTESIAN_POINT('Ctrl Pts',(-5.12620637852558,-1.36680944890504,
1.04087016911624));
#31828=CARTESIAN_POINT('Ctrl Pts',(-5.07056848979215,-1.55291766787536,
0.261011470681804));
#31829=CARTESIAN_POINT('Ctrl Pts',(-5.05194377439629,-1.55295826129353,
-2.70732320311814E-5));
#31830=CARTESIAN_POINT('Origin',(-20.9400562256037,0.,0.));
#31831=CARTESIAN_POINT('',(-6.5900562256037,-1.55321890847038,-0.000648066932651872));
#31832=CARTESIAN_POINT('',(-6.45194377439629,-1.55735540394282,-0.000913172825708491));
#31833=CARTESIAN_POINT('',(-20.9400562256037,-1.5555,1.83293981223255E-13));
#31834=CARTESIAN_POINT('Ctrl Pts',(-6.5900562256037,-1.55321890847038,-0.000648066932651941));
#31835=CARTESIAN_POINT('Ctrl Pts',(-6.5744830299032,-1.55403921561424,-0.218825949717235));
#31836=CARTESIAN_POINT('Ctrl Pts',(-6.52189666086514,-1.40928295541454,
-0.954512421279383));
#31837=CARTESIAN_POINT('Ctrl Pts',(-6.43229711848952,-0.283299401454877,
-1.81600747130234));
#31838=CARTESIAN_POINT('Ctrl Pts',(-6.32125759847683,1.37100397883372,-1.22412817005115));
#31839=CARTESIAN_POINT('Ctrl Pts',(-6.21021807846413,1.77244540527444,0.486393844545889));
#31840=CARTESIAN_POINT('Ctrl Pts',(-6.09917855845144,0.55417642399643,1.75243549889208));
#31841=CARTESIAN_POINT('Ctrl Pts',(-5.9924579408313,-1.10343237309906,1.43009714852447));
#31842=CARTESIAN_POINT('Ctrl Pts',(-5.92275049654872,-1.5538258857936,0.454053818281797));
#31843=CARTESIAN_POINT('Ctrl Pts',(-5.8900562256037,-1.55721324091966,-0.000993547179071299));
#31844=CARTESIAN_POINT('Ctrl Pts',(-6.45194377439629,-1.55735540394282,
-0.000913172825708474));
#31845=CARTESIAN_POINT('Ctrl Pts',(-6.44805990317626,-1.55773235374386,
-0.0549569394560008));
#31846=CARTESIAN_POINT('Ctrl Pts',(-6.40716285861867,-1.53067193784369,
-0.623654417057565));
#31847=CARTESIAN_POINT('Ctrl Pts',(-6.3292526407235,-0.831611090304988,
-1.6390742816145));
#31848=CARTESIAN_POINT('Ctrl Pts',(-6.21821312071081,0.924656853680087,
-1.58844301412132));
#31849=CARTESIAN_POINT('Ctrl Pts',(-6.10717360069812,1.83594738678564,-0.0862478934429835));
#31850=CARTESIAN_POINT('Ctrl Pts',(-5.99613408068542,1.06949761739632,1.49476297537502));
#31851=CARTESIAN_POINT('Ctrl Pts',(-5.88509456067274,-0.674289122018889,
1.70981744232983));
#31852=CARTESIAN_POINT('Ctrl Pts',(-5.80369779190968,-1.50087042795734,
0.722096848042709));
#31853=CARTESIAN_POINT('Ctrl Pts',(-5.7593141964842,-1.55696869986509,0.104153569994228));
#31854=CARTESIAN_POINT('Ctrl Pts',(-5.75194377439629,-1.55602652096245,
0.00136684493791428));
#31855=CARTESIAN_POINT('Origin',(-20.9400562256037,0.,0.));
#31856=CARTESIAN_POINT('',(-7.29005622560369,-1.55485270523888,0.00138463193874137));
#31857=CARTESIAN_POINT('',(-7.15194377439629,-1.55330049259386,-0.00073539602550049));
#31858=CARTESIAN_POINT('',(-20.9400562256037,-1.5555,1.83293981223255E-13));
#31859=CARTESIAN_POINT('Ctrl Pts',(-7.29005622560369,-1.55485270523888,
0.00138463193874141));
#31860=CARTESIAN_POINT('Ctrl Pts',(-7.26322873659525,-1.55161198643692,
-0.373469770863784));
#31861=CARTESIAN_POINT('Ctrl Pts',(-7.19938807424924,-1.22747835831958,
-1.27052714563407));
#31862=CARTESIAN_POINT('Ctrl Pts',(-7.09853423856569,0.271575099355961,
-1.81779774785327));
#31863=CARTESIAN_POINT('Ctrl Pts',(-6.98749471855298,1.67385177993814,-0.75918502717621));
#31864=CARTESIAN_POINT('Ctrl Pts',(-6.8764551985403,1.54651567759537,0.993192300434498));
#31865=CARTESIAN_POINT('Ctrl Pts',(-6.7654156785276,0.00593010012215213,
1.83796260043647));
#31866=CARTESIAN_POINT('Ctrl Pts',(-6.6699493542154,-1.32324876481184,1.12023263145137));
#31867=CARTESIAN_POINT('Ctrl Pts',(-6.61149620324077,-1.55208957270924,
0.299722455455113));
#31868=CARTESIAN_POINT('Ctrl Pts',(-6.5900562256037,-1.55321890847038,-0.000648066932651941));
#31869=CARTESIAN_POINT('Ctrl Pts',(-7.15194377439629,-1.55330049259386,
-0.000735396025500611));
#31870=CARTESIAN_POINT('Ctrl Pts',(-7.13680560986831,-1.55420812252312,
-0.212790680832262));
#31871=CARTESIAN_POINT('Ctrl Pts',(-7.08465427200277,-1.41494999776031,
-0.942184803894316));
#31872=CARTESIAN_POINT('Ctrl Pts',(-6.99548976079967,-0.304553073520857,
-1.8125641868848));
#31873=CARTESIAN_POINT('Ctrl Pts',(-6.88445024078697,1.35657016098623,-1.24010439257756));
#31874=CARTESIAN_POINT('Ctrl Pts',(-6.77341072077428,1.77802146990873,0.465597636067849));
#31875=CARTESIAN_POINT('Ctrl Pts',(-6.66237120076158,0.574666806591611,
1.74582346403357));
#31876=CARTESIAN_POINT('Ctrl Pts',(-6.55521555196892,-1.09337608577705,
1.44169011708872));
#31877=CARTESIAN_POINT('Ctrl Pts',(-6.48507307651382,-1.55414003372731,
0.460078495237449));
#31878=CARTESIAN_POINT('Ctrl Pts',(-6.45194377439629,-1.55735540394282,
-0.000913172825708474));
#31879=CARTESIAN_POINT('Origin',(-20.9400562256037,0.,0.));
#31880=CARTESIAN_POINT('',(-7.9900562256037,-1.5579805623394,-0.000274378025309067));
#31881=CARTESIAN_POINT('',(-7.85194377439629,-1.55468095905983,0.00135958930439439));
#31882=CARTESIAN_POINT('',(-20.9400562256037,-1.5555,1.83293981223255E-13));
#31883=CARTESIAN_POINT('Ctrl Pts',(-7.9900562256037,-1.5579805623394,-0.000274378025309032));
#31884=CARTESIAN_POINT('Ctrl Pts',(-7.98898761662487,-1.55801680100739,
-0.015128171441536));
#31885=CARTESIAN_POINT('Ctrl Pts',(-7.95090583430849,-1.55110026292883,
-0.544434940735035));
#31886=CARTESIAN_POINT('Ctrl Pts',(-7.87581087865453,-0.953360544007956,
-1.57138326318549));
#31887=CARTESIAN_POINT('Ctrl Pts',(-7.76477135864184,0.80169783694629,-1.65391120224947));
#31888=CARTESIAN_POINT('Ctrl Pts',(-7.65373183862914,1.82414221101299,-0.225048618505586));
#31889=CARTESIAN_POINT('Ctrl Pts',(-7.54269231861645,1.17963418386913,1.40946971550936));
#31890=CARTESIAN_POINT('Ctrl Pts',(-7.43165279860376,-0.54285670200082,
1.75597502481768));
#31891=CARTESIAN_POINT('Ctrl Pts',(-7.34744076759951,-1.47296469184551,
0.801794893149571));
#31892=CARTESIAN_POINT('Ctrl Pts',(-7.30024190993282,-1.55608312000881,
0.143706882639392));
#31893=CARTESIAN_POINT('Ctrl Pts',(-7.29005622560369,-1.55485270523888,
0.00138463193874141));
#31894=CARTESIAN_POINT('Ctrl Pts',(-7.85194377439629,-1.55468095905983,
0.0013595893043942));
#31895=CARTESIAN_POINT('Ctrl Pts',(-7.82555131656036,-1.55157709491204,
-0.367519572225172));
#31896=CARTESIAN_POINT('Ctrl Pts',(-7.76214568538688,-1.23583930007717,
-1.2584972052081));
#31897=CARTESIAN_POINT('Ctrl Pts',(-7.66172688087582,0.250262368674325,
-1.82085426462248));
#31898=CARTESIAN_POINT('Ctrl Pts',(-7.55068736086313,1.66484362245829,-0.778740790589749));
#31899=CARTESIAN_POINT('Ctrl Pts',(-7.43964784085044,1.55804400070415,0.97500789639785));
#31900=CARTESIAN_POINT('Ctrl Pts',(-7.32860832083774,0.0274599982776329,
1.83776697507137));
#31901=CARTESIAN_POINT('Ctrl Pts',(-7.23270696535303,-1.3161301222519,1.13245711826584));
#31902=CARTESIAN_POINT('Ctrl Pts',(-7.17381878320588,-1.55198894569782,
0.305689548339082));
#31903=CARTESIAN_POINT('Ctrl Pts',(-7.15194377439629,-1.55330049259386,
-0.000735396025500611));
#31904=CARTESIAN_POINT('Origin',(-20.9400562256037,0.,0.));
#31905=CARTESIAN_POINT('',(-8.69005622560369,-1.55406204600757,-0.00119630707125469));
#31906=CARTESIAN_POINT('',(-8.55194377439629,-1.55801888457014,-0.000163493340269438));
#31907=CARTESIAN_POINT('',(-20.9400562256037,-1.5555,1.83293981223255E-13));
#31908=CARTESIAN_POINT('Ctrl Pts',(-8.6900562256037,-1.55406204600757,-0.00119630707125503));
#31909=CARTESIAN_POINT('Ctrl Pts',(-8.67773332331692,-1.55530151980103,
-0.173603109199959));
#31910=CARTESIAN_POINT('Ctrl Pts',(-8.62839724769259,-1.44936656402823,
-0.862372755859578));
#31911=CARTESIAN_POINT('Ctrl Pts',(-8.5420479987307,-0.44095583657419,-1.78429247515137));
#31912=CARTESIAN_POINT('Ctrl Pts',(-8.43100847871798,1.25875262728536,-1.33928470087313));
#31913=CARTESIAN_POINT('Ctrl Pts',(-8.31996895870532,1.8081775760136,0.329599059907972));
#31914=CARTESIAN_POINT('Ctrl Pts',(-8.2089294386926,0.705239055515858,1.69728593974785));
#31915=CARTESIAN_POINT('Ctrl Pts',(-8.09895852765874,-1.02535025064066,
1.51570965553032));
#31916=CARTESIAN_POINT('Ctrl Pts',(-8.02600078996244,-1.55676161026297,
0.499359392606125));
#31917=CARTESIAN_POINT('Ctrl Pts',(-7.9900562256037,-1.5579805623394,-0.000274378025309032));
#31918=CARTESIAN_POINT('Ctrl Pts',(-8.55194377439629,-1.55801888457014,
-0.0001634933402693));
#31919=CARTESIAN_POINT('Ctrl Pts',(-8.55131019658998,-1.55803205717942,
-0.00896971795875712));
#31920=CARTESIAN_POINT('Ctrl Pts',(-8.51366344544611,-1.5539786003993,-0.532216984914002));
#31921=CARTESIAN_POINT('Ctrl Pts',(-8.43900352096468,-0.971702639962959,
-1.56010752374873));
#31922=CARTESIAN_POINT('Ctrl Pts',(-8.32796400095197,0.782268521994644,
-1.66318894466765));
#31923=CARTESIAN_POINT('Ctrl Pts',(-8.2169244809393,1.82138073092891,-0.246401581101293));
#31924=CARTESIAN_POINT('Ctrl Pts',(-8.10588496092658,1.1960640567365,1.39555446986186));
#31925=CARTESIAN_POINT('Ctrl Pts',(-7.99484544091391,-0.522249555601089,
1.76221363853615));
#31926=CARTESIAN_POINT('Ctrl Pts',(-7.91019837873713,-1.46833344136842,
0.814121917015574));
#31927=CARTESIAN_POINT('Ctrl Pts',(-7.86256448989793,-1.55592999991363,
0.149802021359961));
#31928=CARTESIAN_POINT('Ctrl Pts',(-7.85194377439629,-1.55468095905983,
0.0013595893043942));
#31929=CARTESIAN_POINT('Origin',(-20.9400562256037,0.,0.));
#31930=CARTESIAN_POINT('',(-9.3900562256037,-1.55371612834885,0.00103887111830012));
#31931=CARTESIAN_POINT('',(-9.25194377439629,-1.55421089288766,-0.00124746091003075));
#31932=CARTESIAN_POINT('',(-20.9400562256037,-1.5555,1.83293981223255E-13));
#31933=CARTESIAN_POINT('Ctrl Pts',(-9.3900562256037,-1.55371612834885,0.00103887111830016));
#31934=CARTESIAN_POINT('Ctrl Pts',(-9.36647903000898,-1.55168635657405,
-0.329008869350852));
#31935=CARTESIAN_POINT('Ctrl Pts',(-9.3058886610767,-1.28725468228538,-1.18016031646684));
#31936=CARTESIAN_POINT('Ctrl Pts',(-9.20828511880685,0.111638249353674,
-1.83457858593517));
#31937=CARTESIAN_POINT('Ctrl Pts',(-9.09724559879415,1.60108280900731,-0.902593776508504));
#31938=CARTESIAN_POINT('Ctrl Pts',(-8.98620607878146,1.62741291579734,0.854206584022058));
#31939=CARTESIAN_POINT('Ctrl Pts',(-8.87516655876877,0.166567378401736,
1.83040896936805));
#31940=CARTESIAN_POINT('Ctrl Pts',(-8.77644994104285,-1.26747859705886,
1.21122555034046));
#31941=CARTESIAN_POINT('Ctrl Pts',(-8.71474649665449,-1.55157862585143,
0.344239417119107));
#31942=CARTESIAN_POINT('Ctrl Pts',(-8.6900562256037,-1.55406204600757,-0.00119630707125503));
#31943=CARTESIAN_POINT('Ctrl Pts',(-9.25194377439629,-1.55421089288766,
-0.00124746091003079));
#31944=CARTESIAN_POINT('Ctrl Pts',(-9.24005590328203,-1.55546589319888,
-0.167527666085323));
#31945=CARTESIAN_POINT('Ctrl Pts',(-9.19115485883021,-1.4543434475797,-0.850039222709116));
#31946=CARTESIAN_POINT('Ctrl Pts',(-9.10524064104083,-0.461827170446667,
-1.77900454490864));
#31947=CARTESIAN_POINT('Ctrl Pts',(-8.99420112102814,1.24297754506556,-1.35393808153518));
#31948=CARTESIAN_POINT('Ctrl Pts',(-8.88316160101544,1.81191445877564,0.308395039272923));
#31949=CARTESIAN_POINT('Ctrl Pts',(-8.77212208100275,0.725073034805075,
1.68890810891739));
#31950=CARTESIAN_POINT('Ctrl Pts',(-8.66171613879637,-1.01437844712226,
1.5269787503532));
#31951=CARTESIAN_POINT('Ctrl Pts',(-8.58832336992754,-1.55726252253713,
0.505483779320834));
#31952=CARTESIAN_POINT('Ctrl Pts',(-8.55194377439629,-1.55801888457014,
-0.0001634933402693));
#31953=CARTESIAN_POINT('Origin',(-20.9400562256037,0.,0.));
#31954=CARTESIAN_POINT('',(-10.0900562256037,-1.55780423998256,0.000547110510323483));
#31955=CARTESIAN_POINT('',(-9.95194377439629,-1.5535960288726,0.000967876971002882));
#31956=CARTESIAN_POINT('',(-20.9400562256037,-1.5555,1.83293981223255E-13));
#31957=CARTESIAN_POINT('Ctrl Pts',(-10.0900562256037,-1.55780423998256,
0.000547110510323474));
#31958=CARTESIAN_POINT('Ctrl Pts',(-10.055224736701,-1.55559939196281,-0.483761196717675));
#31959=CARTESIAN_POINT('Ctrl Pts',(-9.98338007446081,-1.05285972037605,
-1.48666276859663));
#31960=CARTESIAN_POINT('Ctrl Pts',(-9.874522238883,0.654057457242615,-1.71765844372971));
#31961=CARTESIAN_POINT('Ctrl Pts',(-9.76348271887031,1.79748789421279,-0.38363909713309));
#31962=CARTESIAN_POINT('Ctrl Pts',(-9.65244319885762,1.29832339351032,1.30096043466144));
#31963=CARTESIAN_POINT('Ctrl Pts',(-9.54140367884492,-0.387285500229918,
1.79670577112734));
#31964=CARTESIAN_POINT('Ctrl Pts',(-9.45394135442695,-1.43622080995592,
0.893931513220443));
#31965=CARTESIAN_POINT('Ctrl Pts',(-9.40349220334654,-1.55487283794477,
0.18912375497161));
#31966=CARTESIAN_POINT('Ctrl Pts',(-9.3900562256037,-1.55371612834885,0.00103887111830016));
#31967=CARTESIAN_POINT('Ctrl Pts',(-9.95194377439629,-1.5535960288726,0.000967876971002899));
#31968=CARTESIAN_POINT('Ctrl Pts',(-9.92880160997409,-1.55174879348202,
-0.323052877225753));
#31969=CARTESIAN_POINT('Ctrl Pts',(-9.86864627221432,-1.29479054227638,
-1.16798978252056));
#31970=CARTESIAN_POINT('Ctrl Pts',(-9.77147776111699,0.0901399223399556,
-1.83576041480606));
#31971=CARTESIAN_POINT('Ctrl Pts',(-9.66043824110429,1.59039972425115,-0.921287264250532));
#31972=CARTESIAN_POINT('Ctrl Pts',(-9.54939872109161,1.63730757628732,0.835084071696088));
#31973=CARTESIAN_POINT('Ctrl Pts',(-9.4383592010789,0.187997765394267,1.82833212146347));
#31974=CARTESIAN_POINT('Ctrl Pts',(-9.33920755218048,-1.25955421209835,
1.22333549611273));
#31975=CARTESIAN_POINT('Ctrl Pts',(-9.2770690766196,-1.55155841947111,0.350189761838226));
#31976=CARTESIAN_POINT('Ctrl Pts',(-9.25194377439629,-1.55421089288766,
-0.00124746091003079));
#31977=CARTESIAN_POINT('Origin',(-20.9400562256037,0.,0.));
#31978=CARTESIAN_POINT('',(-10.7900562256037,-1.55530876292539,-0.00141549567407365));
#31979=CARTESIAN_POINT('',(-10.6519437743963,-1.55770803555897,0.000647550266795888));
#31980=CARTESIAN_POINT('',(-20.9400562256037,-1.5555,1.83293981223255E-13));
#31981=CARTESIAN_POINT('Ctrl Pts',(-10.7900562256037,-1.55530876292539,
-0.00141549567407357));
#31982=CARTESIAN_POINT('Ctrl Pts',(-10.7809836167307,-1.55645685696222,
-0.128090375998343));
#31983=CARTESIAN_POINT('Ctrl Pts',(-10.73489783452,-1.48442131297674,-0.770267129004551));
#31984=CARTESIAN_POINT('Ctrl Pts',(-10.6517988789718,-0.595236530522984,
-1.73891781272768));
#31985=CARTESIAN_POINT('Ctrl Pts',(-10.5407593589592,1.1368648842552,-1.44418832623659));
#31986=CARTESIAN_POINT('Ctrl Pts',(-10.4297198389465,1.83006722788652,0.170281026853745));
#31987=CARTESIAN_POINT('Ctrl Pts',(-10.3186803189338,0.850902723426497,
1.62914279360528));
#31988=CARTESIAN_POINT('Ctrl Pts',(-10.2076407989211,-0.905840595584799,
1.59924810522983));
#31989=CARTESIAN_POINT('Ctrl Pts',(-10.1314327678111,-1.54339980391117,
0.575724981289948));
#31990=CARTESIAN_POINT('Ctrl Pts',(-10.0922379100386,-1.55794234153255,
0.0308819577665884));
#31991=CARTESIAN_POINT('Ctrl Pts',(-10.0900562256037,-1.55780423998256,
0.000547110510323474));
#31992=CARTESIAN_POINT('Ctrl Pts',(-10.6519437743963,-1.55770803555897,
0.000647550266795966));
#31993=CARTESIAN_POINT('Ctrl Pts',(-10.6175473166661,-1.55519061705744,
-0.47769039247032));
#31994=CARTESIAN_POINT('Ctrl Pts',(-10.5461376855984,-1.06339243988215,
-1.47523026632046));
#31995=CARTESIAN_POINT('Ctrl Pts',(-10.4377148811931,0.633891526962291,
-1.72520231805252));
#31996=CARTESIAN_POINT('Ctrl Pts',(-10.3266753611805,1.79287047934082,-0.404668939352399));
#31997=CARTESIAN_POINT('Ctrl Pts',(-10.2156358411678,1.31347401748173,1.28566228519341));
#31998=CARTESIAN_POINT('Ctrl Pts',(-10.1045963211551,-0.366211903252911,
1.8011191931919));
#31999=CARTESIAN_POINT('Ctrl Pts',(-10.0166989655646,-1.43092008288472,
0.906265457554098));
#32000=CARTESIAN_POINT('Ctrl Pts',(-9.96581478331166,-1.55470322948288,
0.195180254354059));
#32001=CARTESIAN_POINT('Ctrl Pts',(-9.95194377439629,-1.5535960288726,0.000967876971002899));
#32002=CARTESIAN_POINT('Origin',(-20.9400562256037,0.,0.));
#32003=CARTESIAN_POINT('',(-11.4900562256037,-1.55305926288001,0.00041138631351628));
#32004=CARTESIAN_POINT('',(-11.3519437743963,-1.55549132498077,-0.00141421151383214));
#32005=CARTESIAN_POINT('',(-20.9400562256037,-1.5555,1.83293981223255E-13));
#32006=CARTESIAN_POINT('Ctrl Pts',(-11.4900562256037,-1.55305926288001,
0.000411386313516286));
#32007=CARTESIAN_POINT('Ctrl Pts',(-11.4697293234227,-1.55238359018918,
-0.284438289989754));
#32008=CARTESIAN_POINT('Ctrl Pts',(-11.4123892479042,-1.34098631575837,
-1.08890284854511));
#32009=CARTESIAN_POINT('Ctrl Pts',(-11.318035999048,-0.0491532482193918,
-1.83731479199404));
#32010=CARTESIAN_POINT('Ctrl Pts',(-11.2069964790353,1.51605673496666,-1.03909271148097));
#32011=CARTESIAN_POINT('Ctrl Pts',(-11.0959569590226,1.69585148053222,0.708681481814863));
#32012=CARTESIAN_POINT('Ctrl Pts',(-10.9849174390099,0.325929498694267,
1.80884262681183));
#32013=CARTESIAN_POINT('Ctrl Pts',(-10.8829505278703,-1.20556935877834,
1.30120052871543));
#32014=CARTESIAN_POINT('Ctrl Pts',(-10.8179967900682,-1.55177302189475,
0.388700259260363));
#32015=CARTESIAN_POINT('Ctrl Pts',(-10.7900562256037,-1.55530876292539,
-0.00141549567407357));
#32016=CARTESIAN_POINT('Ctrl Pts',(-11.3519437743963,-1.55549132498077,
-0.00141421151383192));
#32017=CARTESIAN_POINT('Ctrl Pts',(-11.3433061966958,-1.55659501205107,
-0.121978863546162));
#32018=CARTESIAN_POINT('Ctrl Pts',(-11.2976554456577,-1.48874725562481,
-0.757950576461866));
#32019=CARTESIAN_POINT('Ctrl Pts',(-11.214991521282,-0.615565745527372,
-1.73182571845486));
#32020=CARTESIAN_POINT('Ctrl Pts',(-11.1039520012693,1.11986930393965,-1.45740668595354));
#32021=CARTESIAN_POINT('Ctrl Pts',(-10.9929124812566,1.83193632103844,0.148831521622652));
#32022=CARTESIAN_POINT('Ctrl Pts',(-10.8818729612439,0.869928460211977,
1.61906330335833));
#32023=CARTESIAN_POINT('Ctrl Pts',(-10.7708334412312,-0.887044467963301,
1.60974955133526));
#32024=CARTESIAN_POINT('Ctrl Pts',(-10.6941903789487,-1.54025737311525,
0.587965478802919));
#32025=CARTESIAN_POINT('Ctrl Pts',(-10.6545604900037,-1.55789954854368,
0.0370371799838544));
#32026=CARTESIAN_POINT('Ctrl Pts',(-10.6519437743963,-1.55770803555897,
0.000647550266795966));
#32027=CARTESIAN_POINT('Origin',(-20.9400562256037,0.,0.));
#32028=CARTESIAN_POINT('',(-12.1900562256037,-1.5568114087742,0.00117013613562253));
#32029=CARTESIAN_POINT('',(-12.0519437743963,-1.55301668366533,0.00031493299472482));
#32030=CARTESIAN_POINT('',(-20.9400562256037,-1.5555,1.83293981223255E-13));
#32031=CARTESIAN_POINT('Ctrl Pts',(-12.1900562256037,-1.5568114087742,0.00117013613562249));
#32032=CARTESIAN_POINT('Ctrl Pts',(-12.1584750301148,-1.55312521236765,
-0.4386816463206));
#32033=CARTESIAN_POINT('Ctrl Pts',(-12.0898806612882,-1.12861437631865,
-1.4002653092897));
#32034=CARTESIAN_POINT('Ctrl Pts',(-11.9842731191242,0.501409935092548,
-1.76825613633351));
#32035=CARTESIAN_POINT('Ctrl Pts',(-11.8732335991115,1.75707289349663,-0.539292623378071));
#32036=CARTESIAN_POINT('Ctrl Pts',(-11.7621940790988,1.40707327733112,1.18249164010207));
#32037=CARTESIAN_POINT('Ctrl Pts',(-11.6511545590861,-0.228749431006459,
1.82368182107101));
#32038=CARTESIAN_POINT('Ctrl Pts',(-11.5604419412544,-1.39434711281995,
0.986039404245019));
#32039=CARTESIAN_POINT('Ctrl Pts',(-11.5067424967603,-1.55361391983816,
0.234243324664662));
#32040=CARTESIAN_POINT('Ctrl Pts',(-11.4900562256037,-1.55305926288001,
0.000411386313516286));
#32041=CARTESIAN_POINT('Ctrl Pts',(-12.0519437743963,-1.55301668366533,
0.000314932994724976));
#32042=CARTESIAN_POINT('Ctrl Pts',(-12.0320519033878,-1.55251128218854,
-0.278457518785902));
#32043=CARTESIAN_POINT('Ctrl Pts',(-11.9751468590418,-1.34773454330521,
-1.07663970368379));
#32044=CARTESIAN_POINT('Ctrl Pts',(-11.8812286413582,-0.0706725909392507,
-1.83661288546561));
#32045=CARTESIAN_POINT('Ctrl Pts',(-11.7701891213455,1.50378050738072,-1.05678081539653));
#32046=CARTESIAN_POINT('Ctrl Pts',(-11.6591496013328,1.70403672974556,0.688767253755881));
#32047=CARTESIAN_POINT('Ctrl Pts',(-11.5481100813201,0.34709631401335,1.80490045569464));
#32048=CARTESIAN_POINT('Ctrl Pts',(-11.4457081390079,-1.19680295565656,
1.31314440998192));
#32049=CARTESIAN_POINT('Ctrl Pts',(-11.3803193700333,-1.55186556564147,
0.394656762641098));
#32050=CARTESIAN_POINT('Ctrl Pts',(-11.3519437743963,-1.55549132498077,
-0.00141421151383192));
#32051=CARTESIAN_POINT('Origin',(-20.9400562256037,0.,0.));
#32052=CARTESIAN_POINT('',(-12.8900562256037,-1.55666010321292,-0.00122146201820818));
#32053=CARTESIAN_POINT('',(-12.7519437743963,-1.55664245885653,0.00122697214749692));
#32054=CARTESIAN_POINT('',(-20.9400562256037,-1.5555,1.83293981223255E-13));
#32055=CARTESIAN_POINT('Ctrl Pts',(-12.8900562256037,-1.55666010321292,
-0.00122146201820782));
#32056=CARTESIAN_POINT('Ctrl Pts',(-12.8842339101444,-1.55735948147068,
-0.0823331232632712));
#32057=CARTESIAN_POINT('Ctrl Pts',(-12.8413984213475,-1.51473567899467,
-0.678344946172016));
#32058=CARTESIAN_POINT('Ctrl Pts',(-12.761549759213,-0.744960386131938,
-1.68023085014673));
#32059=CARTESIAN_POINT('Ctrl Pts',(-12.6505102392003,1.00627386240032,-1.53803595554219));
#32060=CARTESIAN_POINT('Ctrl Pts',(-12.5394707191877,1.83794678447648,0.00965940594506788));
#32061=CARTESIAN_POINT('Ctrl Pts',(-12.4284311991749,0.990052298275348,
1.5485277309013));
#32062=CARTESIAN_POINT('Ctrl Pts',(-12.3173916791622,-0.762579793343959,
1.67230790988804));
#32063=CARTESIAN_POINT('Ctrl Pts',(-12.2379333546385,-1.5180706132219,0.667323369933976));
#32064=CARTESIAN_POINT('Ctrl Pts',(-12.1954882034523,-1.55744543598299,
0.0768248129769098));
#32065=CARTESIAN_POINT('Ctrl Pts',(-12.1900562256037,-1.5568114087742,0.00117013613562249));
#32066=CARTESIAN_POINT('Ctrl Pts',(-12.7519437743963,-1.55664245885653,
0.00122697214749681));
#32067=CARTESIAN_POINT('Ctrl Pts',(-12.7207976100799,-1.55289025223912,
-0.432688241818353));
#32068=CARTESIAN_POINT('Ctrl Pts',(-12.6526382724259,-1.13824355650797,
-1.38854277671179));
#32069=CARTESIAN_POINT('Ctrl Pts',(-12.5474657614343,0.480661769934936,
-1.77400839036668));
#32070=CARTESIAN_POINT('Ctrl Pts',(-12.4364262414216,1.75063489249572,-0.559838351084378));
#32071=CARTESIAN_POINT('Ctrl Pts',(-12.3253867214089,1.42082866667544,1.16592770192737));
#32072=CARTESIAN_POINT('Ctrl Pts',(-12.2143472013962,-0.207370712553722,
1.82623626449135));
#32073=CARTESIAN_POINT('Ctrl Pts',(-12.123199552392,-1.38833725657031,0.998354084754823));
#32074=CARTESIAN_POINT('Ctrl Pts',(-12.0690650767254,-1.55345169209053,
0.240259552880984));
#32075=CARTESIAN_POINT('Ctrl Pts',(-12.0519437743963,-1.55301668366533,
0.000314932994724976));
#32076=CARTESIAN_POINT('Origin',(-20.9400562256037,0.,0.));
#32077=CARTESIAN_POINT('',(-13.5900562256037,-1.55302057111372,-0.000324920039265338));
#32078=CARTESIAN_POINT('',(-13.4519437743963,-1.55682839314694,-0.00116389690534152));
#32079=CARTESIAN_POINT('',(-20.9400562256037,-1.5555,1.83293981223255E-13));
#32080=CARTESIAN_POINT('Ctrl Pts',(-13.5900562256037,-1.55302057111372,
-0.000324920039265191));
#32081=CARTESIAN_POINT('Ctrl Pts',(-13.5729796168364,-1.55346826531772,
-0.239641713856127));
#32082=CARTESIAN_POINT('Ctrl Pts',(-13.5188898347316,-1.38895922343596,
-0.997089159776875));
#32083=CARTESIAN_POINT('Ctrl Pts',(-13.4277868792892,-0.209568452681189,
-1.82598541898106));
#32084=CARTESIAN_POINT('Ctrl Pts',(-13.3167473592765,1.4194244756517,-1.1676368633319));
#32085=CARTESIAN_POINT('Ctrl Pts',(-13.2057078392638,1.75130743978355,0.557731062474938));
#32086=CARTESIAN_POINT('Ctrl Pts',(-13.0946683192511,0.482796462927691,
1.77342867408733));
#32087=CARTESIAN_POINT('Ctrl Pts',(-12.9894511146977,-1.13725980242033,
1.38974871282814));
#32088=CARTESIAN_POINT('Ctrl Pts',(-12.9212470834819,-1.55291344812471,
0.433303653605542));
#32089=CARTESIAN_POINT('Ctrl Pts',(-12.8900562256037,-1.55666010321292,
-0.00122146201820782));
#32090=CARTESIAN_POINT('Ctrl Pts',(-13.4519437743963,-1.55682839314694,
-0.00116389690534121));
#32091=CARTESIAN_POINT('Ctrl Pts',(-13.4465564901095,-1.55745489713643,
-0.0761939586894047));
#32092=CARTESIAN_POINT('Ctrl Pts',(-13.4041560324851,-1.51844833398138,
-0.666061655826624));
#32093=CARTESIAN_POINT('Ctrl Pts',(-13.3247424015232,-0.764591851789241,
-1.67138888543208));
#32094=CARTESIAN_POINT('Ctrl Pts',(-13.2137028815105,0.988187893799185,
-1.54971810104841));
#32095=CARTESIAN_POINT('Ctrl Pts',(-13.1026633614978,1.83793377915969,-0.0118713770116975));
#32096=CARTESIAN_POINT('Ctrl Pts',(-12.9916238414851,1.00812414086676,1.53682374486147));
#32097=CARTESIAN_POINT('Ctrl Pts',(-12.8805843214724,-0.742937660327962,
1.68112615202868));
#32098=CARTESIAN_POINT('Ctrl Pts',(-12.8006909657761,-1.51434968958816,
0.679607163890773));
#32099=CARTESIAN_POINT('Ctrl Pts',(-12.7578107834174,-1.55734926274576,
0.08296366527229));
#32100=CARTESIAN_POINT('Ctrl Pts',(-12.7519437743963,-1.55664245885653,
0.00122697214749681));
#32101=CARTESIAN_POINT('Origin',(-20.9400562256037,0.,0.));
#32102=CARTESIAN_POINT('',(-14.2900562256037,-1.55547253832405,0.0014146944387468));
#32103=CARTESIAN_POINT('',(-14.1519437743963,-1.55306423282011,-0.000421191186355668));
#32104=CARTESIAN_POINT('',(-20.9400562256037,-1.5555,1.83293981223255E-13));
#32105=CARTESIAN_POINT('Ctrl Pts',(-14.2900562256037,-1.55547253832405,
0.00141469443874675));
#32106=CARTESIAN_POINT('Ctrl Pts',(-14.2617253235285,-1.55185529681908,
-0.394044692501087));
#32107=CARTESIAN_POINT('Ctrl Pts',(-14.1963812481157,-1.19770891737767,
-1.31191857440859));
#32108=CARTESIAN_POINT('Ctrl Pts',(-14.0940239993653,0.344923864904767,
-1.8053169289933));
#32109=CARTESIAN_POINT('Ctrl Pts',(-13.9829844793526,1.70320660624744,-0.690817590341849));
#32110=CARTESIAN_POINT('Ctrl Pts',(-13.8719449593399,1.50505129966774,1.05497027069917));
#32111=CARTESIAN_POINT('Ctrl Pts',(-13.7609054393273,-0.0684621685615409,
1.83669665926807));
#32112=CARTESIAN_POINT('Ctrl Pts',(-13.6669425280818,-1.34704602164299,
1.07790003576514));
#32113=CARTESIAN_POINT('Ctrl Pts',(-13.609992790174,-1.5524978979924,0.279072165043973));
#32114=CARTESIAN_POINT('Ctrl Pts',(-13.5900562256037,-1.55302057111372,
-0.000324920039265191));
#32115=CARTESIAN_POINT('Ctrl Pts',(-14.1519437743963,-1.55306423282011,
-0.000421191186355634));
#32116=CARTESIAN_POINT('Ctrl Pts',(-14.1353021968015,-1.5536306920086,-0.233624933925084));
#32117=CARTESIAN_POINT('Ctrl Pts',(-14.0816474458692,-1.39495898335225,
-0.984773952170566));
#32118=CARTESIAN_POINT('Ctrl Pts',(-13.9909795215993,-0.230944069595307,
-1.82340515050471));
#32119=CARTESIAN_POINT('Ctrl Pts',(-13.8799400015866,1.40564908600105,-1.18418417199048));
#32120=CARTESIAN_POINT('Ctrl Pts',(-13.7689004815739,1.75772061547503,0.537177572225828));
#32121=CARTESIAN_POINT('Ctrl Pts',(-13.6578609615613,0.503537663837979,
1.76765135908215));
#32122=CARTESIAN_POINT('Ctrl Pts',(-13.5522087258354,-1.12761832251555,
1.40146764598756));
#32123=CARTESIAN_POINT('Ctrl Pts',(-13.483569663447,-1.5531505204737,0.439297805712299));
#32124=CARTESIAN_POINT('Ctrl Pts',(-13.4519437743963,-1.55682839314694,
-0.00116389690534121));
#32125=CARTESIAN_POINT('Origin',(-20.9400562256037,0.,0.));
#32126=CARTESIAN_POINT('',(-14.9900562256037,-1.55771859828449,-0.000637424228261111));
#32127=CARTESIAN_POINT('',(-14.8519437743963,-1.55529006138918,0.00141519769127213));
#32128=CARTESIAN_POINT('',(-20.9400562256037,-1.5555,1.83293981223255E-13));
#32129=CARTESIAN_POINT('Ctrl Pts',(-14.9900562256037,-1.55771859828449,
-0.000637424228261464));
#32130=CARTESIAN_POINT('Ctrl Pts',(-14.9874842035581,-1.55790433195692,
-0.0364048781015495));
#32131=CARTESIAN_POINT('Ctrl Pts',(-14.9478990081749,-1.54058372170137,
-0.586707661205107));
#32132=CARTESIAN_POINT('Ctrl Pts',(-14.8713006394542,-0.888981191146498,
-1.60868086595148));
#32133=CARTESIAN_POINT('Ctrl Pts',(-14.7602611194415,0.867979302403128,
-1.62010913746279));
#32134=CARTESIAN_POINT('Ctrl Pts',(-14.6492215994288,1.83175592377073,-0.151036162628272));
#32135=CARTESIAN_POINT('Ctrl Pts',(-14.5381820794161,1.12162251930453,1.4560579009365));
#32136=CARTESIAN_POINT('Ctrl Pts',(-14.4271425594034,-0.613481054986446,
1.73256534706872));
#32137=CARTESIAN_POINT('Ctrl Pts',(-14.3444339414659,-1.48830675260198,
0.759215790299635));
#32138=CARTESIAN_POINT('Ctrl Pts',(-14.298738496866,-1.5565810759867,0.122606941036985));
#32139=CARTESIAN_POINT('Ctrl Pts',(-14.2900562256037,-1.55547253832405,
0.00141469443874675));
#32140=CARTESIAN_POINT('Ctrl Pts',(-14.8519437743963,-1.55529006138918,
0.00141519769127204));
#32141=CARTESIAN_POINT('Ctrl Pts',(-14.8240479034936,-1.5517644390058,-0.388088446331793));
#32142=CARTESIAN_POINT('Ctrl Pts',(-14.7591388592533,-1.20646344528897,
-1.29997195727927));
#32143=CARTESIAN_POINT('Ctrl Pts',(-14.6572166416755,0.323752302625325,
-1.80923352630697));
#32144=CARTESIAN_POINT('Ctrl Pts',(-14.5461771216628,1.6949973052892,-0.71072191554133));
#32145=CARTESIAN_POINT('Ctrl Pts',(-14.4351376016501,1.51730614988444,1.03726734918786));
#32146=CARTESIAN_POINT('Ctrl Pts',(-14.3240980816374,-0.0469419935946381,
1.8373725684808));
#32147=CARTESIAN_POINT('Ctrl Pts',(-14.2297001392195,-1.34028715463676,
1.09016214116502));
#32148=CARTESIAN_POINT('Ctrl Pts',(-14.1723153701391,-1.55237080832191,
0.285052487359556));
#32149=CARTESIAN_POINT('Ctrl Pts',(-14.1519437743963,-1.55306423282011,
-0.000421191186355634));
#32150=CARTESIAN_POINT('Origin',(-20.9400562256037,0.,0.));
#32151=CARTESIAN_POINT('',(-15.6900562256037,-1.55360798640993,-0.000975396588764602));
#32152=CARTESIAN_POINT('',(-15.5519437743963,-1.55781326646842,-0.000536565987746263));
#32153=CARTESIAN_POINT('',(-20.9400562256037,-1.5555,1.83293981223255E-13));
#32154=CARTESIAN_POINT('Ctrl Pts',(-15.6900562256037,-1.55360798640993,
-0.000975396588764697));
#32155=CARTESIAN_POINT('Ctrl Pts',(-15.6762299102502,-1.55472072171226,
-0.194558284943319));
#32156=CARTESIAN_POINT('Ctrl Pts',(-15.625390421559,-1.43146895103288,-0.904998367253485));
#32157=CARTESIAN_POINT('Ctrl Pts',(-15.5375377595304,-0.368379304064812,
-1.80067719900824));
#32158=CARTESIAN_POINT('Ctrl Pts',(-15.4264982395177,1.31192580014841,-1.28724216120951));
#32159=CARTESIAN_POINT('Ctrl Pts',(-15.315458719505,1.79335624998195,0.402510928225848));
#32160=CARTESIAN_POINT('Ctrl Pts',(-15.2044191994923,0.635967374718456,
1.72443822301191));
#32161=CARTESIAN_POINT('Ctrl Pts',(-15.0959517015252,-1.06231602123872,
1.47640683538839));
#32162=CARTESIAN_POINT('Ctrl Pts',(-15.0244973768957,-1.5552314961529,0.478313482231629));
#32163=CARTESIAN_POINT('Ctrl Pts',(-14.9900562256037,-1.55771859828449,
-0.000637424228261464));
#32164=CARTESIAN_POINT('Ctrl Pts',(-15.5519437743963,-1.55781326646842,
-0.000536565987745981));
#32165=CARTESIAN_POINT('Ctrl Pts',(-15.5498067835232,-1.55794626072305,
-0.0302495182367311));
#32166=CARTESIAN_POINT('Ctrl Pts',(-15.5106566193126,-1.54371834758075,
-0.574467772409033));
#32167=CARTESIAN_POINT('Ctrl Pts',(-15.4344932817643,-0.907764618603845,
-1.59815672053134));
#32168=CARTESIAN_POINT('Ctrl Pts',(-15.3234537617517,0.848941402803422,
-1.63016563599362));
#32169=CARTESIAN_POINT('Ctrl Pts',(-15.212414241739,1.82986091954754,-0.172483394218017));
#32170=CARTESIAN_POINT('Ctrl Pts',(-15.1013747217263,1.13860211855666,1.4428190190688));
#32171=CARTESIAN_POINT('Ctrl Pts',(-14.9903352017136,-0.593143287092892,
1.7396328771166));
#32172=CARTESIAN_POINT('Ctrl Pts',(-14.9071915526036,-1.48397203957219,
0.771532660500938));
#32173=CARTESIAN_POINT('Ctrl Pts',(-14.8610610768312,-1.55644235255271,
0.128717999400674));
#32174=CARTESIAN_POINT('Ctrl Pts',(-14.8519437743963,-1.55529006138918,
0.00141519769127204));
#32175=CARTESIAN_POINT('Origin',(-20.9400562256037,0.,0.));
#32176=CARTESIAN_POINT('',(-16.3900562256037,-1.55419531422885,0.00124249107025136));
#32177=CARTESIAN_POINT('',(-16.2519437743963,-1.55372892642411,-0.00104588007964812));
#32178=CARTESIAN_POINT('',(-20.9400562256037,-1.5555,1.83293981223255E-13));
#32179=CARTESIAN_POINT('Ctrl Pts',(-16.3900562256037,-1.55419531422885,
0.00124249107025116));
#32180=CARTESIAN_POINT('Ctrl Pts',(-16.3649756169422,-1.55155993342647,
-0.349578491669034));
#32181=CARTESIAN_POINT('Ctrl Pts',(-16.3028818349431,-1.26037345479531,
-1.22209225599236));
#32182=CARTESIAN_POINT('Ctrl Pts',(-16.2037748796065,0.185797227123519,
-1.82855710250446));
#32183=CARTESIAN_POINT('Ctrl Pts',(-16.0927353595938,1.63630140628791,-0.837053997341315));
#32184=CARTESIAN_POINT('Ctrl Pts',(-15.9816958395811,1.59150738893344,0.919372567381872));
#32185=CARTESIAN_POINT('Ctrl Pts',(-15.8706563195684,0.0923492065994037,
1.83565065051508));
#32186=CARTESIAN_POINT('Ctrl Pts',(-15.7734431149093,-1.29402133831582,
1.16924087449169));
#32187=CARTESIAN_POINT('Ctrl Pts',(-15.7132430835877,-1.55174191907607,
0.323664887220352));
#32188=CARTESIAN_POINT('Ctrl Pts',(-15.6900562256037,-1.55360798640993,
-0.000975396588764697));
#32189=CARTESIAN_POINT('Ctrl Pts',(-16.2519437743963,-1.55372892642411,
-0.00104588007964796));
#32190=CARTESIAN_POINT('Ctrl Pts',(-16.2385524902153,-1.55489017216451,
-0.188501220428145));
#32191=CARTESIAN_POINT('Ctrl Pts',(-16.1881480326967,-1.43676012847776,
-0.892664308505406));
#32192=CARTESIAN_POINT('Ctrl Pts',(-16.1007304018405,-0.38944755395593,
-1.79623832185249));
#32193=CARTESIAN_POINT('Ctrl Pts',(-15.9896908818278,1.29675670604634,-1.30252199654784));
#32194=CARTESIAN_POINT('Ctrl Pts',(-15.8786513618151,1.7979482560302,0.381475523206329));
#32195=CARTESIAN_POINT('Ctrl Pts',(-15.7676118418024,0.656124176779396,
1.71686999240324));
#32196=CARTESIAN_POINT('Ctrl Pts',(-15.6587093126628,-1.05177064300029,
1.48783477827668));
#32197=CARTESIAN_POINT('Ctrl Pts',(-15.5868199568608,-1.55564276964987,
0.484385647412444));
#32198=CARTESIAN_POINT('Ctrl Pts',(-15.5519437743963,-1.55781326646842,
-0.000536565987745981));
#32199=CARTESIAN_POINT('Origin',(-20.9400562256037,0.,0.));
#32200=CARTESIAN_POINT('',(-17.0900562256037,-1.55801584159885,0.000174956040060638));
#32201=CARTESIAN_POINT('',(-16.9519437743963,-1.55404711770872,0.00119070638040702));
#32202=CARTESIAN_POINT('',(-20.9400562256037,-1.5555,1.83293981223255E-13));
#32203=CARTESIAN_POINT('Ctrl Pts',(-17.0900562256037,-1.55801584159885,
0.000174956040060662));
#32204=CARTESIAN_POINT('Ctrl Pts',(-17.0537213236343,-1.55720986486587,
-0.504853817882453));
#32205=CARTESIAN_POINT('Ctrl Pts',(-16.9803732483272,-1.0155113961936,-1.52582327293244));
#32206=CARTESIAN_POINT('Ctrl Pts',(-16.8700119996827,0.723039919366596,
-1.68977956052457));
#32207=CARTESIAN_POINT('Ctrl Pts',(-16.7589724796699,1.81154203999908,-0.310575472322002));
#32208=CARTESIAN_POINT('Ctrl Pts',(-16.6479329596573,1.24460614954145,1.35244120715334));
#32209=CARTESIAN_POINT('Ctrl Pts',(-16.5368934396446,-0.459685807164506,
1.77955911551557));
#32210=CARTESIAN_POINT('Ctrl Pts',(-16.4509345282934,-1.45383630619501,
0.851306302953154));
#32211=CARTESIAN_POINT('Ctrl Pts',(-16.4019887902798,-1.55544914551719,
0.168152079380301));
#32212=CARTESIAN_POINT('Ctrl Pts',(-16.3900562256037,-1.55419531422885,
0.00124249107025116));
#32213=CARTESIAN_POINT('Ctrl Pts',(-16.9519437743963,-1.55404711770872,
0.00119070638040689));
#32214=CARTESIAN_POINT('Ctrl Pts',(-16.9272981969073,-1.55158138149309,
-0.34362803432111));
#32215=CARTESIAN_POINT('Ctrl Pts',(-16.8656394460808,-1.26828644052862,
-1.20998033778118));
#32216=CARTESIAN_POINT('Ctrl Pts',(-16.7669675219167,0.164364346776865,
-1.83060805961026));
#32217=CARTESIAN_POINT('Ctrl Pts',(-16.655928001904,1.62638365175698,-0.856164542273203));
#32218=CARTESIAN_POINT('Ctrl Pts',(-16.5448884818913,1.60216788290627,0.900666187385256));
#32219=CARTESIAN_POINT('Ctrl Pts',(-16.4338489618786,0.113846090200382,
1.83444285109954));
#32220=CARTESIAN_POINT('Ctrl Pts',(-16.3362007260469,-1.28647431282795,
1.18140975480378));
#32221=CARTESIAN_POINT('Ctrl Pts',(-16.2755656635528,-1.55168051808682,
0.329620634919902));
#32222=CARTESIAN_POINT('Ctrl Pts',(-16.2519437743963,-1.55372892642411,
-0.00104588007964796));
#32223=CARTESIAN_POINT('Origin',(-20.9400562256037,0.,0.));
#32224=CARTESIAN_POINT('',(-17.7900562256037,-1.55469842977811,-0.00136248394244802));
#32225=CARTESIAN_POINT('',(-17.6519437743963,-1.55797555090531,0.00028566433304557));
#32226=CARTESIAN_POINT('',(-20.9400562256037,-1.5555,1.83293981223255E-13));
#32227=CARTESIAN_POINT('Ctrl Pts',(-17.7900562256037,-1.55469842977811,
-0.00136248394244807));
#32228=CARTESIAN_POINT('Ctrl Pts',(-17.7794802036639,-1.55594593301098,
-0.149176061089705));
#32229=CARTESIAN_POINT('Ctrl Pts',(-17.7318910083865,-1.46881329755037,
-0.812855446110298));
#32230=CARTESIAN_POINT('Ctrl Pts',(-17.6472886397715,-0.524370017185474,
-1.76158383684904));
#32231=CARTESIAN_POINT('Ctrl Pts',(-17.5362491197588,1.19438366161834,-1.39699298808207));
#32232=CARTESIAN_POINT('Ctrl Pts',(-17.4252095997461,1.821676008134,0.244209379874806));
#32233=CARTESIAN_POINT('Ctrl Pts',(-17.3141700797334,0.784269631776072,
1.66224631422945));
#32234=CARTESIAN_POINT('Ctrl Pts',(-17.2031305597208,-0.96982436419101,
1.56127588796884));
#32235=CARTESIAN_POINT('Ctrl Pts',(-17.1284259416775,-1.55368629794985,
0.533471930190121));
#32236=CARTESIAN_POINT('Ctrl Pts',(-17.0907344969718,-1.5580308869385,0.00960243592468178));
#32237=CARTESIAN_POINT('Ctrl Pts',(-17.0900562256037,-1.55801584159885,
0.000174956040060662));
#32238=CARTESIAN_POINT('Ctrl Pts',(-17.6519437743963,-1.55797555090531,
0.000285664333045577));
#32239=CARTESIAN_POINT('Ctrl Pts',(-17.6160439035994,-1.55671161178009,
-0.498731121651786));
#32240=CARTESIAN_POINT('Ctrl Pts',(-17.5431308594649,-1.02647039901201,
-1.51454913854194));
#32241=CARTESIAN_POINT('Ctrl Pts',(-17.4332046419928,0.703195832570145,
-1.6981334271154));
#32242=CARTESIAN_POINT('Ctrl Pts',(-17.3221651219801,1.80777954461665,-0.331774961689621));
#32243=CARTESIAN_POINT('Ctrl Pts',(-17.2111256019674,1.26036351771076,1.33776877909999));
#32244=CARTESIAN_POINT('Ctrl Pts',(-17.1000860819547,-0.438808100203742,
1.78482182831828));
#32245=CARTESIAN_POINT('Ctrl Pts',(-17.013692139431,-1.44885012350902,0.86363987975288));
#32246=CARTESIAN_POINT('Ctrl Pts',(-16.9643113702449,-1.55528446866947,
0.174226977407924));
#32247=CARTESIAN_POINT('Ctrl Pts',(-16.9519437743963,-1.55404711770872,
0.00119070638040689));
#32248=CARTESIAN_POINT('Origin',(-20.9400562256037,0.,0.));
#32249=CARTESIAN_POINT('',(-18.4900562256037,-1.55329134941458,0.000728404769962799));
#32250=CARTESIAN_POINT('',(-18.3519437743963,-1.55487053919943,-0.00138677294343165));
#32251=CARTESIAN_POINT('',(-20.9400562256037,-1.5555,1.83293981223255E-13));
#32252=CARTESIAN_POINT('Ctrl Pts',(-18.4900562256037,-1.55329134941458,
0.000728404769962943));
#32253=CARTESIAN_POINT('Ctrl Pts',(-18.4682259103559,-1.5519987435958,-0.305075653610566));
#32254=CARTESIAN_POINT('Ctrl Pts',(-18.4093824217706,-1.31686688150724,
-1.13120485114901));
#32255=CARTESIAN_POINT('Ctrl Pts',(-18.3135257598477,0.0252485661867687,
-1.83779672371819));
#32256=CARTESIAN_POINT('Ctrl Pts',(-18.202486239835,1.5568693034731,-0.976883390785028));
#32257=CARTESIAN_POINT('Ctrl Pts',(-18.0914467198223,1.66577977622518,0.776737156863176));
#32258=CARTESIAN_POINT('Ctrl Pts',(-17.9804071998096,0.252453550943756,
1.820551509628));
#32259=CARTESIAN_POINT('Ctrl Pts',(-17.8799437017367,-1.2349855334043,1.25973428479012));
#32260=CARTESIAN_POINT('Ctrl Pts',(-17.8164933770014,-1.55158001417496,
0.368130879433178));
#32261=CARTESIAN_POINT('Ctrl Pts',(-17.7900562256037,-1.55469842977811,
-0.00136248394244807));
#32262=CARTESIAN_POINT('Ctrl Pts',(-18.3519437743963,-1.55487053919943,
-0.00138677294343177));
#32263=CARTESIAN_POINT('Ctrl Pts',(-18.341802783629,-1.55609861243653,-0.143080456376997));
#32264=CARTESIAN_POINT('Ctrl Pts',(-18.2946486195241,-1.47343564403532,
-0.800528910503304));
#32265=CARTESIAN_POINT('Ctrl Pts',(-18.2104812820817,-0.544969521563382,
-1.75532009416732));
#32266=CARTESIAN_POINT('Ctrl Pts',(-18.099441762069,1.17793694271932,-1.4108885006591));
#32267=CARTESIAN_POINT('Ctrl Pts',(-17.9884022420563,1.82441171535083,0.222853162755832));
#32268=CARTESIAN_POINT('Ctrl Pts',(-17.8773627220436,0.803687711301754,
1.6529450720079));
#32269=CARTESIAN_POINT('Ctrl Pts',(-17.7663232020309,-0.95146865288028,
1.57252947891983));
#32270=CARTESIAN_POINT('Ctrl Pts',(-17.6911835528151,-1.55080035464189,
0.545690517664059));
#32271=CARTESIAN_POINT('Ctrl Pts',(-17.6530570769369,-1.5580147473316,0.0157608357841803));
#32272=CARTESIAN_POINT('Ctrl Pts',(-17.6519437743963,-1.55797555090531,
0.000285664333045577));
#32273=CARTESIAN_POINT('Origin',(-20.9400562256037,0.,0.));
#32274=CARTESIAN_POINT('',(-19.1900562256037,-1.55732260026824,0.00102952447757971));
#32275=CARTESIAN_POINT('',(-19.0519437743963,-1.55320700821059,0.000650635102509151));
#32276=CARTESIAN_POINT('',(-20.9400562256037,-1.5555,1.83293981223255E-13));
#32277=CARTESIAN_POINT('Ctrl Pts',(-19.1900562256037,-1.55732260026824,
0.00102952447757978));
#32278=CARTESIAN_POINT('Ctrl Pts',(-19.156971617048,-1.5540834599925,-0.459324401254566));
#32279=CARTESIAN_POINT('Ctrl Pts',(-19.0868738351547,-1.09444465366423,
-1.44067331686593));
#32280=CARTESIAN_POINT('Ctrl Pts',(-18.9797628799239,0.572581864613586,
-1.74641810285352));
#32281=CARTESIAN_POINT('Ctrl Pts',(-18.8687233599111,1.7774511739937,-0.467787493561026));
#32282=CARTESIAN_POINT('Ctrl Pts',(-18.7576838398985,1.35806626263998,1.23849733645003));
#32283=CARTESIAN_POINT('Ctrl Pts',(-18.6466443198858,-0.302373835599965,
1.81291555390549));
#32284=CARTESIAN_POINT('Ctrl Pts',(-18.5574351151208,-1.41437165322348,
0.943454576583954));
#32285=CARTESIAN_POINT('Ctrl Pts',(-18.5052390836935,-1.55419034929111,
0.213413360024777));
#32286=CARTESIAN_POINT('Ctrl Pts',(-18.4900562256037,-1.55329134941458,
0.000728404769962943));
#32287=CARTESIAN_POINT('Ctrl Pts',(-19.0519437743963,-1.55320700821059,
0.000650635102509029));
#32288=CARTESIAN_POINT('Ctrl Pts',(-19.030548490321,-1.55209814412289,-0.29910286970105));
#32289=CARTESIAN_POINT('Ctrl Pts',(-18.9721400329082,-1.32398103540958,
-1.11899594634625));
#32290=CARTESIAN_POINT('Ctrl Pts',(-18.8767184021578,0.00372273104669908,
-1.83795501911246));
#32291=CARTESIAN_POINT('Ctrl Pts',(-18.7656788821451,1.54531676928027,-0.995059804671333));
#32292=CARTESIAN_POINT('Ctrl Pts',(-18.6546393621325,1.67476548588617,0.757173652727654));
#32293=CARTESIAN_POINT('Ctrl Pts',(-18.5435998421197,0.273761951577427,
1.81746760404448));
#32294=CARTESIAN_POINT('Ctrl Pts',(-18.4427013128744,-1.22661269048955,
1.27176249184623));
#32295=CARTESIAN_POINT('Ctrl Pts',(-18.3788159569665,-1.55161631986385,
0.374081326539656));
#32296=CARTESIAN_POINT('Ctrl Pts',(-18.3519437743963,-1.55487053919943,
-0.00138677294343177));
#32297=CARTESIAN_POINT('Ctrl Pts',(-19.8760740822721,-0.685825729128707,
1.39614588036676));
#32298=CARTESIAN_POINT('Ctrl Pts',(-19.8390609089345,-1.14966653079063,
1.1682943639365));
#32299=CARTESIAN_POINT('Ctrl Pts',(-19.7650345622594,-1.82446514616035,
0.217992868365382));
#32300=CARTESIAN_POINT('Ctrl Pts',(-19.6539950422467,-1.1726414776927,-1.41687333944346));
#32301=CARTESIAN_POINT('Ctrl Pts',(-19.542955522234,0.552287169619636,-1.75246537632802));
#32302=CARTESIAN_POINT('Ctrl Pts',(-19.4319160022213,1.77174315090552,-0.488859491694061));
#32303=CARTESIAN_POINT('Ctrl Pts',(-19.3208764822086,1.37253690144282,1.22265204623408));
#32304=CARTESIAN_POINT('Ctrl Pts',(-19.2098369621959,-0.281145520007231,
1.81625519837393));
#32305=CARTESIAN_POINT('Ctrl Pts',(-19.0987974421832,-1.67779713459217,
0.750436187074751));
#32306=CARTESIAN_POINT('Ctrl Pts',(-18.9877579221705,-1.541289524424,-1.00132217474655));
#32307=CARTESIAN_POINT('Ctrl Pts',(-18.8767184021578,0.00372273104669908,
-1.83795501911246));
#32308=CARTESIAN_POINT('Ctrl Pts',(-18.7656788821451,1.54531676928027,-0.995059804671333));
#32309=CARTESIAN_POINT('Ctrl Pts',(-18.6546393621325,1.67476548588617,0.757173652727654));
#32310=CARTESIAN_POINT('Ctrl Pts',(-18.5435998421197,0.273761951577427,
1.81746760404448));
#32311=CARTESIAN_POINT('Ctrl Pts',(-18.4325603221071,-1.3774105812666,1.21691540392665));
#32312=CARTESIAN_POINT('Ctrl Pts',(-18.3215208020943,-1.76986786954587,
-0.495691858702389));
#32313=CARTESIAN_POINT('Ctrl Pts',(-18.2104812820817,-0.544969521563382,
-1.75532009416732));
#32314=CARTESIAN_POINT('Ctrl Pts',(-18.099441762069,1.17793694271932,-1.4108885006591));
#32315=CARTESIAN_POINT('Ctrl Pts',(-17.9884022420563,1.82441171535083,0.222853162755832));
#32316=CARTESIAN_POINT('Ctrl Pts',(-17.8773627220436,0.803687711301754,
1.6529450720079));
#32317=CARTESIAN_POINT('Ctrl Pts',(-17.7663232020309,-0.95146865288028,
1.57252947891983));
#32318=CARTESIAN_POINT('Ctrl Pts',(-17.6552836820182,-1.83714625700249,
0.0550921927705897));
#32319=CARTESIAN_POINT('Ctrl Pts',(-17.5442441620055,-1.0439879835733,-1.5126898472865));
#32320=CARTESIAN_POINT('Ctrl Pts',(-17.4332046419928,0.703195832570145,
-1.6981334271154));
#32321=CARTESIAN_POINT('Ctrl Pts',(-17.3221651219801,1.80777954461665,-0.331774961689621));
#32322=CARTESIAN_POINT('Ctrl Pts',(-17.2111256019674,1.26036351771076,1.33776877909999));
#32323=CARTESIAN_POINT('Ctrl Pts',(-17.1000860819547,-0.438808100203742,
1.78482182831828));
#32324=CARTESIAN_POINT('Ctrl Pts',(-16.9890465619421,-1.7369845485084,0.600854545137668));
#32325=CARTESIAN_POINT('Ctrl Pts',(-16.8780070419293,-1.44785571598004,
-1.13219050140136));
#32326=CARTESIAN_POINT('Ctrl Pts',(-16.7669675219167,0.164364346776865,
-1.83060805961026));
#32327=CARTESIAN_POINT('Ctrl Pts',(-16.655928001904,1.62638365175698,-0.856164542273203));
#32328=CARTESIAN_POINT('Ctrl Pts',(-16.5448884818913,1.60216788290627,0.900666187385256));
#32329=CARTESIAN_POINT('Ctrl Pts',(-16.4338489618786,0.113846090200382,
1.83444285109954));
#32330=CARTESIAN_POINT('Ctrl Pts',(-16.3228094418659,-1.47851145821767,
1.09185409926492));
#32331=CARTESIAN_POINT('Ctrl Pts',(-16.2117699218532,-1.71976369772685,
-0.648501603808868));
#32332=CARTESIAN_POINT('Ctrl Pts',(-16.1007304018405,-0.38944755395593,
-1.79623832185249));
#32333=CARTESIAN_POINT('Ctrl Pts',(-15.9896908818278,1.29675670604634,-1.30252199654784));
#32334=CARTESIAN_POINT('Ctrl Pts',(-15.8786513618151,1.7979482560302,0.381475523206329));
#32335=CARTESIAN_POINT('Ctrl Pts',(-15.7676118418024,0.656124176779396,
1.71686999240324));
#32336=CARTESIAN_POINT('Ctrl Pts',(-15.6565723217897,-1.0852846088457,1.48334042753872));
#32337=CARTESIAN_POINT('Ctrl Pts',(-15.545532801777,-1.83492982812703,-0.105707294062363));
#32338=CARTESIAN_POINT('Ctrl Pts',(-15.4344932817643,-0.907764618603845,
-1.59815672053134));
#32339=CARTESIAN_POINT('Ctrl Pts',(-15.3234537617517,0.848941402803422,
-1.63016563599362));
#32340=CARTESIAN_POINT('Ctrl Pts',(-15.212414241739,1.82986091954754,-0.172483394218017));
#32341=CARTESIAN_POINT('Ctrl Pts',(-15.1013747217263,1.13860211855666,1.4428190190688));
#32342=CARTESIAN_POINT('Ctrl Pts',(-14.9903352017136,-0.593143287092892,
1.7396328771166));
#32343=CARTESIAN_POINT('Ctrl Pts',(-14.8792956817009,-1.78285769279516,
0.446721337535475));
#32344=CARTESIAN_POINT('Ctrl Pts',(-14.7682561616882,-1.3433466499118,-1.25441671080192));
#32345=CARTESIAN_POINT('Ctrl Pts',(-14.6572166416755,0.323752302625325,
-1.80923352630697));
#32346=CARTESIAN_POINT('Ctrl Pts',(-14.5461771216628,1.6949973052892,-0.71072191554133));
#32347=CARTESIAN_POINT('Ctrl Pts',(-14.4351376016501,1.51730614988444,1.03726734918786));
#32348=CARTESIAN_POINT('Ctrl Pts',(-14.3240980816374,-0.0469419935946381,
1.8373725684808));
#32349=CARTESIAN_POINT('Ctrl Pts',(-14.2130585616247,-1.56829322450421,
0.958435114205744));
#32350=CARTESIAN_POINT('Ctrl Pts',(-14.102019041612,-1.65649404608369,-0.796347274408376));
#32351=CARTESIAN_POINT('Ctrl Pts',(-13.9909795215993,-0.230944069595307,
-1.82340515050471));
#32352=CARTESIAN_POINT('Ctrl Pts',(-13.8799400015866,1.40564908600105,-1.18418417199048));
#32353=CARTESIAN_POINT('Ctrl Pts',(-13.7689004815739,1.75772061547503,0.537177572225828));
#32354=CARTESIAN_POINT('Ctrl Pts',(-13.6578609615613,0.503537663837979,
1.76765135908215));
#32355=CARTESIAN_POINT('Ctrl Pts',(-13.5468214415485,-1.21079215177004,
1.38279567231766));
#32356=CARTESIAN_POINT('Ctrl Pts',(-13.4357819215359,-1.81866608220935,
-0.265697549084784));
#32357=CARTESIAN_POINT('Ctrl Pts',(-13.3247424015232,-0.764591851789241,
-1.67138888543208));
#32358=CARTESIAN_POINT('Ctrl Pts',(-13.2137028815105,0.988187893799185,
-1.54971810104841));
#32359=CARTESIAN_POINT('Ctrl Pts',(-13.1026633614978,1.83793377915969,-0.0118713770116975));
#32360=CARTESIAN_POINT('Ctrl Pts',(-12.9916238414851,1.00812414086676,1.53682374486147));
#32361=CARTESIAN_POINT('Ctrl Pts',(-12.8805843214724,-0.742937660327962,
1.68112615202868));
#32362=CARTESIAN_POINT('Ctrl Pts',(-12.7695448014597,-1.81508215488039,
0.289168250683079));
#32363=CARTESIAN_POINT('Ctrl Pts',(-12.658505281447,-1.22855358205609,-1.36703972224128));
#32364=CARTESIAN_POINT('Ctrl Pts',(-12.5474657614343,0.480661769934936,
-1.77400839036668));
#32365=CARTESIAN_POINT('Ctrl Pts',(-12.4364262414216,1.75063489249572,-0.559838351084378));
#32366=CARTESIAN_POINT('Ctrl Pts',(-12.3253867214089,1.42082866667544,1.16592770192737));
#32367=CARTESIAN_POINT('Ctrl Pts',(-12.2143472013962,-0.207370712553722,
1.82623626449135));
#32368=CARTESIAN_POINT('Ctrl Pts',(-12.1033076813836,-1.64606890862666,
0.817678820944377));
#32369=CARTESIAN_POINT('Ctrl Pts',(-11.9922681613708,-1.58054309013141,
-0.938096501649056));
#32370=CARTESIAN_POINT('Ctrl Pts',(-11.8812286413582,-0.0706725909392507,
-1.83661288546561));
#32371=CARTESIAN_POINT('Ctrl Pts',(-11.7701891213455,1.50378050738072,-1.05678081539653));
#32372=CARTESIAN_POINT('Ctrl Pts',(-11.6591496013328,1.70403672974556,0.688767253755881));
#32373=CARTESIAN_POINT('Ctrl Pts',(-11.5481100813201,0.34709631401335,1.80490045569464));
#32374=CARTESIAN_POINT('Ctrl Pts',(-11.4370705613074,-1.32703046504225,
1.2716649130247));
#32375=CARTESIAN_POINT('Ctrl Pts',(-11.3260310412947,-1.78847952257671,
-0.423653754252368));
#32376=CARTESIAN_POINT('Ctrl Pts',(-11.214991521282,-0.615565745527372,
-1.73182571845486));
#32377=CARTESIAN_POINT('Ctrl Pts',(-11.1039520012693,1.11986930393965,-1.45740668595354));
#32378=CARTESIAN_POINT('Ctrl Pts',(-10.9929124812566,1.83193632103844,0.148831521622652));
#32379=CARTESIAN_POINT('Ctrl Pts',(-10.8818729612439,0.869928460211977,
1.61906330335833));
#32380=CARTESIAN_POINT('Ctrl Pts',(-10.7708334412312,-0.887044467963301,
1.60974955133526));
#32381=CARTESIAN_POINT('Ctrl Pts',(-10.6597939212185,-1.83341124003695,
0.129401433819494));
#32382=CARTESIAN_POINT('Ctrl Pts',(-10.5487544012059,-1.10435531176706,
-1.46919734941914));
#32383=CARTESIAN_POINT('Ctrl Pts',(-10.4377148811931,0.633891526962291,
-1.72520231805252));
#32384=CARTESIAN_POINT('Ctrl Pts',(-10.3266753611805,1.79287047934082,-0.404668939352399));
#32385=CARTESIAN_POINT('Ctrl Pts',(-10.2156358411678,1.31347401748173,1.28566228519341));
#32386=CARTESIAN_POINT('Ctrl Pts',(-10.1045963211551,-0.366211903252911,
1.8011191931919));
#32387=CARTESIAN_POINT('Ctrl Pts',(-9.99355680114238,-1.71124309816971,
0.670662780490254));
#32388=CARTESIAN_POINT('Ctrl Pts',(-9.88251728112968,-1.49249227306246,
-1.07266412311459));
#32389=CARTESIAN_POINT('Ctrl Pts',(-9.77147776111699,0.0901399223399556,
-1.83576041480606));
#32390=CARTESIAN_POINT('Ctrl Pts',(-9.66043824110429,1.59039972425115,-0.921287264250532));
#32391=CARTESIAN_POINT('Ctrl Pts',(-9.54939872109161,1.63730757628732,0.835084071696088));
#32392=CARTESIAN_POINT('Ctrl Pts',(-9.4383592010789,0.187997765394267,1.82833212146347));
#32393=CARTESIAN_POINT('Ctrl Pts',(-9.32731968106623,-1.43310968526294,
1.15079891213624));
#32394=CARTESIAN_POINT('Ctrl Pts',(-9.21628016105352,-1.74460124269406,
-0.578366674488338));
#32395=CARTESIAN_POINT('Ctrl Pts',(-9.10524064104083,-0.461827170446667,
-1.77900454490864));
#32396=CARTESIAN_POINT('Ctrl Pts',(-8.99420112102814,1.24297754506556,-1.35393808153518));
#32397=CARTESIAN_POINT('Ctrl Pts',(-8.88316160101544,1.81191445877564,0.308395039272923));
#32398=CARTESIAN_POINT('Ctrl Pts',(-8.77212208100275,0.725073034805075,
1.68890810891739));
#32399=CARTESIAN_POINT('Ctrl Pts',(-8.66108256099006,-1.0243604991031,1.52604949921214));
#32400=CARTESIAN_POINT('Ctrl Pts',(-8.55004304097736,-1.83770462979697,
-0.0313560168251536));
#32401=CARTESIAN_POINT('Ctrl Pts',(-8.43900352096468,-0.971702639962959,
-1.56010752374873));
#32402=CARTESIAN_POINT('Ctrl Pts',(-8.32796400095197,0.782268521994644,
-1.66318894466765));
#32403=CARTESIAN_POINT('Ctrl Pts',(-8.2169244809393,1.82138073092891,-0.246401581101293));
#32404=CARTESIAN_POINT('Ctrl Pts',(-8.10588496092658,1.1960640567365,1.39555446986186));
#32405=CARTESIAN_POINT('Ctrl Pts',(-7.99484544091391,-0.522249555601089,
1.76221363853615));
#32406=CARTESIAN_POINT('Ctrl Pts',(-7.8838059209012,-1.76331685156899,0.518512475395882));
#32407=CARTESIAN_POINT('Ctrl Pts',(-7.77276640088852,-1.39301566865845,
-1.19901995523027));
#32408=CARTESIAN_POINT('Ctrl Pts',(-7.66172688087582,0.250262368674325,
-1.82085426462248));
#32409=CARTESIAN_POINT('Ctrl Pts',(-7.55068736086313,1.66484362245829,-0.778740790589749));
#32410=CARTESIAN_POINT('Ctrl Pts',(-7.43964784085044,1.55804400070415,0.97500789639785));
#32411=CARTESIAN_POINT('Ctrl Pts',(-7.32860832083774,0.0274599982776329,
1.83776697507137));
#32412=CARTESIAN_POINT('Ctrl Pts',(-7.21756880082506,-1.52821772205629,
1.02112296035368));
#32413=CARTESIAN_POINT('Ctrl Pts',(-7.10652928081235,-1.68736715310754,
-0.728651903711305));
#32414=CARTESIAN_POINT('Ctrl Pts',(-6.99548976079967,-0.304553073520857,
-1.8125641868848));
#32415=CARTESIAN_POINT('Ctrl Pts',(-6.88445024078697,1.35657016098623,-1.24010439257756));
#32416=CARTESIAN_POINT('Ctrl Pts',(-6.77341072077428,1.77802146990873,0.465597636067849));
#32417=CARTESIAN_POINT('Ctrl Pts',(-6.66237120076158,0.574666806591611,
1.74582346403357));
#32418=CARTESIAN_POINT('Ctrl Pts',(-6.55133168074889,-1.15383452969896,
1.43066676212274));
#32419=CARTESIAN_POINT('Ctrl Pts',(-6.4402921607362,-1.82792945607851,-0.191873421215389));
#32420=CARTESIAN_POINT('Ctrl Pts',(-6.3292526407235,-0.831611090304988,
-1.6390742816145));
#32421=CARTESIAN_POINT('Ctrl Pts',(-6.21821312071081,0.924656853680087,
-1.58844301412132));
#32422=CARTESIAN_POINT('Ctrl Pts',(-6.10717360069812,1.83594738678564,-0.0862478934429835));
#32423=CARTESIAN_POINT('Ctrl Pts',(-5.99613408068542,1.06949761739632,1.49476297537502));
#32424=CARTESIAN_POINT('Ctrl Pts',(-5.88509456067274,-0.674289122018889,
1.70981744232983));
#32425=CARTESIAN_POINT('Ctrl Pts',(-5.77405504066003,-1.80189151776093,
0.362392693620539));
#32426=CARTESIAN_POINT('Ctrl Pts',(-5.66301552064736,-1.28287482091343,
-1.31619667984489));
#32427=CARTESIAN_POINT('Ctrl Pts',(-5.55197600063464,0.408468929309301,
-1.79200854907483));
#32428=CARTESIAN_POINT('Ctrl Pts',(-5.44093648062197,1.726542296104,-0.630232660159929));
#32429=CARTESIAN_POINT('Ctrl Pts',(-5.32989696060926,1.46685280597546,1.1074675398269));
#32430=CARTESIAN_POINT('Ctrl Pts',(-5.21885744059658,-0.133287989090187,
1.83313278791599));
#32431=CARTESIAN_POINT('Ctrl Pts',(-5.10781792058388,-1.61162647503488,
0.8836297930327));
#32432=CARTESIAN_POINT('Ctrl Pts',(-4.99677840057119,-1.61721540987848,
-0.873358932066274));
#32433=CARTESIAN_POINT('Ctrl Pts',(-4.8857388805585,-0.144947467941284,
-1.83224772825777));
#32434=CARTESIAN_POINT('Ctrl Pts',(-4.7746993605458,1.45977754246094,-1.11677707385809));
#32435=CARTESIAN_POINT('Ctrl Pts',(-4.66365984053311,1.73051682250325,0.619235846185912));
#32436=CARTESIAN_POINT('Ctrl Pts',(-4.55262032052042,0.419861211735448,
1.78937365271996));
#32437=CARTESIAN_POINT('Ctrl Pts',(-4.44158080050772,-1.27447537020456,
1.324331543425));
#32438=CARTESIAN_POINT('Ctrl Pts',(-4.33054128049503,-1.80416055280736,
-0.350921936991871));
#32439=CARTESIAN_POINT('Ctrl Pts',(-4.21950176048233,-0.685153134847353,
-1.70549309232754));
#32440=CARTESIAN_POINT('Ctrl Pts',(-4.10846224046965,1.0599664669302,-1.50153674452297));
#32441=CARTESIAN_POINT('Ctrl Pts',(-3.99742272045695,1.83645893175252,0.0745660657000111));
#32442=CARTESIAN_POINT('Ctrl Pts',(-3.88638320044426,0.93474362991831,1.5825283101715));
#32443=CARTESIAN_POINT('Ctrl Pts',(-3.77534368043157,-0.821166662308707,
1.64433172410147));
#32444=CARTESIAN_POINT('Ctrl Pts',(-3.66430416041887,-1.82667178805772,
0.20349861148378));
#32445=CARTESIAN_POINT('Ctrl Pts',(-3.55326464040618,-1.1629129140303,-1.42329724953858));
#32446=CARTESIAN_POINT('Ctrl Pts',(-3.44222512039348,0.563548452575144,
-1.74944409679311));
#32447=CARTESIAN_POINT('Ctrl Pts',(-3.3311856003808,1.77502341045502,-0.476899778205122));
#32448=CARTESIAN_POINT('Ctrl Pts',(-3.22014608036809,1.36443210709099,1.23144895602193));
#32449=CARTESIAN_POINT('Ctrl Pts',(-3.10910656035541,-0.293015589158281,
1.81446503711471));
#32450=CARTESIAN_POINT('Ctrl Pts',(-2.99806704034271,-1.68269740770543,
0.739371990178813));
#32451=CARTESIAN_POINT('Ctrl Pts',(-2.88702752033002,-1.53468306041474,
-1.01137995345248));
#32452=CARTESIAN_POINT('Ctrl Pts',(-2.77598800031732,0.0157677844803547,
-1.83790448190824));
#32453=CARTESIAN_POINT('Ctrl Pts',(-2.66494848030463,1.55180958399743,-0.984900257957451));
#32454=CARTESIAN_POINT('Ctrl Pts',(-2.55390896029194,1.66976418974896,0.768133489551486));
#32455=CARTESIAN_POINT('Ctrl Pts',(-2.44286944027925,0.261841363970268,
1.81922527888795));
#32456=CARTESIAN_POINT('Ctrl Pts',(-2.33182992026655,-1.38535945017504,
1.20785788805628));
#32457=CARTESIAN_POINT('Ctrl Pts',(-2.22079040025386,-1.76657988960961,
-0.507283956920983));
#32458=CARTESIAN_POINT('Ctrl Pts',(-2.10975088024117,-0.533449971191177,
-1.75885550507193));
#32459=CARTESIAN_POINT('Ctrl Pts',(-1.99871136022847,1.18716147401266,-1.40313541149553));
#32460=CARTESIAN_POINT('Ctrl Pts',(-1.88767184021578,1.82291149503699,0.234809115073605));
#32461=CARTESIAN_POINT('Ctrl Pts',(-1.77663232020309,0.792833618333258,
1.65817871653077));
#32462=CARTESIAN_POINT('Ctrl Pts',(-1.66559280019039,-0.96175759007224,
1.56625756194791));
#32463=CARTESIAN_POINT('Ctrl Pts',(-1.5545532801777,-1.83746826916603,0.0430471165426282));
#32464=CARTESIAN_POINT('Ctrl Pts',(-1.44351376016501,-1.03404772328313,
-1.51950265405236));
#32465=CARTESIAN_POINT('Ctrl Pts',(-1.33247424015232,0.714312595491066,
-1.69348504977325));
#32466=CARTESIAN_POINT('Ctrl Pts',(-1.22143472013962,1.8099179685225,-0.319919240308951));
#32467=CARTESIAN_POINT('Ctrl Pts',(-1.11039520012693,1.25156189493757,1.34600919589416));
#32468=CARTESIAN_POINT('Ctrl Pts',(-0.999355680114236,-0.45049222129505,
1.78189485367676));
#32469=CARTESIAN_POINT('Ctrl Pts',(-0.888316160101544,-1.74090124670998,
0.589476331112601));
#32470=CARTESIAN_POINT('Ctrl Pts',(-0.77727664008885,-1.44037375318949,
-1.14170098836771));
#32471=CARTESIAN_POINT('Ctrl Pts',(-0.66623712007616,0.17630871353902,-1.82941001051451));
#32472=CARTESIAN_POINT('Ctrl Pts',(-0.555197600063458,1.63206374948406,
-0.84563791873513));
#32473=CARTESIAN_POINT('Ctrl Pts',(-0.444158080050773,1.59603445699364,
0.91144468152982));
#32474=CARTESIAN_POINT('Ctrl Pts',(-0.333118560038075,0.102187466450462,
1.83458816486299));
#32475=CARTESIAN_POINT('Ctrl Pts',(-0.222079040025385,-1.48635127732985,
1.08322572698902));
#32476=CARTESIAN_POINT('Ctrl Pts',(-0.111039520012692,-1.71404440126355,
-0.662001322286585));
#32477=CARTESIAN_POINT('Ctrl Pts',(-0.0370131733375646,-0.825376844998173,
-1.41612072810435));
#32478=CARTESIAN_POINT('Ctrl Pts',(0.,-0.319621170202026,-1.52230829911641));
#32479=CARTESIAN_POINT('Ctrl Pts',(-19.7993827215147,-0.744392439309325,
1.51537102412035));
#32480=CARTESIAN_POINT('Ctrl Pts',(-19.7623695481771,-1.24784334693123,
1.26806192078395));
#32481=CARTESIAN_POINT('Ctrl Pts',(-19.688343201502,-1.98026700210055,0.236608567078233));
#32482=CARTESIAN_POINT('Ctrl Pts',(-19.5773036814893,-1.27278026026218,
-1.53786852336466));
#32483=CARTESIAN_POINT('Ctrl Pts',(-19.4662641614766,0.599450233391951,
-1.90211874661982));
#32484=CARTESIAN_POINT('Ctrl Pts',(-19.3552246414639,1.92304276424226,-0.530606091381193));
#32485=CARTESIAN_POINT('Ctrl Pts',(-19.2441851214512,1.48974593502792,1.32706152666359));
#32486=CARTESIAN_POINT('Ctrl Pts',(-19.1331456014385,-0.305154196686319,
1.9713559583765));
#32487=CARTESIAN_POINT('Ctrl Pts',(-19.0221060814259,-1.8210741426571,0.814520365913112));
#32488=CARTESIAN_POINT('Ctrl Pts',(-18.9110665614131,-1.67290934130666,
-1.08683099005494));
#32489=CARTESIAN_POINT('Ctrl Pts',(-18.8000270414005,0.00404063704095619,
-1.99490885498866));
#32490=CARTESIAN_POINT('Ctrl Pts',(-18.6889875213878,1.67728049639015,-1.08003383920717));
#32491=CARTESIAN_POINT('Ctrl Pts',(-18.5779480013751,1.81778360356014,0.821833183556338));
#32492=CARTESIAN_POINT('Ctrl Pts',(-18.4669084813624,0.297140101733544,
1.97267189852895));
#32493=CARTESIAN_POINT('Ctrl Pts',(-18.3558689613497,-1.4950358071607,1.32083499858318));
#32494=CARTESIAN_POINT('Ctrl Pts',(-18.244829441337,-1.92100734153001,-0.538021914567167));
#32495=CARTESIAN_POINT('Ctrl Pts',(-18.1337899213243,-0.591507688142816,
-1.90521724567824));
#32496=CARTESIAN_POINT('Ctrl Pts',(-18.0227504013116,1.27852793632774,-1.53137260384405));
#32497=CARTESIAN_POINT('Ctrl Pts',(-17.9117108812989,1.98020900851858,0.241883910716462));
#32498=CARTESIAN_POINT('Ctrl Pts',(-17.8006713612862,0.872319352350435,
1.79409981564771));
#32499=CARTESIAN_POINT('Ctrl Pts',(-17.6896318412736,-1.03272018147192,
1.7068170600512));
#32500=CARTESIAN_POINT('Ctrl Pts',(-17.5785923212608,-1.99403102790477,
0.0597968405406536));
#32501=CARTESIAN_POINT('Ctrl Pts',(-17.4675528012482,-1.13314028432416,
-1.64186736880022));
#32502=CARTESIAN_POINT('Ctrl Pts',(-17.3565132812354,0.763245878488775,
-1.84314707132529));
#32503=CARTESIAN_POINT('Ctrl Pts',(-17.2454737612228,1.96215651847923,-0.360107185461877));
#32504=CARTESIAN_POINT('Ctrl Pts',(-17.1344342412101,1.36799340345118,1.45200875734308));
#32505=CARTESIAN_POINT('Ctrl Pts',(-17.0233947211974,-0.47628051591815,
1.93723830717499));
#32506=CARTESIAN_POINT('Ctrl Pts',(-16.9123552011847,-1.8853159194675,0.65216506399276));
#32507=CARTESIAN_POINT('Ctrl Pts',(-16.801315681172,-1.57149666804647,-1.22887493616156));
#32508=CARTESIAN_POINT('Ctrl Pts',(-16.6902761611593,0.178400389247811,
-1.98693449521611));
#32509=CARTESIAN_POINT('Ctrl Pts',(-16.5792366411466,1.76527015882334,-0.929277489899003));
#32510=CARTESIAN_POINT('Ctrl Pts',(-16.4681971211339,1.73898646242799,0.977579393358277));
#32511=CARTESIAN_POINT('Ctrl Pts',(-16.3571576011212,0.123568080331052,
1.99109676220276));
#32512=CARTESIAN_POINT('Ctrl Pts',(-16.2461180811085,-1.60477028519716,
1.18509397037967));
#32513=CARTESIAN_POINT('Ctrl Pts',(-16.1350785610958,-1.86662447851419,
-0.703880986454943));
#32514=CARTESIAN_POINT('Ctrl Pts',(-16.0240390410831,-0.422704781053617,
-1.94962972252928));
#32515=CARTESIAN_POINT('Ctrl Pts',(-15.9129995210704,1.4074944211132,-1.41375204382615));
#32516=CARTESIAN_POINT('Ctrl Pts',(-15.8019600010578,1.95148567808699,0.414051971507585));
#32517=CARTESIAN_POINT('Ctrl Pts',(-15.690920481045,0.712154495957904,1.86348366259991));
#32518=CARTESIAN_POINT('Ctrl Pts',(-15.5798809610324,-1.17796347236763,
1.61001162873322));
#32519=CARTESIAN_POINT('Ctrl Pts',(-15.4688414410197,-1.99162532507519,
-0.114734264315));
#32520=CARTESIAN_POINT('Ctrl Pts',(-15.357801921007,-0.985284001548998,
-1.73463276320396));
#32521=CARTESIAN_POINT('Ctrl Pts',(-15.2467624009943,0.921437523882869,
-1.7693751090341));
#32522=CARTESIAN_POINT('Ctrl Pts',(-15.1357228809816,1.98612355245008,-0.187212770109111));
#32523=CARTESIAN_POINT('Ctrl Pts',(-15.0246833609689,1.23583407917913,1.56602985783425));
#32524=CARTESIAN_POINT('Ctrl Pts',(-14.9136438409562,-0.643795296073198,
1.88819040449921));
#32525=CARTESIAN_POINT('Ctrl Pts',(-14.8026043209435,-1.93510644251742,
0.484869511329067));
#32526=CARTESIAN_POINT('Ctrl Pts',(-14.6915648009308,-1.45806295549196,
-1.36153876357265));
#32527=CARTESIAN_POINT('Ctrl Pts',(-14.5805252809181,0.351399424150296,
-1.96373466425475));
#32528=CARTESIAN_POINT('Ctrl Pts',(-14.4694857609054,1.8397431375313,-0.77141465814138));
#32529=CARTESIAN_POINT('Ctrl Pts',(-14.3584462408927,1.64687788474545,1.12584573526981));
#32530=CARTESIAN_POINT('Ctrl Pts',(-14.2474067208801,-0.0509506477139025,
1.99427666545703));
#32531=CARTESIAN_POINT('Ctrl Pts',(-14.1363672008673,-1.7022190468475,1.04028155008079));
#32532=CARTESIAN_POINT('Ctrl Pts',(-14.0253276808547,-1.79795185758359,
-0.864352072190827));
#32533=CARTESIAN_POINT('Ctrl Pts',(-13.914288160842,-0.250665747883883,
-1.97911648715448));
#32534=CARTESIAN_POINT('Ctrl Pts',(-13.8032486408293,1.52568576461917,-1.2853086534087));
#32535=CARTESIAN_POINT('Ctrl Pts',(-13.6922091208166,1.90782276168028,0.583050338224345));
#32536=CARTESIAN_POINT('Ctrl Pts',(-13.5811696008039,0.546537719348393,
1.91860155014488));
#32537=CARTESIAN_POINT('Ctrl Pts',(-13.4701300807912,-1.31418884575491,
1.50088076294629));
#32538=CARTESIAN_POINT('Ctrl Pts',(-13.3590905607785,-1.97397272182371,
-0.288387032275693));
#32539=CARTESIAN_POINT('Ctrl Pts',(-13.2480510407658,-0.829884866455036,
-1.81411865524772));
#32540=CARTESIAN_POINT('Ctrl Pts',(-13.1370115207531,1.07257509527332,-1.6820576838766));
#32541=CARTESIAN_POINT('Ctrl Pts',(-13.0259720007404,1.99488580123086,-0.0128851440188925));
#32542=CARTESIAN_POINT('Ctrl Pts',(-12.9149324807277,1.09421381624131,1.66806220244796));
#32543=CARTESIAN_POINT('Ctrl Pts',(-12.803892960715,-0.806381495673676,
1.824687444557));
#32544=CARTESIAN_POINT('Ctrl Pts',(-12.6928534407024,-1.97008274176989,
0.313862035724786));
#32545=CARTESIAN_POINT('Ctrl Pts',(-12.5818139206897,-1.33346702948977,
-1.48377931922258));
#32546=CARTESIAN_POINT('Ctrl Pts',(-12.470774400677,0.521708317737177,-1.92550144588175));
#32547=CARTESIAN_POINT('Ctrl Pts',(-12.3597348806643,1.90013194696043,-0.607646254846737));
#32548=CARTESIAN_POINT('Ctrl Pts',(-12.2486953606516,1.54216161935306,1.26549315552602));
#32549=CARTESIAN_POINT('Ctrl Pts',(-12.1376558406389,-0.225079322636813,
1.98218936668781));
#32550=CARTESIAN_POINT('Ctrl Pts',(-12.0266163206262,-1.78663645605788,
0.88750524549088));
#32551=CARTESIAN_POINT('Ctrl Pts',(-11.9155768006135,-1.71551500086051,
-1.0182061032578));
#32552=CARTESIAN_POINT('Ctrl Pts',(-11.8045372806008,-0.0767077409422943,
-1.99345210862173));
#32553=CARTESIAN_POINT('Ctrl Pts',(-11.6934977605881,1.63219720773243,-1.14702557162399));
#32554=CARTESIAN_POINT('Ctrl Pts',(-11.5824582405754,1.84955449183783,0.747585158099991));
#32555=CARTESIAN_POINT('Ctrl Pts',(-11.4714187205627,0.376736918563704,
1.95903156714741));
#32556=CARTESIAN_POINT('Ctrl Pts',(-11.36037920055,-1.44035343521676,1.38025989166828));
#32557=CARTESIAN_POINT('Ctrl Pts',(-11.2493396805373,-1.94120835355214,
-0.459832050849315));
#32558=CARTESIAN_POINT('Ctrl Pts',(-11.1383001605246,-0.668132540682749,
-1.8797165464425));
#32559=CARTESIAN_POINT('Ctrl Pts',(-11.027260640512,1.21550155886733,-1.58186325176356));
#32560=CARTESIAN_POINT('Ctrl Pts',(-10.9162211204993,1.98837618473367,0.161541124401333));
#32561=CARTESIAN_POINT('Ctrl Pts',(-10.8051816004866,0.944216790093985,
1.75732468263366));
#32562=CARTESIAN_POINT('Ctrl Pts',(-10.6941420804739,-0.962794434851429,
1.74721557430902));
#32563=CARTESIAN_POINT('Ctrl Pts',(-10.5831025604612,-1.98997705577781,
0.140451786627161));
#32564=CARTESIAN_POINT('Ctrl Pts',(-10.4720630404485,-1.19866273526199,
-1.59466078962992));
#32565=CARTESIAN_POINT('Ctrl Pts',(-10.3610235204358,0.688023268844763,
-1.87252753475538));
#32566=CARTESIAN_POINT('Ctrl Pts',(-10.2499840004231,1.9459742800517,-0.439226010461765));
#32567=CARTESIAN_POINT('Ctrl Pts',(-10.1389444804104,1.42563932252114,1.39545258212894));
#32568=CARTESIAN_POINT('Ctrl Pts',(-10.0279049603977,-0.39748490088419,
1.95492740030364));
#32569=CARTESIAN_POINT('Ctrl Pts',(-9.91686544038502,-1.85737625462972,
0.727934636919118));
#32570=CARTESIAN_POINT('Ctrl Pts',(-9.80582592037233,-1.61994500440615,
-1.16426524881077));
#32571=CARTESIAN_POINT('Ctrl Pts',(-9.69478640035963,0.0978375027648033,
-1.99252684045702));
#32572=CARTESIAN_POINT('Ctrl Pts',(-9.58374688034695,1.72621335119086,-0.999961425785681));
#32573=CARTESIAN_POINT('Ctrl Pts',(-9.47270736033424,1.77712694179689,0.906396833417073));
#32574=CARTESIAN_POINT('Ctrl Pts',(-9.36166784032156,0.204052005083444,
1.98446420126701));
#32575=CARTESIAN_POINT('Ctrl Pts',(-9.25062832030885,-1.5554913866617,1.24907242900888));
#32576=CARTESIAN_POINT('Ctrl Pts',(-9.13958880029619,-1.89358304816144,
-0.627756821232938));
#32577=CARTESIAN_POINT('Ctrl Pts',(-9.02854928028346,-0.501265320542654,
-1.93092425157233));
#32578=CARTESIAN_POINT('Ctrl Pts',(-8.9175097602708,1.34912273990295,-1.4695588520252));
#32579=CARTESIAN_POINT('Ctrl Pts',(-8.80647024025808,1.96664453738317,0.334730713364926));
#32580=CARTESIAN_POINT('Ctrl Pts',(-8.6954307202454,0.786991304251073,1.83313394871245));
#32581=CARTESIAN_POINT('Ctrl Pts',(-8.5843912002327,-1.11183669301559,1.65636788031917));
#32582=CARTESIAN_POINT('Ctrl Pts',(-8.47335168022002,-1.99463708345048,
-0.0340336923217584));
#32583=CARTESIAN_POINT('Ctrl Pts',(-8.36231216020732,-1.05468206823365,
-1.6933343207516));
#32584=CARTESIAN_POINT('Ctrl Pts',(-8.25127264019463,0.849071051945344,
-1.80521847310438));
#32585=CARTESIAN_POINT('Ctrl Pts',(-8.14023312018193,1.97691919043286,-0.267443267604836));
#32586=CARTESIAN_POINT('Ctrl Pts',(-8.02919360016924,1.29820303168762,1.51472910957899));
#32587=CARTESIAN_POINT('Ctrl Pts',(-7.91815408015655,-0.566847530080274,
1.91269947052086));
#32588=CARTESIAN_POINT('Ctrl Pts',(-7.80711456014386,-1.91389689343126,
0.56279131852139));
#32589=CARTESIAN_POINT('Ctrl Pts',(-7.69607504013116,-1.51197350514412,
-1.30141135181429));
#32590=CARTESIAN_POINT('Ctrl Pts',(-7.58503552011847,0.271633750634426,
-1.97634776605868));
#32591=CARTESIAN_POINT('Ctrl Pts',(-7.47399600010577,1.80701445360575,-0.845242066717456));
#32592=CARTESIAN_POINT('Ctrl Pts',(-7.36295648009308,1.69109458128501,1.05826958003969));
#32593=CARTESIAN_POINT('Ctrl Pts',(-7.25191696008039,0.0298049697366587,
1.99470475275613));
#32594=CARTESIAN_POINT('Ctrl Pts',(-7.1408774400677,-1.6587212605197,1.1083226817082));
#32595=CARTESIAN_POINT('Ctrl Pts',(-7.02983792005499,-1.83146140158355,
-0.790875793913607));
#32596=CARTESIAN_POINT('Ctrl Pts',(-6.91879840004232,-0.330560659462779,
-1.96734974961353));
#32597=CARTESIAN_POINT('Ctrl Pts',(-6.8077588800296,1.47241570028829,-1.34600423195228));
#32598=CARTESIAN_POINT('Ctrl Pts',(-6.69671936001693,1.92985722599114,0.505357768495393));
#32599=CARTESIAN_POINT('Ctrl Pts',(-6.58567984000423,0.623740999761369,
1.8949096422008));
#32600=CARTESIAN_POINT('Ctrl Pts',(-6.47464031999154,-1.2523672758867,1.5528398478842));
#32601=CARTESIAN_POINT('Ctrl Pts',(-6.36360079997884,-1.98402714990627,
-0.208258626048653));
#32602=CARTESIAN_POINT('Ctrl Pts',(-6.25256127996616,-0.902627273630063,
-1.77904451652791));
#32603=CARTESIAN_POINT('Ctrl Pts',(-6.14152175995345,1.00361876436081,-1.72408954602473));
#32604=CARTESIAN_POINT('Ctrl Pts',(-6.03048223994077,1.99272977907838,-0.0936131105300822));
#32605=CARTESIAN_POINT('Ctrl Pts',(-5.91944271992807,1.16082833646465,1.62240961540223));
#32606=CARTESIAN_POINT('Ctrl Pts',(-5.80840319991538,-0.731870653171702,
1.85582885361632));
#32607=CARTESIAN_POINT('Ctrl Pts',(-5.69736367990268,-1.95576567822975,
0.393339546381216));
#32608=CARTESIAN_POINT('Ctrl Pts',(-5.58632415988999,-1.39242707980852,
-1.42859448910627));
#32609=CARTESIAN_POINT('Ctrl Pts',(-5.4752846398773,0.443350504007648,-1.94503874446888));
#32610=CARTESIAN_POINT('Ctrl Pts',(-5.3642451198646,1.87398194144794,-0.684051949793199));
#32611=CARTESIAN_POINT('Ctrl Pts',(-5.25320559985191,1.59211603177235,1.20204073485982));
#32612=CARTESIAN_POINT('Ctrl Pts',(-5.14216607983922,-0.144670237810325,
1.98967482498543));
#32613=CARTESIAN_POINT('Ctrl Pts',(-5.03112655982653,-1.74925277961036,
0.959088160658));
#32614=CARTESIAN_POINT('Ctrl Pts',(-4.92008703981383,-1.75531898661405,
-0.94794021020374));
#32615=CARTESIAN_POINT('Ctrl Pts',(-4.80904751980114,-0.157325388432984,
-1.98871418485495));
#32616=CARTESIAN_POINT('Ctrl Pts',(-4.69800799978845,1.58443656971279,-1.21214526499329));
#32617=CARTESIAN_POINT('Ctrl Pts',(-4.58696847977575,1.87829587613392,0.67211605291583));
#32618=CARTESIAN_POINT('Ctrl Pts',(-4.47592895976307,0.455715640724303,
1.94217883874994));
#32619=CARTESIAN_POINT('Ctrl Pts',(-4.36488943975036,-1.38331035038812,
1.43742403674008));
#32620=CARTESIAN_POINT('Ctrl Pts',(-4.25384991973768,-1.95822847958197,
-0.380889234086341));
#32621=CARTESIAN_POINT('Ctrl Pts',(-4.14281039972498,-0.743662408229242,
-1.85113522182343));
#32622=CARTESIAN_POINT('Ctrl Pts',(-4.03177087971229,1.15048326475978,-1.62976183671034));
#32623=CARTESIAN_POINT('Ctrl Pts',(-3.92073135969959,1.99328500789168,0.0809337025116572));
#32624=CARTESIAN_POINT('Ctrl Pts',(-3.80969183968691,1.01456691000454,1.71766975056653));
#32625=CARTESIAN_POINT('Ctrl Pts',(-3.6986523196742,-0.891290934232011,
1.78475092308452));
#32626=CARTESIAN_POINT('Ctrl Pts',(-3.58761279966152,-1.98266208218415,
0.220876559983982));
#32627=CARTESIAN_POINT('Ctrl Pts',(-3.47657327964882,-1.26222091708206,
-1.54484100908882));
#32628=CARTESIAN_POINT('Ctrl Pts',(-3.36553375963613,0.61167318381939,-1.89883946217874));
#32629=CARTESIAN_POINT('Ctrl Pts',(-3.25449423962344,1.92660314453117,-0.517625067311445));
#32630=CARTESIAN_POINT('Ctrl Pts',(-3.14345471961074,1.4809490244114,1.33660965654155));
#32631=CARTESIAN_POINT('Ctrl Pts',(-3.03241519959805,-0.318037921158636,
1.96941292467288));
#32632=CARTESIAN_POINT('Ctrl Pts',(-2.92137567958535,-1.8263928790374,0.802511331888053));
#32633=CARTESIAN_POINT('Ctrl Pts',(-2.81033615957267,-1.66573871231129,
-1.09774766189583));
#32634=CARTESIAN_POINT('Ctrl Pts',(-2.69929663955997,0.0171142887374011,
-1.99485400211406));
#32635=CARTESIAN_POINT('Ctrl Pts',(-2.58825711954728,1.68432777090903,-1.06900670878697));
#32636=CARTESIAN_POINT('Ctrl Pts',(-2.47721759953459,1.81235521720314,0.833728945586275));
#32637=CARTESIAN_POINT('Ctrl Pts',(-2.36617807952189,0.284201544735738,
1.97457967160987));
#32638=CARTESIAN_POINT('Ctrl Pts',(-2.2551385595092,-1.50366347693917,1.31100400792993));
#32639=CARTESIAN_POINT('Ctrl Pts',(-2.14409903949651,-1.91743858156491,
-0.550603930527132));
#32640=CARTESIAN_POINT('Ctrl Pts',(-2.03305951948381,-0.579004415318382,
-1.90905456620366));
#32641=CARTESIAN_POINT('Ctrl Pts',(-1.92201999947112,1.2885402048375,-1.52295743259934));
#32642=CARTESIAN_POINT('Ctrl Pts',(-1.81098047945842,1.97858067553034,0.254860852426422));
#32643=CARTESIAN_POINT('Ctrl Pts',(-1.69994095944573,0.860538364268268,
1.79978039199151));
#32644=CARTESIAN_POINT('Ctrl Pts',(-1.58890143943304,-1.04388775178742,
1.70000954704084));
#32645=CARTESIAN_POINT('Ctrl Pts',(-1.47786191942035,-1.99438053858907,
0.0467231641033586));
#32646=CARTESIAN_POINT('Ctrl Pts',(-1.36682239940765,-1.12235116649073,
-1.64926196137903));
#32647=CARTESIAN_POINT('Ctrl Pts',(-1.25578287939496,0.775311967462195,
-1.83810174158394));
#32648=CARTESIAN_POINT('Ctrl Pts',(-1.14474335938227,1.96447755503407,-0.347239034000803));
#32649=CARTESIAN_POINT('Ctrl Pts',(-1.03370383936957,1.35844015811823,1.46095287200342));
#32650=CARTESIAN_POINT('Ctrl Pts',(-0.922664319356883,-0.488962413127507,
1.9340613808792));
#32651=CARTESIAN_POINT('Ctrl Pts',(-0.811624799344187,-1.88956708766444,
0.639815197061019));
#32652=CARTESIAN_POINT('Ctrl Pts',(-0.700585279331496,-1.56337577625731,
-1.23919757978839));
#32653=CARTESIAN_POINT('Ctrl Pts',(-0.589545759318804,0.191364756043121,
-1.9856341376312));
#32654=CARTESIAN_POINT('Ctrl Pts',(-0.478506239306104,1.77143531364765,
-0.917851935796283));
#32655=CARTESIAN_POINT('Ctrl Pts',(-0.367466719293418,1.73232926704656,
0.989278326786373));
#32656=CARTESIAN_POINT('Ctrl Pts',(-0.25642719928072,0.110913857831672,
1.99125448516684));
#32657=CARTESIAN_POINT('Ctrl Pts',(-0.14538767926803,-1.61327959277311,
1.17572877042737));
#32658=CARTESIAN_POINT('Ctrl Pts',(-0.0343481592553372,-1.86041677754202,
-0.718533525636265));
#32659=CARTESIAN_POINT('Ctrl Pts',(0.0396781874197904,-0.895860649290834,
-1.53705164209763));
#32660=CARTESIAN_POINT('Ctrl Pts',(0.0766913607573549,-0.346915509926753,
-1.65230719704803));
#32661=CARTESIAN_POINT('Ctrl Pts',(-19.7226913607574,-0.802959149489944,
1.63459616787394));
#32662=CARTESIAN_POINT('Ctrl Pts',(-19.6856781874198,-1.34602016307183,
1.3678294776314));
#32663=CARTESIAN_POINT('Ctrl Pts',(-19.6116518407446,-2.13606885804074,
0.255224265791084));
#32664=CARTESIAN_POINT('Ctrl Pts',(-19.500612320732,-1.37291904283165,-1.65886370728586));
#32665=CARTESIAN_POINT('Ctrl Pts',(-19.3895728007193,0.646613297164265,
-2.05177211691162));
#32666=CARTESIAN_POINT('Ctrl Pts',(-19.2785332807066,2.07434237757899,-0.572352691068324));
#32667=CARTESIAN_POINT('Ctrl Pts',(-19.1674937606939,1.60695496861303,1.43147100709311));
#32668=CARTESIAN_POINT('Ctrl Pts',(-19.0564542406812,-0.329162873365406,
2.12645671837908));
#32669=CARTESIAN_POINT('Ctrl Pts',(-18.9454147206685,-1.96435115072204,
0.878604544751473));
#32670=CARTESIAN_POINT('Ctrl Pts',(-18.8343752006558,-1.80452915818932,
-1.17233980536332));
#32671=CARTESIAN_POINT('Ctrl Pts',(-18.7233356806431,0.00435854303521161,
-2.15186269086486));
#32672=CARTESIAN_POINT('Ctrl Pts',(-18.6122961606304,1.80924422350002,-1.165007873743));
#32673=CARTESIAN_POINT('Ctrl Pts',(-18.5012566406177,1.96080172123412,0.886492714385021));
#32674=CARTESIAN_POINT('Ctrl Pts',(-18.390217120605,0.320518251889661,2.12787619301341));
#32675=CARTESIAN_POINT('Ctrl Pts',(-18.2791776005923,-1.6126610330548,1.42475459323971));
#32676=CARTESIAN_POINT('Ctrl Pts',(-18.1681380805797,-2.07214681351415,
-0.580351970431944));
#32677=CARTESIAN_POINT('Ctrl Pts',(-18.0570985605669,-0.63804585472225,
-2.05511439718916));
#32678=CARTESIAN_POINT('Ctrl Pts',(-17.9460590405543,1.37911892993617,-1.65185670702901));
#32679=CARTESIAN_POINT('Ctrl Pts',(-17.8350195205416,2.13600630168632,0.260914658677094));
#32680=CARTESIAN_POINT('Ctrl Pts',(-17.7239800005289,0.940950993399115,
1.93525455928752));
#32681=CARTESIAN_POINT('Ctrl Pts',(-17.6129404805162,-1.11397171006355,
1.84110464118256));
#32682=CARTESIAN_POINT('Ctrl Pts',(-17.5019009605035,-2.15091579880705,
0.0645014883107155));
#32683=CARTESIAN_POINT('Ctrl Pts',(-17.3908614404908,-1.22229258507502,
-1.77104489031393));
#32684=CARTESIAN_POINT('Ctrl Pts',(-17.2798219204781,0.823295924407405,
-1.98816071553518));
#32685=CARTESIAN_POINT('Ctrl Pts',(-17.1687824004654,2.11653349234182,-0.388439409234132));
#32686=CARTESIAN_POINT('Ctrl Pts',(-17.0577428804527,1.4756232891916,1.56624873558618));
#32687=CARTESIAN_POINT('Ctrl Pts',(-16.94670336044,-0.513752931632555,2.08965478603169));
#32688=CARTESIAN_POINT('Ctrl Pts',(-16.8356638404273,-2.0336472904266,0.70347558284785));
#32689=CARTESIAN_POINT('Ctrl Pts',(-16.7246243204146,-1.6951376201129,-1.32555937092177));
#32690=CARTESIAN_POINT('Ctrl Pts',(-16.613584800402,0.192436431718756,-2.14326093082196));
#32691=CARTESIAN_POINT('Ctrl Pts',(-16.5025452803892,1.90415666588971,-1.0023904375248));
#32692=CARTESIAN_POINT('Ctrl Pts',(-16.3915057603766,1.87580504194971,1.0544925993313));
#32693=CARTESIAN_POINT('Ctrl Pts',(-16.2804662403639,0.133290070461722,
2.14775067330598));
#32694=CARTESIAN_POINT('Ctrl Pts',(-16.1694267203512,-1.73102911217666,
1.27833384149443));
#32695=CARTESIAN_POINT('Ctrl Pts',(-16.0583872003385,-2.01348525930153,
-0.75926036910102));
#32696=CARTESIAN_POINT('Ctrl Pts',(-15.9473476803258,-0.455962008151305,
-2.10302112320607));
#32697=CARTESIAN_POINT('Ctrl Pts',(-15.8363081603131,1.51823213618007,-1.52498209110447));
#32698=CARTESIAN_POINT('Ctrl Pts',(-15.7252686403004,2.10502310014378,0.446628419808841));
#32699=CARTESIAN_POINT('Ctrl Pts',(-15.6142291202877,0.768184815136414,
2.01009733279657));
#32700=CARTESIAN_POINT('Ctrl Pts',(-15.503189600275,-1.27064233588956,1.73668282992772));
#32701=CARTESIAN_POINT('Ctrl Pts',(-15.3921500802623,-2.14832082202336,
-0.12376123456764));
#32702=CARTESIAN_POINT('Ctrl Pts',(-15.2811105602496,-1.06280338449415,
-1.87110880587658));
#32703=CARTESIAN_POINT('Ctrl Pts',(-15.1700710402369,0.993933644962316,
-1.90858458207459));
#32704=CARTESIAN_POINT('Ctrl Pts',(-15.0590315202243,2.14238618535262,-0.201942146000205));
#32705=CARTESIAN_POINT('Ctrl Pts',(-14.9479920002115,1.33306603980161,1.6892406965997));
#32706=CARTESIAN_POINT('Ctrl Pts',(-14.8369524801989,-0.694447305053506,
2.03674793188182));
#32707=CARTESIAN_POINT('Ctrl Pts',(-14.7259129601861,-2.08735519223967,
0.523017685122661));
#32708=CARTESIAN_POINT('Ctrl Pts',(-14.6148734401735,-1.57277926107211,
-1.46866081634339));
#32709=CARTESIAN_POINT('Ctrl Pts',(-14.5038339201608,0.379046545675268,
-2.11823580220253));
#32710=CARTESIAN_POINT('Ctrl Pts',(-14.3927944001481,1.9844889697734,-0.832107400741434));
#32711=CARTESIAN_POINT('Ctrl Pts',(-14.2817548801354,1.77644961960646,1.21442412135177));
#32712=CARTESIAN_POINT('Ctrl Pts',(-14.1707153601227,-0.0549593018331681,
2.15118076243326));
#32713=CARTESIAN_POINT('Ctrl Pts',(-14.05967584011,-1.83614486919079,1.12212798595584));
#32714=CARTESIAN_POINT('Ctrl Pts',(-13.9486363200973,-1.9394096690835,-0.932356869973282));
#32715=CARTESIAN_POINT('Ctrl Pts',(-13.8375968000846,-0.270387426172459,
-2.13482782380425));
#32716=CARTESIAN_POINT('Ctrl Pts',(-13.7265572800719,1.6457224432373,-1.38643313482693));
#32717=CARTESIAN_POINT('Ctrl Pts',(-13.6155177600592,2.05792490788552,0.628923104222863));
#32718=CARTESIAN_POINT('Ctrl Pts',(-13.5044782400466,0.589537774858808,
2.06955174120762));
#32719=CARTESIAN_POINT('Ctrl Pts',(-13.3934387200338,-1.41758553973979,
1.61896585357493));
#32720=CARTESIAN_POINT('Ctrl Pts',(-13.2823992000212,-2.12927936143807,
-0.311076515466602));
#32721=CARTESIAN_POINT('Ctrl Pts',(-13.1713596800084,-0.895177881120831,
-1.95684842506337));
#32722=CARTESIAN_POINT('Ctrl Pts',(-13.0603201599958,1.15696229674745,-1.81439726670479));
#32723=CARTESIAN_POINT('Ctrl Pts',(-12.9492806399831,2.15183782330204,-0.0138989110260861));
#32724=CARTESIAN_POINT('Ctrl Pts',(-12.8382411199704,1.18030349161586,1.79930066003444));
#32725=CARTESIAN_POINT('Ctrl Pts',(-12.7272015999577,-0.869825331019388,
1.96824873708532));
#32726=CARTESIAN_POINT('Ctrl Pts',(-12.616162079945,-2.12508332865939,0.33855582076649));
#32727=CARTESIAN_POINT('Ctrl Pts',(-12.5051225599323,-1.43838047692345,
-1.60051891620387));
#32728=CARTESIAN_POINT('Ctrl Pts',(-12.3940830399196,0.562754865539417,
-2.07699450139683));
#32729=CARTESIAN_POINT('Ctrl Pts',(-12.2830435199069,2.04962900142514,-0.655454158609094));
#32730=CARTESIAN_POINT('Ctrl Pts',(-12.1720039998942,1.66349457203068,1.36505860912468));
#32731=CARTESIAN_POINT('Ctrl Pts',(-12.0609644798815,-0.242787932719905,
2.13814246888428));
#32732=CARTESIAN_POINT('Ctrl Pts',(-11.9499249598688,-1.92720400348909,
0.957331670037384));
#32733=CARTESIAN_POINT('Ctrl Pts',(-11.8388854398561,-1.85048691158961,
-1.09831570486655));
#32734=CARTESIAN_POINT('Ctrl Pts',(-11.7278459198435,-0.0827428909453353,
-2.15029133177786));
#32735=CARTESIAN_POINT('Ctrl Pts',(-11.6168063998307,1.76061390808414,-1.23727032785145));
#32736=CARTESIAN_POINT('Ctrl Pts',(-11.5057668798181,1.9950722539301,0.806403062444103));
#32737=CARTESIAN_POINT('Ctrl Pts',(-11.3947273598054,0.406377523114059,
2.11316267860017));
#32738=CARTESIAN_POINT('Ctrl Pts',(-11.2836878397927,-1.55367640539128,
1.48885487031187));
#32739=CARTESIAN_POINT('Ctrl Pts',(-11.17264831978,-2.09393718452755,-0.496010347446261));
#32740=CARTESIAN_POINT('Ctrl Pts',(-11.0616087997673,-0.720699335838131,
-2.02760737443013));
#32741=CARTESIAN_POINT('Ctrl Pts',(-10.9505692797546,1.31113381379501,-1.70631981757357));
#32742=CARTESIAN_POINT('Ctrl Pts',(-10.8395297597419,2.1448160484289,0.174250727180013));
#32743=CARTESIAN_POINT('Ctrl Pts',(-10.7284902397292,1.018505119976,1.89558606190899));
#32744=CARTESIAN_POINT('Ctrl Pts',(-10.6174507197165,-1.03854440173956,
1.88468159728278));
#32745=CARTESIAN_POINT('Ctrl Pts',(-10.5064111997038,-2.14654287151867,
0.15150213943483));
#32746=CARTESIAN_POINT('Ctrl Pts',(-10.3953716796911,-1.29297015875692,
-1.7201242298407));
#32747=CARTESIAN_POINT('Ctrl Pts',(-10.2843321596785,0.742155010727236,
-2.01985275145824));
#32748=CARTESIAN_POINT('Ctrl Pts',(-10.1732926396657,2.09907808076259,-0.473783081571129));
#32749=CARTESIAN_POINT('Ctrl Pts',(-10.0622531196531,1.53780462756055,1.50524287906447));
#32750=CARTESIAN_POINT('Ctrl Pts',(-9.95121359964035,-0.428757898515473,
2.10873560741539));
#32751=CARTESIAN_POINT('Ctrl Pts',(-9.84017407962767,-2.00350941108974,
0.78520649334798));
#32752=CARTESIAN_POINT('Ctrl Pts',(-9.72913455961497,-1.74739773574985,
-1.25586637450696));
#32753=CARTESIAN_POINT('Ctrl Pts',(-9.61809503960229,0.105535083189655,
-2.14929326610798));
#32754=CARTESIAN_POINT('Ctrl Pts',(-9.50705551958959,1.86202697813056,-1.07863558732083));
#32755=CARTESIAN_POINT('Ctrl Pts',(-9.3960159995769,1.91694630730648,0.977709595138056));
#32756=CARTESIAN_POINT('Ctrl Pts',(-9.2849764795642,0.220106244772615,2.14059628107054));
#32757=CARTESIAN_POINT('Ctrl Pts',(-9.17393695955151,-1.67787308806046,
1.34734594588154));
#32758=CARTESIAN_POINT('Ctrl Pts',(-9.06289743953881,-2.04256485362883,
-0.677146967977541));
#32759=CARTESIAN_POINT('Ctrl Pts',(-8.95185791952613,-0.540703470638638,
-2.08284395823602));
#32760=CARTESIAN_POINT('Ctrl Pts',(-8.84081839951343,1.45526793474034,-1.58517962251523));
#32761=CARTESIAN_POINT('Ctrl Pts',(-8.72977887950073,2.12137461599071,0.361066387456933));
#32762=CARTESIAN_POINT('Ctrl Pts',(-8.61873935948805,0.848909573697069,
1.9773597885075));
#32763=CARTESIAN_POINT('Ctrl Pts',(-8.50769983947535,-1.19931288692809,
1.78668626142621));
#32764=CARTESIAN_POINT('Ctrl Pts',(-8.39666031946266,-2.15156953710398,
-0.0367113678183627));
#32765=CARTESIAN_POINT('Ctrl Pts',(-8.28562079944997,-1.13766149650434,
-1.82656111775448));
#32766=CARTESIAN_POINT('Ctrl Pts',(-8.17458127943727,0.915873581896044,
-1.94724800154111));
#32767=CARTESIAN_POINT('Ctrl Pts',(-8.06354175942458,2.13245764993681,-0.28848495410838));
#32768=CARTESIAN_POINT('Ctrl Pts',(-7.95250223941187,1.40034200663875,1.63390374929613));
#32769=CARTESIAN_POINT('Ctrl Pts',(-7.84146271939921,-0.611445504559457,
2.06318530250556));
#32770=CARTESIAN_POINT('Ctrl Pts',(-7.73042319938648,-2.06447693529353,
0.607070161646897));
#32771=CARTESIAN_POINT('Ctrl Pts',(-7.61938367937381,-1.63093134162977,
-1.40380274839831));
#32772=CARTESIAN_POINT('Ctrl Pts',(-7.50834415936112,0.293005132594524,
-2.13184126749489));
#32773=CARTESIAN_POINT('Ctrl Pts',(-7.39730463934841,1.94918528475322,-0.91174334284516));
#32774=CARTESIAN_POINT('Ctrl Pts',(-7.28626511933573,1.82414516186586,1.14153126368152));
#32775=CARTESIAN_POINT('Ctrl Pts',(-7.17522559932303,0.0321499411956851,
2.15164253044089));
#32776=CARTESIAN_POINT('Ctrl Pts',(-7.06418607931035,-1.7892247989831,1.19552240306272));
#32777=CARTESIAN_POINT('Ctrl Pts',(-6.95314655929764,-1.97555565005957,
-0.853099684115907));
#32778=CARTESIAN_POINT('Ctrl Pts',(-6.84210703928496,-0.356568245404698,
-2.12213531234225));
#32779=CARTESIAN_POINT('Ctrl Pts',(-6.73106751927225,1.58826123959035,-1.45190407132699));
#32780=CARTESIAN_POINT('Ctrl Pts',(-6.62002799925957,2.08169298207356,0.545117900922933));
#32781=CARTESIAN_POINT('Ctrl Pts',(-6.50898847924688,0.672815192931128,
2.04399582036804));
#32782=CARTESIAN_POINT('Ctrl Pts',(-6.39794895923417,-1.35090002207445,
1.67501293364566));
#32783=CARTESIAN_POINT('Ctrl Pts',(-6.28690943922149,-2.14012484373404,
-0.224643830881916));
#32784=CARTESIAN_POINT('Ctrl Pts',(-6.17586991920879,-0.973643456955139,
-1.91901475144131));
#32785=CARTESIAN_POINT('Ctrl Pts',(-6.0648303991961,1.08258067504153,-1.85973607792815));
#32786=CARTESIAN_POINT('Ctrl Pts',(-5.95379087918341,2.14951217137112,-0.10097832761718));
#32787=CARTESIAN_POINT('Ctrl Pts',(-5.84275135917072,1.25215905553298,1.75005625542945));
#32788=CARTESIAN_POINT('Ctrl Pts',(-5.73171183915802,-0.789452184324518,
2.00184026490282));
#32789=CARTESIAN_POINT('Ctrl Pts',(-5.62067231914534,-2.10963983869857,
0.424286399141893));
#32790=CARTESIAN_POINT('Ctrl Pts',(-5.50963279913263,-1.50197933870362,
-1.54099229836765));
#32791=CARTESIAN_POINT('Ctrl Pts',(-5.39859327911995,0.478232078705997,
-2.09806893986292));
#32792=CARTESIAN_POINT('Ctrl Pts',(-5.28755375910724,2.02142158679187,-0.737871239426468));
#32793=CARTESIAN_POINT('Ctrl Pts',(-5.17651423909456,1.71737925756923,1.29661392989273));
#32794=CARTESIAN_POINT('Ctrl Pts',(-5.06547471908186,-0.156052486530463,
2.14621686205486));
#32795=CARTESIAN_POINT('Ctrl Pts',(-4.95443519906917,-1.88687908418583,
1.0345465282833));
#32796=CARTESIAN_POINT('Ctrl Pts',(-4.84339567905648,-1.89342256334962,
-1.02252148834121));
#32797=CARTESIAN_POINT('Ctrl Pts',(-4.73235615904378,-0.169703308924683,
-2.14518064145213));
#32798=CARTESIAN_POINT('Ctrl Pts',(-4.62131663903109,1.70909559696464,-1.30751345612848));
#32799=CARTESIAN_POINT('Ctrl Pts',(-4.5102771190184,2.02607492976459,0.724996259645748));
#32800=CARTESIAN_POINT('Ctrl Pts',(-4.39923759900571,0.491570069713157,
2.09498402477993));
#32801=CARTESIAN_POINT('Ctrl Pts',(-4.28819807899301,-1.49214533057168,
1.55051653005515));
#32802=CARTESIAN_POINT('Ctrl Pts',(-4.17715855898032,-2.11229640635658,
-0.41085653118081));
#32803=CARTESIAN_POINT('Ctrl Pts',(-4.06611903896763,-0.802171681611132,
-1.99677735131931));
#32804=CARTESIAN_POINT('Ctrl Pts',(-3.95507951895493,1.24100006258937,-1.7579869288977));
#32805=CARTESIAN_POINT('Ctrl Pts',(-3.84403999894224,2.15011108403084,0.0873013393233009));
#32806=CARTESIAN_POINT('Ctrl Pts',(-3.73300047892955,1.09439019009076,1.85281119096156));
#32807=CARTESIAN_POINT('Ctrl Pts',(-3.62196095891685,-0.961415206155314,
1.92517012206756));
#32808=CARTESIAN_POINT('Ctrl Pts',(-3.51092143890416,-2.13865237631059,
0.238254508484187));
#32809=CARTESIAN_POINT('Ctrl Pts',(-3.39988191889147,-1.36152892013381,
-1.66638476863905));
#32810=CARTESIAN_POINT('Ctrl Pts',(-3.28884239887877,0.659797915063637,
-2.04823482756436));
#32811=CARTESIAN_POINT('Ctrl Pts',(-3.17780287886608,2.07818287860732,-0.558350356417769));
#32812=CARTESIAN_POINT('Ctrl Pts',(-3.06676335885339,1.59746594173181,1.44177035706117));
#32813=CARTESIAN_POINT('Ctrl Pts',(-2.9557238388407,-0.343060253158991,
2.12436081223105));
#32814=CARTESIAN_POINT('Ctrl Pts',(-2.844684318828,-1.97008835036937,0.865650673597296));
#32815=CARTESIAN_POINT('Ctrl Pts',(-2.73364479881531,-1.79679436420783,
-1.18411537033918));
#32816=CARTESIAN_POINT('Ctrl Pts',(-2.62260527880261,0.0184607929944456,
-2.15180352231987));
#32817=CARTESIAN_POINT('Ctrl Pts',(-2.51156575878993,1.81684595782065,-1.1531131596165));
#32818=CARTESIAN_POINT('Ctrl Pts',(-2.40052623877722,1.95494624465731,0.899324401621065));
#32819=CARTESIAN_POINT('Ctrl Pts',(-2.28948671876454,0.30656172550121,2.1299340643318));
#32820=CARTESIAN_POINT('Ctrl Pts',(-2.17844719875184,-1.6219675037033,1.41415012780357));
#32821=CARTESIAN_POINT('Ctrl Pts',(-2.06740767873915,-2.06829727352021,
-0.593923904133282));
#32822=CARTESIAN_POINT('Ctrl Pts',(-1.95636815872646,-0.624558859445587,
-2.05925362733538));
#32823=CARTESIAN_POINT('Ctrl Pts',(-1.84532863871376,1.38991893566234,-1.64277945370315));
#32824=CARTESIAN_POINT('Ctrl Pts',(-1.73428911870107,2.13424985602369,0.274912589779238));
#32825=CARTESIAN_POINT('Ctrl Pts',(-1.62324959868838,0.928243110203279,
1.94138206745225));
#32826=CARTESIAN_POINT('Ctrl Pts',(-1.51221007867568,-1.12601791350259,
1.83376153213378));
#32827=CARTESIAN_POINT('Ctrl Pts',(-1.40117055866299,-2.15129280801212,
0.0503992116640912));
#32828=CARTESIAN_POINT('Ctrl Pts',(-1.2901310386503,-1.21065460969833,-1.7790212687057));
#32829=CARTESIAN_POINT('Ctrl Pts',(-1.17909151863761,0.836311339433325,
-1.98271843339464));
#32830=CARTESIAN_POINT('Ctrl Pts',(-1.06805199862491,2.11903714154564,-0.374558827692656));
#32831=CARTESIAN_POINT('Ctrl Pts',(-0.95701247861222,1.46531842129889,1.57589654811268));
#32832=CARTESIAN_POINT('Ctrl Pts',(-0.845972958599524,-0.527432604959965,
2.08622790808164));
#32833=CARTESIAN_POINT('Ctrl Pts',(-0.734933438586833,-2.03823292861889,
0.690154063009435));
#32834=CARTESIAN_POINT('Ctrl Pts',(-0.623893918574141,-1.68637779932512,
-1.33669417120906));
#32835=CARTESIAN_POINT('Ctrl Pts',(-0.512854398561449,0.206420798547222,
-2.14185826474789));
#32836=CARTESIAN_POINT('Ctrl Pts',(-0.401814878548749,1.91080687781125,
-0.990065952857435));
#32837=CARTESIAN_POINT('Ctrl Pts',(-0.290775358536063,1.86862407709947,
1.06711197204293));
#32838=CARTESIAN_POINT('Ctrl Pts',(-0.179735838523365,0.119640249212883,
2.14792080547069));
#32839=CARTESIAN_POINT('Ctrl Pts',(-0.0686963185106752,-1.74020790821638,
1.26823181386572));
#32840=CARTESIAN_POINT('Ctrl Pts',(0.0423432015020179,-2.0067891538205,
-0.775065728985946));
#32841=CARTESIAN_POINT('Ctrl Pts',(0.116369548177145,-0.966344453583496,
-1.65798255609091));
#32842=CARTESIAN_POINT('Ctrl Pts',(0.15338272151471,-0.374209849651479,
-1.78230609497965));
#32843=CARTESIAN_POINT('Ctrl Pts',(-19.646,-0.861525859670562,1.75382131162753));
#32844=CARTESIAN_POINT('Ctrl Pts',(-19.6089868266624,-1.44419697921243,
1.46759703447886));
#32845=CARTESIAN_POINT('Ctrl Pts',(-19.5349604799873,-2.29187071398093,
0.273839964503935));
#32846=CARTESIAN_POINT('Ctrl Pts',(-19.4239209599746,-1.47305782540113,
-1.77985889120705));
#32847=CARTESIAN_POINT('Ctrl Pts',(-19.3128814399619,0.693776360936581,
-2.20142548720342));
#32848=CARTESIAN_POINT('Ctrl Pts',(-19.2018419199492,2.22564199091573,-0.614099290755457));
#32849=CARTESIAN_POINT('Ctrl Pts',(-19.0908023999365,1.72416400219814,1.53588048752263));
#32850=CARTESIAN_POINT('Ctrl Pts',(-18.9797628799238,-0.353171550044496,
2.28155747838165));
#32851=CARTESIAN_POINT('Ctrl Pts',(-18.8687233599112,-2.10762815878697,
0.942688723589834));
#32852=CARTESIAN_POINT('Ctrl Pts',(-18.7576838398985,-1.93614897507197,
-1.25784862067171));
#32853=CARTESIAN_POINT('Ctrl Pts',(-18.6466443198858,0.00467644902946805,
-2.30881652674107));
#32854=CARTESIAN_POINT('Ctrl Pts',(-18.5356047998731,1.9412079506099,-1.24998190827883));
#32855=CARTESIAN_POINT('Ctrl Pts',(-18.4245652798604,2.10381983890809,0.951152245213705));
#32856=CARTESIAN_POINT('Ctrl Pts',(-18.3135257598477,0.343896402045778,
2.28308048749787));
#32857=CARTESIAN_POINT('Ctrl Pts',(-18.202486239835,-1.73028625894889,1.52867418789625));
#32858=CARTESIAN_POINT('Ctrl Pts',(-18.0914467198223,-2.2232862854983,-0.622682026296723));
#32859=CARTESIAN_POINT('Ctrl Pts',(-17.9804071998096,-0.684584021301682,
-2.20501154870007));
#32860=CARTESIAN_POINT('Ctrl Pts',(-17.8693676797969,1.4797099235446,-1.77234081021396));
#32861=CARTESIAN_POINT('Ctrl Pts',(-17.7583281597842,2.29180359485407,0.279945406637725));
#32862=CARTESIAN_POINT('Ctrl Pts',(-17.6472886397715,1.0095826344478,2.07640930292734));
#32863=CARTESIAN_POINT('Ctrl Pts',(-17.5362491197588,-1.19522323865519,
1.97539222231392));
#32864=CARTESIAN_POINT('Ctrl Pts',(-17.4252095997461,-2.30780056970933,
0.0692061360807777));
#32865=CARTESIAN_POINT('Ctrl Pts',(-17.3141700797335,-1.31144488582588,
-1.90022241182763));
#32866=CARTESIAN_POINT('Ctrl Pts',(-17.2031305597207,0.883345970326033,
-2.13317435974508));
#32867=CARTESIAN_POINT('Ctrl Pts',(-17.0920910397081,2.2709104662044,-0.416771633006387));
#32868=CARTESIAN_POINT('Ctrl Pts',(-16.9810515196954,1.58325317493202,1.68048871382927));
#32869=CARTESIAN_POINT('Ctrl Pts',(-16.8700119996827,-0.55122534734696,
2.2420712648884));
#32870=CARTESIAN_POINT('Ctrl Pts',(-16.75897247967,-2.18197866138569,0.754786101702939));
#32871=CARTESIAN_POINT('Ctrl Pts',(-16.6479329596573,-1.81877857217932,
-1.42224380568198));
#32872=CARTESIAN_POINT('Ctrl Pts',(-16.5368934396446,0.206472474189701,
-2.2995873664278));
#32873=CARTESIAN_POINT('Ctrl Pts',(-16.4258539196319,2.04304317295608,-1.0755033851506));
#32874=CARTESIAN_POINT('Ctrl Pts',(-16.3148143996192,2.01262362147143,1.13140580530432));
#32875=CARTESIAN_POINT('Ctrl Pts',(-16.2037748796065,0.143012060592391,
2.3044045844092));
#32876=CARTESIAN_POINT('Ctrl Pts',(-16.0927353595938,-1.85728793915615,
1.37157371260918));
#32877=CARTESIAN_POINT('Ctrl Pts',(-15.9816958395811,-2.16034604008886,
-0.814639751747095));
#32878=CARTESIAN_POINT('Ctrl Pts',(-15.8706563195684,-0.489219235248991,
-2.25641252388286));
#32879=CARTESIAN_POINT('Ctrl Pts',(-15.7596167995557,1.62896985124693,-1.63621213838278));
#32880=CARTESIAN_POINT('Ctrl Pts',(-15.648577279543,2.25856052220058,0.479204868110092));
#32881=CARTESIAN_POINT('Ctrl Pts',(-15.5375377595304,0.82421513431492,2.15671100299323));
#32882=CARTESIAN_POINT('Ctrl Pts',(-15.4264982395177,-1.36332119941149,
1.86335403112222));
#32883=CARTESIAN_POINT('Ctrl Pts',(-15.315458719505,-2.30501631897153,-0.132788204820276));
#32884=CARTESIAN_POINT('Ctrl Pts',(-15.2044191994923,-1.1403227674393,-2.00758484854921));
#32885=CARTESIAN_POINT('Ctrl Pts',(-15.0933796794796,1.06642976604176,-2.04779405511507));
#32886=CARTESIAN_POINT('Ctrl Pts',(-14.9823401594669,2.29864881825516,-0.216671521891302));
#32887=CARTESIAN_POINT('Ctrl Pts',(-14.8713006394542,1.43029800042407,1.81245153536515));
#32888=CARTESIAN_POINT('Ctrl Pts',(-14.7602611194415,-0.74509931403381,
2.18530545926443));
#32889=CARTESIAN_POINT('Ctrl Pts',(-14.6492215994288,-2.23960394196192,
0.561165858916255));
#32890=CARTESIAN_POINT('Ctrl Pts',(-14.5381820794161,-1.68749556665226,
-1.57578286911412));
#32891=CARTESIAN_POINT('Ctrl Pts',(-14.4271425594034,0.406693667200237,
-2.27273694015031));
#32892=CARTESIAN_POINT('Ctrl Pts',(-14.3161030393907,2.12923480201551,-0.892800143341485));
#32893=CARTESIAN_POINT('Ctrl Pts',(-14.205063519378,1.90602135446747,1.30300250743372));
#32894=CARTESIAN_POINT('Ctrl Pts',(-14.0940239993654,-0.0589679559524329,
2.3080848594095));
#32895=CARTESIAN_POINT('Ctrl Pts',(-13.9829844793526,-1.97007069153408,
1.20397442183089));
#32896=CARTESIAN_POINT('Ctrl Pts',(-13.87194495934,-2.08086748058341,-1.00036166775573));
#32897=CARTESIAN_POINT('Ctrl Pts',(-13.7609054393273,-0.290109104461037,
-2.29053916045402));
#32898=CARTESIAN_POINT('Ctrl Pts',(-13.6498659193146,1.76575912185542,-1.48755761624515));
#32899=CARTESIAN_POINT('Ctrl Pts',(-13.5388263993019,2.20802705409076,0.674795870221375));
#32900=CARTESIAN_POINT('Ctrl Pts',(-13.4277868792892,0.632537830369223,
2.22050193227036));
#32901=CARTESIAN_POINT('Ctrl Pts',(-13.3167473592765,-1.52098223372466,
1.73705094420357));
#32902=CARTESIAN_POINT('Ctrl Pts',(-13.2057078392638,-2.28458600105243,
-0.333765998657508));
#32903=CARTESIAN_POINT('Ctrl Pts',(-13.0946683192511,-0.960470895786627,
-2.09957819487902));
#32904=CARTESIAN_POINT('Ctrl Pts',(-12.9836287992384,1.24134949822159,-1.94673684953298));
#32905=CARTESIAN_POINT('Ctrl Pts',(-12.8725892792257,2.30878984537321,-0.0149126780332815));
#32906=CARTESIAN_POINT('Ctrl Pts',(-12.761549759213,1.26639316699041,1.93053911762093));
#32907=CARTESIAN_POINT('Ctrl Pts',(-12.6505102392003,-0.933269166365103,
2.11181002961364));
#32908=CARTESIAN_POINT('Ctrl Pts',(-12.5394707191876,-2.28008391554889,
0.363249605808196));
#32909=CARTESIAN_POINT('Ctrl Pts',(-12.428431199175,-1.54329392435714,-1.71725851318516));
#32910=CARTESIAN_POINT('Ctrl Pts',(-12.3173916791623,0.603801413341659,
-2.2284875569119));
#32911=CARTESIAN_POINT('Ctrl Pts',(-12.2063521591496,2.19912605588985,-0.703262062371451));
#32912=CARTESIAN_POINT('Ctrl Pts',(-12.0953126391369,1.7848275247083,1.46462406272333));
#32913=CARTESIAN_POINT('Ctrl Pts',(-11.9842731191242,-0.260496542802998,
2.29409557108074));
#32914=CARTESIAN_POINT('Ctrl Pts',(-11.8732335991115,-2.0677715509203,1.02715809458389));
#32915=CARTESIAN_POINT('Ctrl Pts',(-11.7621940790988,-1.9854588223187,-1.1784253064753));
#32916=CARTESIAN_POINT('Ctrl Pts',(-11.6511545590861,-0.0887780409483811,
-2.30713055493398));
#32917=CARTESIAN_POINT('Ctrl Pts',(-11.5401150390734,1.88903060843585,-1.32751508407891));
#32918=CARTESIAN_POINT('Ctrl Pts',(-11.4290755190607,2.14059001602237,0.865220966788218));
#32919=CARTESIAN_POINT('Ctrl Pts',(-11.318035999048,0.436018127664415,2.26729379005294));
#32920=CARTESIAN_POINT('Ctrl Pts',(-11.2069964790353,-1.6669993755658,1.59744984895545));
#32921=CARTESIAN_POINT('Ctrl Pts',(-11.0959569590226,-2.24666601550298,
-0.53218864404321));
#32922=CARTESIAN_POINT('Ctrl Pts',(-10.9849174390099,-0.773266130993508,
-2.17549820241776));
#32923=CARTESIAN_POINT('Ctrl Pts',(-10.8738779189972,1.40676606872269,-1.83077638338358));
#32924=CARTESIAN_POINT('Ctrl Pts',(-10.7628383989846,2.30125591212414,0.186960329958694));
#32925=CARTESIAN_POINT('Ctrl Pts',(-10.6517988789719,1.09279344985801,2.03384744118433));
#32926=CARTESIAN_POINT('Ctrl Pts',(-10.5407593589592,-1.11429436862769,
2.02214762025654));
#32927=CARTESIAN_POINT('Ctrl Pts',(-10.4297198389465,-2.30310868725953,
0.162552492242497));
#32928=CARTESIAN_POINT('Ctrl Pts',(-10.3186803189338,-1.38727758225186,
-1.84558767005147));
#32929=CARTESIAN_POINT('Ctrl Pts',(-10.2076407989211,0.796286752609709,
-2.1671779681611));
#32930=CARTESIAN_POINT('Ctrl Pts',(-10.0966012789084,2.25218188147347,-0.508340152680491));
#32931=CARTESIAN_POINT('Ctrl Pts',(-9.9855617588957,1.64996993259997,1.615033176));
#32932=CARTESIAN_POINT('Ctrl Pts',(-9.87452223888301,-0.460030896146754,
2.26254381452713));
#32933=CARTESIAN_POINT('Ctrl Pts',(-9.7634827188703,-2.14964256754975,0.842478349776842));
#32934=CARTESIAN_POINT('Ctrl Pts',(-9.65244319885763,-1.87485046709354,
-1.34746750020314));
#32935=CARTESIAN_POINT('Ctrl Pts',(-9.54140367884492,0.113232663614504,
-2.30605969175894));
#32936=CARTESIAN_POINT('Ctrl Pts',(-9.43036415883224,1.99784060507026,-1.15730974885597));
#32937=CARTESIAN_POINT('Ctrl Pts',(-9.31932463881954,2.05676567281605,1.04902235685904));
#32938=CARTESIAN_POINT('Ctrl Pts',(-9.20828511880685,0.23616048446179,2.29672836087408));
#32939=CARTESIAN_POINT('Ctrl Pts',(-9.09724559879414,-1.80025478945923,
1.44561946275418));
#32940=CARTESIAN_POINT('Ctrl Pts',(-8.98620607878147,-2.19154665909622,
-0.726537114722142));
#32941=CARTESIAN_POINT('Ctrl Pts',(-8.87516655876876,-0.580141620734622,
-2.23476366489971));
#32942=CARTESIAN_POINT('Ctrl Pts',(-8.76412703875608,1.56141312957773,-1.70080039300526));
#32943=CARTESIAN_POINT('Ctrl Pts',(-8.65308751874337,2.27610469459825,0.387402061548938));
#32944=CARTESIAN_POINT('Ctrl Pts',(-8.54204799873069,0.910827843143066,
2.12158562830256));
#32945=CARTESIAN_POINT('Ctrl Pts',(-8.431008478718,-1.28678908084058,1.91700464253325));
#32946=CARTESIAN_POINT('Ctrl Pts',(-8.3199689587053,-2.30850199075749,-0.0393890433149694));
#32947=CARTESIAN_POINT('Ctrl Pts',(-8.20892943869261,-1.22064092477503,
-1.95978791475735));
#32948=CARTESIAN_POINT('Ctrl Pts',(-8.09788991867992,0.982676111846747,
-2.08927752997785));
#32949=CARTESIAN_POINT('Ctrl Pts',(-7.98685039866722,2.28799610944076,-0.309526640611922));
#32950=CARTESIAN_POINT('Ctrl Pts',(-7.87581087865452,1.50248098158987,1.75307838901326));
#32951=CARTESIAN_POINT('Ctrl Pts',(-7.76477135864184,-0.656043479038643,
2.21367113449027));
#32952=CARTESIAN_POINT('Ctrl Pts',(-7.65373183862914,-2.2150569771558,0.651349004772403));
#32953=CARTESIAN_POINT('Ctrl Pts',(-7.54269231861645,-1.74988917811544,
-1.50619414498233));
#32954=CARTESIAN_POINT('Ctrl Pts',(-7.43165279860375,0.314376514554623,
-2.2873347689311));
#32955=CARTESIAN_POINT('Ctrl Pts',(-7.32061327859107,2.09135611590069,-0.978244618972865));
#32956=CARTESIAN_POINT('Ctrl Pts',(-7.20957375857837,1.95719574244671,1.22479294732335));
#32957=CARTESIAN_POINT('Ctrl Pts',(-7.09853423856569,0.0344949126547129,
2.30858030812565));
#32958=CARTESIAN_POINT('Ctrl Pts',(-6.98749471855298,-1.91972833744651,
1.28272212441724));
#32959=CARTESIAN_POINT('Ctrl Pts',(-6.87645519854029,-2.11964989853558,
-0.915323574318207));
#32960=CARTESIAN_POINT('Ctrl Pts',(-6.76541567852761,-0.382575831346619,
-2.27692087507098));
#32961=CARTESIAN_POINT('Ctrl Pts',(-6.65437615851489,1.70410677889241,-1.5578039107017));
#32962=CARTESIAN_POINT('Ctrl Pts',(-6.54333663850222,2.23352873815598,0.584878033350475));
#32963=CARTESIAN_POINT('Ctrl Pts',(-6.43229711848952,0.721889386100885,
2.19308199853527));
#32964=CARTESIAN_POINT('Ctrl Pts',(-6.32125759847682,-1.44943276826219,
1.79718601940713));
#32965=CARTESIAN_POINT('Ctrl Pts',(-6.21021807846414,-2.29622253756181,
-0.241029035715179));
#32966=CARTESIAN_POINT('Ctrl Pts',(-6.09917855845143,-1.04465964028021,
-2.05898498635472));
#32967=CARTESIAN_POINT('Ctrl Pts',(-5.98813903843876,1.16154258572225,-1.99538260983157));
#32968=CARTESIAN_POINT('Ctrl Pts',(-5.87709951842604,2.30629456366387,-0.108343544704277));
#32969=CARTESIAN_POINT('Ctrl Pts',(-5.76605999841337,1.34348977460131,1.87770289545666));
#32970=CARTESIAN_POINT('Ctrl Pts',(-5.65502047840067,-0.847033715477332,
2.14785167618931));
#32971=CARTESIAN_POINT('Ctrl Pts',(-5.54398095838797,-2.26351399916739,
0.455233251902571));
#32972=CARTESIAN_POINT('Ctrl Pts',(-5.43294143837529,-1.61153159759871,
-1.65339010762904));
#32973=CARTESIAN_POINT('Ctrl Pts',(-5.32190191836258,0.513113653404346,
-2.25109913525696));
#32974=CARTESIAN_POINT('Ctrl Pts',(-5.2108623983499,2.16886123213581,-0.791690529059738));
#32975=CARTESIAN_POINT('Ctrl Pts',(-5.0998228783372,1.84264248336612,1.39118712492565));
#32976=CARTESIAN_POINT('Ctrl Pts',(-4.98878335832451,-0.167434735250603,
2.3027588991243));
#32977=CARTESIAN_POINT('Ctrl Pts',(-4.87774383831182,-2.0245053887613,1.1100048959086));
#32978=CARTESIAN_POINT('Ctrl Pts',(-4.76670431829912,-2.03152614008519,
-1.09710276647867));
#32979=CARTESIAN_POINT('Ctrl Pts',(-4.65566479828643,-0.182081229416383,
-2.30164709804931));
#32980=CARTESIAN_POINT('Ctrl Pts',(-4.54462527827374,1.83375462421648,-1.40288164726367));
#32981=CARTESIAN_POINT('Ctrl Pts',(-4.43358575826104,2.17385398339526,0.777876466375666));
#32982=CARTESIAN_POINT('Ctrl Pts',(-4.32254623824835,0.527424498702014,
2.24778921080992));
#32983=CARTESIAN_POINT('Ctrl Pts',(-4.21150671823566,-1.60098031075524,
1.66360902337022));
#32984=CARTESIAN_POINT('Ctrl Pts',(-4.10046719822296,-2.26636433313119,
-0.44082382827528));
#32985=CARTESIAN_POINT('Ctrl Pts',(-3.98942767821027,-0.860680954993021,
-2.1424194808152));
#32986=CARTESIAN_POINT('Ctrl Pts',(-3.87838815819758,1.33151686041895,-1.88621202108507));
#32987=CARTESIAN_POINT('Ctrl Pts',(-3.76734863818489,2.30693716017,0.093668976134945));
#32988=CARTESIAN_POINT('Ctrl Pts',(-3.65630911817219,1.17421347017698,1.98795263135658));
#32989=CARTESIAN_POINT('Ctrl Pts',(-3.5452695981595,-1.03153947807862,2.06558932105061));
#32990=CARTESIAN_POINT('Ctrl Pts',(-3.4342300781468,-2.29464267043703,0.255632456984391));
#32991=CARTESIAN_POINT('Ctrl Pts',(-3.32319055813411,-1.46083692318556,
-1.78792852818929));
#32992=CARTESIAN_POINT('Ctrl Pts',(-3.21215103812142,0.707922646307885,
-2.19763019294999));
#32993=CARTESIAN_POINT('Ctrl Pts',(-3.10111151810873,2.22976261268347,-0.599075645524091));
#32994=CARTESIAN_POINT('Ctrl Pts',(-2.99007199809603,1.71398285905222,1.54693105758079));
#32995=CARTESIAN_POINT('Ctrl Pts',(-2.87903247808334,-0.36808258515935,
2.27930869978922));
#32996=CARTESIAN_POINT('Ctrl Pts',(-2.76799295807064,-2.11378382170134,
0.928790015306536));
#32997=CARTESIAN_POINT('Ctrl Pts',(-2.65695343805796,-1.92785001610438,
-1.27048307878253));
#32998=CARTESIAN_POINT('Ctrl Pts',(-2.54591391804526,0.0198072972514943,
-2.30875304252568));
#32999=CARTESIAN_POINT('Ctrl Pts',(-2.43487439803257,1.94936414473225,-1.23721961044602));
#33000=CARTESIAN_POINT('Ctrl Pts',(-2.32383487801987,2.09753727211149,0.964919857655855));
#33001=CARTESIAN_POINT('Ctrl Pts',(-2.21279535800718,0.328921906266679,
2.28528845705372));
#33002=CARTESIAN_POINT('Ctrl Pts',(-2.10175583799449,-1.74027153046743,
1.51729624767722));
#33003=CARTESIAN_POINT('Ctrl Pts',(-1.9907163179818,-2.21915596547551,-0.637243877739432));
#33004=CARTESIAN_POINT('Ctrl Pts',(-1.8796767979691,-0.670113303572792,
-2.2094526884671));
#33005=CARTESIAN_POINT('Ctrl Pts',(-1.76863727795641,1.49129766648718,-1.76260147480695));
#33006=CARTESIAN_POINT('Ctrl Pts',(-1.65759775794372,2.28991903651704,0.294964327132055));
#33007=CARTESIAN_POINT('Ctrl Pts',(-1.54655823793102,0.995947856138289,
2.08298374291299));
#33008=CARTESIAN_POINT('Ctrl Pts',(-1.43551871791833,-1.20814807521776,
1.96751351722672));
#33009=CARTESIAN_POINT('Ctrl Pts',(-1.32447919790564,-2.30820507743518,
0.0540752592248201));
#33010=CARTESIAN_POINT('Ctrl Pts',(-1.21343967789294,-1.29895805290592,
-1.90878057603237));
#33011=CARTESIAN_POINT('Ctrl Pts',(-1.10240015788025,0.897310711404452,
-2.12733512520534));
#33012=CARTESIAN_POINT('Ctrl Pts',(-0.991360637867558,2.27359672805721,
-0.401878621384507));
#33013=CARTESIAN_POINT('Ctrl Pts',(-0.880321117854865,1.57219668447955,
1.69084022422195));
#33014=CARTESIAN_POINT('Ctrl Pts',(-0.769281597842169,-0.565902796792421,
2.23839443528408));
#33015=CARTESIAN_POINT('Ctrl Pts',(-0.658242077829478,-2.18689876957334,
0.740492928957852));
#33016=CARTESIAN_POINT('Ctrl Pts',(-0.547202557816786,-1.80937982239294,
-1.43419076262974));
#33017=CARTESIAN_POINT('Ctrl Pts',(-0.436163037804094,0.221476841051321,
-2.29808239186457));
#33018=CARTESIAN_POINT('Ctrl Pts',(-0.325123517791394,2.05017844197486,
-1.06227996991859));
#33019=CARTESIAN_POINT('Ctrl Pts',(-0.214083997778708,2.00491888715238,
1.14494561729948));
#33020=CARTESIAN_POINT('Ctrl Pts',(-0.10304447776601,0.128366640594097,
2.30458712577454));
#33021=CARTESIAN_POINT('Ctrl Pts',(0.00799504224667972,-1.86713622365964,
1.36073485730407));
#33022=CARTESIAN_POINT('Ctrl Pts',(0.119034562259373,-2.15316153009897,
-0.831597932335627));
#33023=CARTESIAN_POINT('Ctrl Pts',(0.1930609089345,-1.03682825787616,-1.77891347008418));
#33024=CARTESIAN_POINT('Ctrl Pts',(0.230074082272065,-0.401504189376206,
-1.91230499291127));
#33025=CARTESIAN_POINT('',(-3.47334515779567E-15,-1.49576112924109,1.26226672651054));
#33026=CARTESIAN_POINT('Ctrl Pts',(1.30451205393456E-15,-1.49576882860604,
1.26227079838504));
#33027=CARTESIAN_POINT('Ctrl Pts',(1.26307732327094E-15,-1.52238887744143,
1.22395926652586));
#33028=CARTESIAN_POINT('Ctrl Pts',(5.84589016432815E-15,-1.54749918699467,
1.18468636375502));
#33029=CARTESIAN_POINT('Ctrl Pts',(6.21724893790088E-15,-1.57101022548392,
1.14448601145151));
#33030=CARTESIAN_POINT('Ctrl Pts',(6.79018338235568E-15,-1.60728319042775,
1.08246467749374));
#33031=CARTESIAN_POINT('Ctrl Pts',(9.85209575142001E-15,-1.63975192740418,
1.01823590395021));
#33032=CARTESIAN_POINT('Ctrl Pts',(1.33504318711175E-14,-1.66840521532328,
0.952176670234068));
#33033=CARTESIAN_POINT('Ctrl Pts',(1.5040522558895E-14,-1.68224798326476,
0.920262613972653));
#33034=CARTESIAN_POINT('Ctrl Pts',(2.12362379568834E-16,-1.69519946625923,
0.887921168479435));
#33035=CARTESIAN_POINT('Ctrl Pts',(-2.77555756156289E-17,-1.70725413156156,
0.85519453645218));
#33036=CARTESIAN_POINT('Ctrl Pts',(-1.29001408656712E-16,-1.71233698606792,
0.841395338804994));
#33037=CARTESIAN_POINT('Ctrl Pts',(4.27514254701297E-15,-1.71726036257382,
0.827527661185538));
#33038=CARTESIAN_POINT('Ctrl Pts',(3.94129173741931E-15,-1.72202369968651,
0.813594684328385));
#33039=CARTESIAN_POINT('Ctrl Pts',(3.62096552284113E-15,-1.72659406975068,
0.800226144830491));
#33040=CARTESIAN_POINT('Ctrl Pts',(2.32644902118985E-15,-1.73101538799027,
0.786802333572161));
#33041=CARTESIAN_POINT('Ctrl Pts',(2.63677968348475E-15,-1.73528526710846,
0.773333511905552));
#33042=CARTESIAN_POINT('Ctrl Pts',(4.20467166006644E-15,-1.75685809256139,
0.705284620864877));
#33043=CARTESIAN_POINT('Ctrl Pts',(1.47365000165689E-15,-1.77458920356206,
0.636029775253738));
#33044=CARTESIAN_POINT('Ctrl Pts',(1.36002320516582E-15,-1.78846506651383,
0.565940828545306));
#33045=CARTESIAN_POINT('Ctrl Pts',(1.27834854242507E-15,-1.79843900278432,
0.51556106548726));
#33046=CARTESIAN_POINT('Ctrl Pts',(6.37284015678416E-15,-1.80641993884282,
0.46475008199631));
#33047=CARTESIAN_POINT('Ctrl Pts',(6.07847105982273E-15,-1.81238629657331,
0.413647700170702));
#33048=CARTESIAN_POINT('Ctrl Pts',(5.9169951520491E-15,-1.81565913682923,
0.385615533819469));
#33049=CARTESIAN_POINT('Ctrl Pts',(3.8882620403915E-15,-1.81832553753825,
0.357495735434968));
#33050=CARTESIAN_POINT('Ctrl Pts',(4.413136522885E-15,-1.82038020010595,
0.329311981061615));
#33051=CARTESIAN_POINT('Ctrl Pts',(4.64123187199515E-15,-1.82127309734388,
0.317064132275969));
#33052=CARTESIAN_POINT('Ctrl Pts',(-3.94730007868664E-15,-1.82205028923469,
0.304805345141405));
#33053=CARTESIAN_POINT('Ctrl Pts',(-3.88578058618805E-15,-1.82271089774678,
0.292550090914232));
#33054=CARTESIAN_POINT('Ctrl Pts',(-3.53663723185213E-15,-1.82646006833395,
0.222997492293347));
#33055=CARTESIAN_POINT('Ctrl Pts',(-9.71519400458447E-16,-1.82646676303548,
0.153449623029913));
#33056=CARTESIAN_POINT('Ctrl Pts',(-4.9960036108132E-16,-1.82271640812221,
0.0842505500111845));
#33057=CARTESIAN_POINT('Ctrl Pts',(-3.8896594232137E-17,-1.81905518131974,
0.0166960100539114));
#33058=CARTESIAN_POINT('Ctrl Pts',(-2.20143127797879E-15,-1.81181305450115,
-0.0505270526769876));
#33059=CARTESIAN_POINT('Ctrl Pts',(-3.63598040564739E-15,-1.80092992405888,
-0.117084349296312));
#33060=CARTESIAN_POINT('Ctrl Pts',(-4.59707087045625E-15,-1.79363866250945,
-0.161675072549023));
#33061=CARTESIAN_POINT('Ctrl Pts',(-7.24725434000752E-15,-1.78471220461912,
-0.205966658589872));
#33062=CARTESIAN_POINT('Ctrl Pts',(-7.79931674799172E-15,-1.7741212964033,
-0.249851830349142));
#33063=CARTESIAN_POINT('Ctrl Pts',(-8.24041846233515E-15,-1.76565908687249,
-0.284916388662309));
#33064=CARTESIAN_POINT('Ctrl Pts',(5.28590280211643E-16,-1.75613409737704,
-0.31972140139832));
#33065=CARTESIAN_POINT('Ctrl Pts',(6.66133814775094E-16,-1.74552739422258,
-0.354208724051798));
#33066=CARTESIAN_POINT('Ctrl Pts',(7.24534204826618E-16,-1.74102383392549,
-0.368851892130823));
#33067=CARTESIAN_POINT('Ctrl Pts',(-7.28293105322084E-16,-1.73632360239176,
-0.383442108934698));
#33068=CARTESIAN_POINT('Ctrl Pts',(-8.04911692853238E-16,-1.731434767294,
-0.397947207271473));
#33069=CARTESIAN_POINT('Ctrl Pts',(-1.13106292697556E-15,-1.7106238955208,
-0.459692742865968));
#33070=CARTESIAN_POINT('Ctrl Pts',(4.18317703168387E-15,-1.68637376486003,
-0.519987462298931));
#33071=CARTESIAN_POINT('Ctrl Pts',(3.1641356201817E-15,-1.65863595149533,
-0.578525678013812));
#33072=CARTESIAN_POINT('Ctrl Pts',(2.86946734591812E-15,-1.65061522387449,
-0.595452718277804));
#33073=CARTESIAN_POINT('Ctrl Pts',(5.57580897614692E-15,-1.64230259171472,
-0.612232718698034));
#33074=CARTESIAN_POINT('Ctrl Pts',(5.41233724504764E-15,-1.63369620203523,
-0.628857825595402));
#33075=CARTESIAN_POINT('Ctrl Pts',(4.79851125833417E-15,-1.6021508290194,
-0.68979455028902));
#33076=CARTESIAN_POINT('Ctrl Pts',(-3.78633153299722E-15,-1.56666180412204,
-0.748653919227771));
#33077=CARTESIAN_POINT('Ctrl Pts',(-3.78863607153335E-15,-1.52754044393195,
-0.805204911162976));
#33078=CARTESIAN_POINT('Ctrl Pts',(-3.79072214767112E-15,-1.49212765534529,
-0.856395061813092));
#33079=CARTESIAN_POINT('Ctrl Pts',(-2.05473902985757E-16,-1.45373734054848,
-0.90569356900811));
#33080=CARTESIAN_POINT('Ctrl Pts',(8.18789480661053E-16,-1.4125803735405,
-0.952892246296203));
#33081=CARTESIAN_POINT('Ctrl Pts',(1.01336693800835E-15,-1.40476185916187,
-0.961858493419257));
#33082=CARTESIAN_POINT('Ctrl Pts',(-1.57502819886435E-15,-1.39684930901895,
-0.970742099247602));
#33083=CARTESIAN_POINT('Ctrl Pts',(-1.51267887105178E-15,-1.38884786051959,
-0.97953835419035));
#33084=CARTESIAN_POINT('Ctrl Pts',(-1.1728207214089E-15,-1.34523299606383,
-1.0274856061257));
#33085=CARTESIAN_POINT('Ctrl Pts',(4.26408912821895E-15,-1.29894819098313,
-1.07287671206358));
#33086=CARTESIAN_POINT('Ctrl Pts',(3.09474668114262E-15,-1.25027379293301,
-1.11553472901405));
#33087=CARTESIAN_POINT('Ctrl Pts',(1.9305259728076E-15,-1.20181258952987,
-1.1580059031636));
#33088=CARTESIAN_POINT('Ctrl Pts',(-1.33080683399921E-15,-1.1509816522108,
-1.19776833545068));
#33089=CARTESIAN_POINT('Ctrl Pts',(-1.31145094783847E-15,-1.09803478904449,
-1.23460162248222));
#33090=CARTESIAN_POINT('Ctrl Pts',(-1.29249638855516E-15,-1.0461857314288,
-1.27067120446058));
#33091=CARTESIAN_POINT('Ctrl Pts',(5.22726634415042E-16,-0.992306651654647,
-1.3039321130855));
#33092=CARTESIAN_POINT('Ctrl Pts',(1.40165656858926E-15,-0.936628381019438,
-1.33412827396106));
#33093=CARTESIAN_POINT('Ctrl Pts',(1.55885413648105E-15,-0.92667026218884,
-1.33952888994277));
#33094=CARTESIAN_POINT('Ctrl Pts',(6.8101243531962E-15,-0.916654592115581,
-1.344831336662));
#33095=CARTESIAN_POINT('Ctrl Pts',(7.13318293321663E-15,-0.906582699777643,
-1.35003396913283));
#33096=CARTESIAN_POINT('Ctrl Pts',(7.43361135889431E-15,-0.897216340405636,
-1.35487215879643));
#33097=CARTESIAN_POINT('Ctrl Pts',(2.40141014764684E-15,-0.887809725328665,
-1.35961970024266));
#33098=CARTESIAN_POINT('Ctrl Pts',(2.23432383705813E-15,-0.878364903116739,
-1.36427535802199));
#33099=CARTESIAN_POINT('Ctrl Pts',(1.25007779416339E-15,-0.822728813869338,
-1.39170018253469));
#33100=CARTESIAN_POINT('Ctrl Pts',(7.66888170002638E-16,-0.765757994888109,
-1.41594579927101));
#33101=CARTESIAN_POINT('Ctrl Pts',(-7.97972798949331E-17,-0.707686469549987,
-1.43682247825627));
#33102=CARTESIAN_POINT('Ctrl Pts',(-9.11162927195913E-16,-0.650665681891094,
-1.4573214176678));
#33103=CARTESIAN_POINT('Ctrl Pts',(-2.79461917356239E-15,-0.59258279903694,
-1.47457243551005));
#33104=CARTESIAN_POINT('Ctrl Pts',(-3.42607886505419E-15,-0.533655823086145,
-1.48834629363144));
#33105=CARTESIAN_POINT('Ctrl Pts',(-4.03744356266809E-15,-0.476604085154388,
-1.50168182512904));
#33106=CARTESIAN_POINT('Ctrl Pts',(2.17949943466874E-15,-0.4187604494125,
-1.51175801196898));
#33107=CARTESIAN_POINT('Ctrl Pts',(2.21480819795339E-15,-0.360330467682485,
-1.5183183843601));
#33108=CARTESIAN_POINT('Ctrl Pts',(2.22298984612665E-15,-0.346791235242338,
-1.51983853555761));
#33109=CARTESIAN_POINT('Ctrl Pts',(-7.06947890110157E-17,-0.333220577381782,
-1.52116970064367));
#33110=CARTESIAN_POINT('Ctrl Pts',(-1.38777878078145E-17,-0.319621170202027,
-1.52230829911641));
#33111=CARTESIAN_POINT('Ctrl Pts',(-0.62186969212423,-1.9522756157026,0.00152956335005719));
#33112=CARTESIAN_POINT('Ctrl Pts',(-0.596980647355082,-1.94905199344704,
-0.435857502745632));
#33113=CARTESIAN_POINT('Ctrl Pts',(-0.572091602585934,-1.80373720486496,
-0.875183433556484));
#33114=CARTESIAN_POINT('Ctrl Pts',(-0.547202557816786,-1.53382353634896,
-1.21572541890428));
#33115=CARTESIAN_POINT('Ctrl Pts',(-0.510189384479222,-1.13242760124485,
-1.72215463904135));
#33116=CARTESIAN_POINT('Ctrl Pts',(-0.473176211141658,-0.455475380096762,
-2.01011851545296));
#33117=CARTESIAN_POINT('Ctrl Pts',(-0.436163037804093,0.1877843306312,-1.94813338333444));
#33118=CARTESIAN_POINT('Ctrl Pts',(-0.399149864466528,0.831044041359161,
-1.88614825121591));
#33119=CARTESIAN_POINT('Ctrl Pts',(-0.36213669112896,1.44061124166701,-1.47421411056724));
#33120=CARTESIAN_POINT('Ctrl Pts',(-0.325123517791396,1.73785158268385,
-0.900376109039905));
#33121=CARTESIAN_POINT('Ctrl Pts',(-0.288110344453831,2.0350919237007,-0.326538107512548));
#33122=CARTESIAN_POINT('Ctrl Pts',(-0.25109717111627,2.02000540542655,0.409203754893459));
#33123=CARTESIAN_POINT('Ctrl Pts',(-0.214083997778705,1.69970343852974,
0.970348270842328));
#33124=CARTESIAN_POINT('Ctrl Pts',(-0.177070824441142,1.37940147163295,
1.53149278679117));
#33125=CARTESIAN_POINT('Ctrl Pts',(-0.140057651103576,0.753884056113526,
1.91803995628285));
#33126=CARTESIAN_POINT('Ctrl Pts',(-0.103044477766013,0.108541537644872,
1.95400482961695));
#33127=CARTESIAN_POINT('Ctrl Pts',(-0.0686963185106752,-0.490335175692911,
1.98738016832708));
#33128=CARTESIAN_POINT('Ctrl Pts',(-0.0343481592553384,-1.10628488527308,
1.7188407961645));
#33129=CARTESIAN_POINT('Ctrl Pts',(-1.90819582357449E-15,-1.495768828606,
1.26227079838508));
#33130=CARTESIAN_POINT('',(-19.646,-0.903606778650192,-1.26612599672285));
#33131=CARTESIAN_POINT('Ctrl Pts',(-19.646,-0.905542040608585,-1.26787934382136));
#33132=CARTESIAN_POINT('Ctrl Pts',(-19.646,-0.938681876239101,-1.25016622609516));
#33133=CARTESIAN_POINT('Ctrl Pts',(-19.646,-0.971073440107613,-1.23120562508964));
#33134=CARTESIAN_POINT('Ctrl Pts',(-19.646,-1.00263785675273,-1.21101354619544));
#33135=CARTESIAN_POINT('Ctrl Pts',(-19.646,-1.05261277003695,-1.17904408504205));
#33136=CARTESIAN_POINT('Ctrl Pts',(-19.646,-1.1005155382739,-1.14399043040363));
#33137=CARTESIAN_POINT('Ctrl Pts',(-19.646,-1.14626793887678,-1.10617282136889));
#33138=CARTESIAN_POINT('Ctrl Pts',(-19.646,-1.17314439188448,-1.08395752383931));
#33139=CARTESIAN_POINT('Ctrl Pts',(-19.646,-1.19927853253817,-1.06078746270321));
#33140=CARTESIAN_POINT('Ctrl Pts',(-19.646,-1.22465143234114,-1.03672005685037));
#33141=CARTESIAN_POINT('Ctrl Pts',(-19.646,-1.23635098556182,-1.02562247250465));
#33142=CARTESIAN_POINT('Ctrl Pts',(-19.646,-1.24789041542034,-1.01433201252715));
#33143=CARTESIAN_POINT('Ctrl Pts',(-19.646,-1.25925110031853,-1.00287136143659));
#33144=CARTESIAN_POINT('Ctrl Pts',(-19.646,-1.30312281878128,-0.958613602106813));
#33145=CARTESIAN_POINT('Ctrl Pts',(-19.646,-1.3443847292608,-0.911772278773441));
#33146=CARTESIAN_POINT('Ctrl Pts',(-19.646,-1.38294904546205,-0.862696554410881));
#33147=CARTESIAN_POINT('Ctrl Pts',(-19.646,-1.41264445582053,-0.824907118031911));
#33148=CARTESIAN_POINT('Ctrl Pts',(-19.646,-1.44074010106896,-0.785791596811784));
#33149=CARTESIAN_POINT('Ctrl Pts',(-19.646,-1.4671857543939,-0.745491044869591));
#33150=CARTESIAN_POINT('Ctrl Pts',(-19.646,-1.47620661389258,-0.731744149970738));
#33151=CARTESIAN_POINT('Ctrl Pts',(-19.646,-1.48503539940812,-0.717859249822184));
#33152=CARTESIAN_POINT('Ctrl Pts',(-19.646,-1.49366982591613,-0.703841592408462));
#33153=CARTESIAN_POINT('Ctrl Pts',(-19.646,-1.50209114300791,-0.69016990988787));
#33154=CARTESIAN_POINT('Ctrl Pts',(-19.646,-1.51032951371256,-0.676368303403145));
#33155=CARTESIAN_POINT('Ctrl Pts',(-19.646,-1.51836903542545,-0.662465935470385));
#33156=CARTESIAN_POINT('Ctrl Pts',(-19.646,-1.55076424157064,-0.606446424463152));
#33157=CARTESIAN_POINT('Ctrl Pts',(-19.646,-1.57997764506433,-0.548725277846029));
#33158=CARTESIAN_POINT('Ctrl Pts',(-19.646,-1.6059180737153,-0.489656925507297));
#33159=CARTESIAN_POINT('Ctrl Pts',(-19.646,-1.63239976292013,-0.429356081233618));
#33160=CARTESIAN_POINT('Ctrl Pts',(-19.646,-1.65547122307238,-0.367650443296635));
#33161=CARTESIAN_POINT('Ctrl Pts',(-19.646,-1.67500154178622,-0.304875460933321));
#33162=CARTESIAN_POINT('Ctrl Pts',(-19.646,-1.68790625616863,-0.263396710400418));
#33163=CARTESIAN_POINT('Ctrl Pts',(-19.646,-1.69926421211363,-0.221450247756649));
#33164=CARTESIAN_POINT('Ctrl Pts',(-19.646,-1.70902729549459,-0.17912585728895));
#33165=CARTESIAN_POINT('Ctrl Pts',(-19.646,-1.71381101181734,-0.158387749292715));
#33166=CARTESIAN_POINT('Ctrl Pts',(-19.646,-1.7182116941742,-0.137558839576148));
#33167=CARTESIAN_POINT('Ctrl Pts',(-19.646,-1.72222284706313,-0.116649366767487));
#33168=CARTESIAN_POINT('Ctrl Pts',(-19.646,-1.72468902535469,-0.103793589549136));
#33169=CARTESIAN_POINT('Ctrl Pts',(-19.646,-1.72700794401817,-0.0909073545491223));
#33170=CARTESIAN_POINT('Ctrl Pts',(-19.646,-1.72917798177892,-0.0779930136645168));
#33171=CARTESIAN_POINT('Ctrl Pts',(-19.646,-1.73099216263167,-0.0671964504052968));
#33172=CARTESIAN_POINT('Ctrl Pts',(-19.646,-1.73270181297803,-0.0563826288020671));
#33173=CARTESIAN_POINT('Ctrl Pts',(-19.646,-1.73430467550777,-0.0455638649458739));
#33174=CARTESIAN_POINT('Ctrl Pts',(-19.646,-1.74423506188351,0.0214627846927948));
#33175=CARTESIAN_POINT('Ctrl Pts',(-19.646,-1.75008999734432,0.0887933599084955));
#33176=CARTESIAN_POINT('Ctrl Pts',(-19.646,-1.75174634352653,0.156072973815415));
#33177=CARTESIAN_POINT('Ctrl Pts',(-19.646,-1.75216732819483,0.173173074173518));
#33178=CARTESIAN_POINT('Ctrl Pts',(-19.646,-1.75231686986298,0.190270032654354));
#33179=CARTESIAN_POINT('Ctrl Pts',(-19.646,-1.75219248471346,0.207358295798386));
#33180=CARTESIAN_POINT('Ctrl Pts',(-19.646,-1.75172041634255,0.272211926443289));
#33181=CARTESIAN_POINT('Ctrl Pts',(-19.646,-1.74730691088489,0.336939554811864));
#33182=CARTESIAN_POINT('Ctrl Pts',(-19.646,-1.73916871539667,0.401305845369932));
#33183=CARTESIAN_POINT('Ctrl Pts',(-19.646,-1.73475683721818,0.436200095963245));
#33184=CARTESIAN_POINT('Ctrl Pts',(-19.646,-1.72924938721083,0.470988342069356));
#33185=CARTESIAN_POINT('Ctrl Pts',(-19.646,-1.7226747045139,0.505633709783685));
#33186=CARTESIAN_POINT('Ctrl Pts',(-19.646,-1.7177037781737,0.531828064534477));
#33187=CARTESIAN_POINT('Ctrl Pts',(-19.646,-1.71212268625163,0.557940753879483));
#33188=CARTESIAN_POINT('Ctrl Pts',(-19.646,-1.70594210832947,0.58395576292157));
#33189=CARTESIAN_POINT('Ctrl Pts',(-19.646,-1.70239611990861,0.598881376997373));
#33190=CARTESIAN_POINT('Ctrl Pts',(-19.646,-1.69865150339267,0.613779102795182));
#33191=CARTESIAN_POINT('Ctrl Pts',(-19.646,-1.69471797730657,0.628617701099107));
#33192=CARTESIAN_POINT('Ctrl Pts',(-19.646,-1.67733891462321,0.694177436667802));
#33193=CARTESIAN_POINT('Ctrl Pts',(-19.646,-1.65625524843458,0.758681559480687));
#33194=CARTESIAN_POINT('Ctrl Pts',(-19.646,-1.63172440972949,0.821874451021119));
#33195=CARTESIAN_POINT('Ctrl Pts',(-19.646,-1.60667765966343,0.886396360744345));
#33196=CARTESIAN_POINT('Ctrl Pts',(-19.646,-1.57803704609287,0.949552185162904));
#33197=CARTESIAN_POINT('Ctrl Pts',(-19.646,-1.54602141156002,1.01107293048721));
#33198=CARTESIAN_POINT('Ctrl Pts',(-19.646,-1.51376408399581,1.07305810938115));
#33199=CARTESIAN_POINT('Ctrl Pts',(-19.646,-1.47808026191821,1.13338441161316));
#33200=CARTESIAN_POINT('Ctrl Pts',(-19.646,-1.43914228877744,1.19176565197817));
#33201=CARTESIAN_POINT('Ctrl Pts',(-19.646,-1.42928345262248,1.206547394243));
#33202=CARTESIAN_POINT('Ctrl Pts',(-19.646,-1.41921576123314,1.22120434749156));
#33203=CARTESIAN_POINT('Ctrl Pts',(-19.646,-1.40894153299102,1.23573163636577));
#33204=CARTESIAN_POINT('Ctrl Pts',(-19.646,-1.4015641455592,1.2461629248123));
#33205=CARTESIAN_POINT('Ctrl Pts',(-19.646,-1.39407933992703,1.25652845558403));
#33206=CARTESIAN_POINT('Ctrl Pts',(-19.646,-1.38649911575537,1.26681166279554));
#33207=CARTESIAN_POINT('Ctrl Pts',(-19.646,-1.34366530428306,1.32491930566387));
#33208=CARTESIAN_POINT('Ctrl Pts',(-19.646,-1.2977140106402,1.38050707160548));
#33209=CARTESIAN_POINT('Ctrl Pts',(-19.646,-1.2488866714459,1.4332945374332));
#33210=CARTESIAN_POINT('Ctrl Pts',(-19.646,-1.19994324988706,1.48620750045065));
#33211=CARTESIAN_POINT('Ctrl Pts',(-19.646,-1.14810965971326,1.53630784170276));
#33212=CARTESIAN_POINT('Ctrl Pts',(-19.646,-1.09357943713849,1.58329695308289));
#33213=CARTESIAN_POINT('Ctrl Pts',(-19.646,-1.04021055626029,1.62928532740834));
#33214=CARTESIAN_POINT('Ctrl Pts',(-19.646,-0.984258111839382,1.67229443841277));
#33215=CARTESIAN_POINT('Ctrl Pts',(-19.646,-0.925863744774077,1.71201523240195));
#33216=CARTESIAN_POINT('Ctrl Pts',(-19.646,-0.90473592603761,1.72638671680443));
#33217=CARTESIAN_POINT('Ctrl Pts',(-19.646,-0.883288096751299,1.74032739005835));
#33218=CARTESIAN_POINT('Ctrl Pts',(-19.646,-0.861525859670609,1.7538213116275));
#33219=CARTESIAN_POINT('Ctrl Pts',(-19.646,-0.90554204060855,-1.26787934382138));
#33220=CARTESIAN_POINT('Ctrl Pts',(-19.6116518407447,-0.515303398567461,
-1.54346439101212));
#33221=CARTESIAN_POINT('Ctrl Pts',(-19.5402905081518,0.58155483362262,-1.722138088561));
#33222=CARTESIAN_POINT('Ctrl Pts',(-19.4319160022213,1.77174315090552,-0.488859491694061));
#33223=CARTESIAN_POINT('Ctrl Pts',(-19.3208764822086,1.37253690144282,1.22265204623408));
#33224=CARTESIAN_POINT('Ctrl Pts',(-19.2098369621959,-0.281145520007231,
1.81625519837393));
#33225=CARTESIAN_POINT('Ctrl Pts',(-19.1201927262585,-1.40868791973966,
0.955800011746829));
#33226=CARTESIAN_POINT('Ctrl Pts',(-19.0675616636586,-1.554016444368,0.219461333177004));
#33227=CARTESIAN_POINT('Ctrl Pts',(-19.0519437743963,-1.55320700821059,
0.000650635102509029));
#33228=CARTESIAN_POINT('Origin',(-19.646,-2.59090492670967E-16,0.));
#33229=CARTESIAN_POINT('',(-19.646,-1.954,-2.39295984553393E-16));
#33230=CARTESIAN_POINT('Origin',(-19.646,0.,0.));
#33231=CARTESIAN_POINT('Origin',(-19.646,0.,0.));
#33232=CARTESIAN_POINT('',(-19.646,0.903606778650242,-1.26612599672281));
#33233=CARTESIAN_POINT('Ctrl Pts',(-19.646,0.863566768236388,1.75638951800437));
#33234=CARTESIAN_POINT('Ctrl Pts',(-19.646,0.903322736553012,1.7319792089365));
#33235=CARTESIAN_POINT('Ctrl Pts',(-19.646,0.942081600816466,1.706082519315));
#33236=CARTESIAN_POINT('Ctrl Pts',(-19.646,0.979747741712395,1.67869459433238));
#33237=CARTESIAN_POINT('Ctrl Pts',(-19.646,1.0378592801315,1.63644034643253));
#33238=CARTESIAN_POINT('Ctrl Pts',(-19.646,1.09337204689005,1.59063767529025));
#33239=CARTESIAN_POINT('Ctrl Pts',(-19.646,1.14612449678451,1.5416273763348));
#33240=CARTESIAN_POINT('Ctrl Pts',(-19.646,1.17160987932026,1.51794987472928));
#33241=CARTESIAN_POINT('Ctrl Pts',(-19.646,1.19645037254775,1.49352326161613));
#33242=CARTESIAN_POINT('Ctrl Pts',(-19.646,1.22062397437646,1.46838397290312));
#33243=CARTESIAN_POINT('Ctrl Pts',(-19.646,1.23081678670849,1.45778397817217));
#33244=CARTESIAN_POINT('Ctrl Pts',(-19.646,1.24089100137359,1.44705726575374));
#33245=CARTESIAN_POINT('Ctrl Pts',(-19.646,1.25084482785001,1.43620652381068));
#33246=CARTESIAN_POINT('Ctrl Pts',(-19.646,1.26039541734236,1.42579535357066));
#33247=CARTESIAN_POINT('Ctrl Pts',(-19.646,1.2698316591578,1.41527374749551));
#33248=CARTESIAN_POINT('Ctrl Pts',(-19.646,1.27914724914785,1.40465014664234));
#33249=CARTESIAN_POINT('Ctrl Pts',(-19.646,1.32621262813245,1.35097627296714));
#33250=CARTESIAN_POINT('Ctrl Pts',(-19.646,1.37024304194926,1.29465625509195));
#33251=CARTESIAN_POINT('Ctrl Pts',(-19.646,1.41107688405619,1.23602526535197));
#33252=CARTESIAN_POINT('Ctrl Pts',(-19.646,1.44042814800574,1.19388145603382));
#33253=CARTESIAN_POINT('Ctrl Pts',(-19.646,1.46812692994879,1.15054294882141));
#33254=CARTESIAN_POINT('Ctrl Pts',(-19.646,1.49409735999621,1.10612915663656));
#33255=CARTESIAN_POINT('Ctrl Pts',(-19.646,1.50834342473973,1.08176599600291));
#33256=CARTESIAN_POINT('Ctrl Pts',(-19.646,1.52206917616524,1.05707922579962));
#33257=CARTESIAN_POINT('Ctrl Pts',(-19.646,1.53526026066111,1.03208840623726));
#33258=CARTESIAN_POINT('Ctrl Pts',(-19.646,1.54099272219805,1.0212281231451));
#33259=CARTESIAN_POINT('Ctrl Pts',(-19.646,1.54662359108262,1.01031139276512));
#33260=CARTESIAN_POINT('Ctrl Pts',(-19.646,1.55214625633791,0.999351117833026));
#33261=CARTESIAN_POINT('Ctrl Pts',(-19.646,1.58348920551541,0.937147937975382));
#33262=CARTESIAN_POINT('Ctrl Pts',(-19.646,1.61140228754486,0.873447373552883));
#33263=CARTESIAN_POINT('Ctrl Pts',(-19.646,1.63573409282643,0.808558728131928));
#33264=CARTESIAN_POINT('Ctrl Pts',(-19.646,1.65948765101661,0.745212166006688));
#33265=CARTESIAN_POINT('Ctrl Pts',(-19.646,1.67982822719404,0.680732341235376));
#33266=CARTESIAN_POINT('Ctrl Pts',(-19.646,1.69656663148463,0.615401331854704));
#33267=CARTESIAN_POINT('Ctrl Pts',(-19.646,1.70778068689243,0.571632191958015));
#33268=CARTESIAN_POINT('Ctrl Pts',(-19.646,1.71737693174782,0.527480906477519));
#33269=CARTESIAN_POINT('Ctrl Pts',(-19.646,1.72528552443309,0.483033998311475));
#33270=CARTESIAN_POINT('Ctrl Pts',(-19.646,1.7316045497537,0.447520582802376));
#33271=CARTESIAN_POINT('Ctrl Pts',(-19.646,1.73684596146418,0.411818446376242));
#33272=CARTESIAN_POINT('Ctrl Pts',(-19.646,1.74096908581929,0.375973249752788));
#33273=CARTESIAN_POINT('Ctrl Pts',(-19.646,1.74271973989503,0.360753592483218));
#33274=CARTESIAN_POINT('Ctrl Pts',(-19.646,1.74426900447266,0.345503519836166));
#33275=CARTESIAN_POINT('Ctrl Pts',(-19.646,1.74561136180707,0.330255732772084));
#33276=CARTESIAN_POINT('Ctrl Pts',(-19.646,1.75132555048616,0.265348475971802));
#33277=CARTESIAN_POINT('Ctrl Pts',(-19.646,1.75330734745255,0.200390062729164));
#33278=CARTESIAN_POINT('Ctrl Pts',(-19.646,1.75138973772329,0.135641060055424));
#33279=CARTESIAN_POINT('Ctrl Pts',(-19.646,1.75083523799717,0.116918113617963));
#33280=CARTESIAN_POINT('Ctrl Pts',(-19.646,1.74995436364999,0.0982127193910304));
#33281=CARTESIAN_POINT('Ctrl Pts',(-19.646,1.74874226605705,0.079531327482009));
#33282=CARTESIAN_POINT('Ctrl Pts',(-19.646,1.74429950877487,0.0110575590098168));
#33283=CARTESIAN_POINT('Ctrl Pts',(-19.646,1.73541095028425,-0.0570958748323909));
#33284=CARTESIAN_POINT('Ctrl Pts',(-19.646,1.72226904404541,-0.124592446033735));
#33285=CARTESIAN_POINT('Ctrl Pts',(-19.646,1.71037294405752,-0.185690580905332));
#33286=CARTESIAN_POINT('Ctrl Pts',(-19.646,1.69499049540238,-0.246250814205604));
#33287=CARTESIAN_POINT('Ctrl Pts',(-19.646,1.6762313128498,-0.305997837855447));
#33288=CARTESIAN_POINT('Ctrl Pts',(-19.646,1.67266766774541,-0.317347862715789));
#33289=CARTESIAN_POINT('Ctrl Pts',(-19.646,1.66898472870697,-0.328659924368977));
#33290=CARTESIAN_POINT('Ctrl Pts',(-19.646,1.66518531160415,-0.339927647595734));
#33291=CARTESIAN_POINT('Ctrl Pts',(-19.646,1.64447516439434,-0.401346596984588));
#33292=CARTESIAN_POINT('Ctrl Pts',(-19.646,1.62029376539845,-0.46149556132515));
#33293=CARTESIAN_POINT('Ctrl Pts',(-19.646,1.59282690139432,-0.520099973095403));
#33294=CARTESIAN_POINT('Ctrl Pts',(-19.646,1.56548034847439,-0.578447684271151));
#33295=CARTESIAN_POINT('Ctrl Pts',(-19.646,1.53487629167091,-0.635265175881805));
#33296=CARTESIAN_POINT('Ctrl Pts',(-19.646,1.50115876935599,-0.690248721836702));
#33297=CARTESIAN_POINT('Ctrl Pts',(-19.646,1.46814035521906,-0.744092224158713));
#33298=CARTESIAN_POINT('Ctrl Pts',(-19.646,1.43213550204336,-0.796177659254549));
#33299=CARTESIAN_POINT('Ctrl Pts',(-19.646,1.39325288886873,-0.846177847660815));
#33300=CARTESIAN_POINT('Ctrl Pts',(-19.646,1.38629874007184,-0.855120372909513));
#33301=CARTESIAN_POINT('Ctrl Pts',(-19.646,1.37925248612795,-0.863996072867638));
#33302=CARTESIAN_POINT('Ctrl Pts',(-19.646,1.37211468424398,-0.872802907558143));
#33303=CARTESIAN_POINT('Ctrl Pts',(-19.646,1.3654767793905,-0.880992954254046));
#33304=CARTESIAN_POINT('Ctrl Pts',(-19.646,1.35876562654603,-0.88911612283082));
#33305=CARTESIAN_POINT('Ctrl Pts',(-19.646,1.35198260679088,-0.897170459130779));
#33306=CARTESIAN_POINT('Ctrl Pts',(-19.646,1.31202659151418,-0.944615283981971));
#33307=CARTESIAN_POINT('Ctrl Pts',(-19.646,1.26957231590532,-0.989683649287115));
#33308=CARTESIAN_POINT('Ctrl Pts',(-19.646,1.2247580044259,-1.03210786368823));
#33309=CARTESIAN_POINT('Ctrl Pts',(-19.646,1.18075456163743,-1.07376445573702));
#33310=CARTESIAN_POINT('Ctrl Pts',(-19.646,1.13447500920147,-1.1128722506342));
#33311=CARTESIAN_POINT('Ctrl Pts',(-19.646,1.08602704351211,-1.14913379788722));
#33312=CARTESIAN_POINT('Ctrl Pts',(-19.646,1.03912084562306,-1.18424138779347));
#33313=CARTESIAN_POINT('Ctrl Pts',(-19.646,0.990181444901801,-1.21668129711651));
#33314=CARTESIAN_POINT('Ctrl Pts',(-19.646,0.939294206718905,-1.24613612817705));
#33315=CARTESIAN_POINT('Ctrl Pts',(-19.646,0.927502678262808,-1.25296136552578));
#33316=CARTESIAN_POINT('Ctrl Pts',(-19.646,0.915606530740291,-1.25962610621517));
#33317=CARTESIAN_POINT('Ctrl Pts',(-19.646,0.903606778650211,-1.26612599672283));
#33318=CARTESIAN_POINT('Origin',(-19.646,0.,0.));
#33319=CARTESIAN_POINT('Origin',(-20.9400562256037,0.,0.));
#33320=CARTESIAN_POINT('Ctrl Pts',(-19.646,0.903606778650211,-1.26612599672283));
#33321=CARTESIAN_POINT('Ctrl Pts',(-19.6089868266624,1.32425114367218,-0.965921198291487));
#33322=CARTESIAN_POINT('Ctrl Pts',(-19.5349604799873,1.83563729847737,0.081414173630813));
#33323=CARTESIAN_POINT('Ctrl Pts',(-19.4239209599746,0.926784913186551,
1.58861167214729));
#33324=CARTESIAN_POINT('Ctrl Pts',(-19.3128814399619,-0.829751980945401,
1.63941117334604));
#33325=CARTESIAN_POINT('Ctrl Pts',(-19.234926528505,-1.53031391152993,0.624960285503497));
#33326=CARTESIAN_POINT('Ctrl Pts',(-19.1939847903856,-1.55770722541468,
0.0556933182705827));
#33327=CARTESIAN_POINT('Ctrl Pts',(-19.1900562256037,-1.55732260026824,
0.00102952447757978));
#33328=CARTESIAN_POINT('Ctrl Pts',(-19.8760740822721,1.13509973994379,-1.59049193030947));
#33329=CARTESIAN_POINT('Ctrl Pts',(-19.8390609089345,1.66350802618803,-1.21337834873771));
#33330=CARTESIAN_POINT('Ctrl Pts',(-19.7650345622594,2.30590503453859,0.102271485229633));
#33331=CARTESIAN_POINT('Ctrl Pts',(-19.6539950422467,1.16421582794371,1.9955944759729));
#33332=CARTESIAN_POINT('Ctrl Pts',(-19.542955522234,-1.04232424993082,2.05940818561114));
#33333=CARTESIAN_POINT('Ctrl Pts',(-19.4319160022213,-2.29585551567116,
0.244228327910747));
#33334=CARTESIAN_POINT('Ctrl Pts',(-19.3208764822086,-1.45163427674195,
-1.79566928904087));
#33335=CARTESIAN_POINT('Ctrl Pts',(-19.2098369621959,0.719270307589218,
-2.19382897651929));
#33336=CARTESIAN_POINT('Ctrl Pts',(-19.0987974421832,2.23281233943022,-0.587628905444012));
#33337=CARTESIAN_POINT('Ctrl Pts',(-18.9877579221705,1.70598616341913,1.55578514652744));
#33338=CARTESIAN_POINT('Ctrl Pts',(-18.8767184021578,-0.379838299429391,
2.27736225800791));
#33339=CARTESIAN_POINT('Ctrl Pts',(-18.7656788821451,-2.11854523576817,
0.917883122180374));
#33340=CARTESIAN_POINT('Ctrl Pts',(-18.6546393621324,-1.92127159556107,
-1.28041564965079));
#33341=CARTESIAN_POINT('Ctrl Pts',(-18.5435998421198,0.03171693881648,-2.30861767801051));
#33342=CARTESIAN_POINT('Ctrl Pts',(-18.432560322107,1.95572010220925,-1.22714892034321));
#33343=CARTESIAN_POINT('Ctrl Pts',(-18.3215208020944,2.09253210076758,0.975727678888284));
#33344=CARTESIAN_POINT('Ctrl Pts',(-18.2104812820816,0.317129050815823,
2.28695445182457));
#33345=CARTESIAN_POINT('Ctrl Pts',(-18.099441762069,-1.74807521169763,1.50829928845439));
#33346=CARTESIAN_POINT('Ctrl Pts',(-17.9884022420563,-2.21583935163955,
-0.648682819590979));
#33347=CARTESIAN_POINT('Ctrl Pts',(-17.8773627220436,-0.658707176843674,
-2.21287998534429));
#33348=CARTESIAN_POINT('Ctrl Pts',(-17.7663232020309,1.50037008987612,-1.75488543793783));
#33349=CARTESIAN_POINT('Ctrl Pts',(-17.6552836820182,2.28836703304007,0.306772824349375));
#33350=CARTESIAN_POINT('Ctrl Pts',(-17.5442441620055,0.985189881382429,
2.08809340919601));
#33351=CARTESIAN_POINT('Ctrl Pts',(-17.4332046419928,-1.21828145781376,
1.96125559954424));
#33352=CARTESIAN_POINT('Ctrl Pts',(-17.3221651219801,-2.30845297604624,
0.0421673077566786));
#33353=CARTESIAN_POINT('Ctrl Pts',(-17.2111256019674,-1.28909530809731,
-1.91545464701142));
#33354=CARTESIAN_POINT('Ctrl Pts',(-17.1000860819548,0.908273868493995,
-2.12268033511088));
#33355=CARTESIAN_POINT('Ctrl Pts',(-16.989046561942,2.27563686670409,-0.390141094771527));
#33356=CARTESIAN_POINT('Ctrl Pts',(-16.8780070419294,1.56345896252262,1.69892003778701));
#33357=CARTESIAN_POINT('Ctrl Pts',(-16.7669675219166,-0.577451666473502,
2.23546030968653));
#33358=CARTESIAN_POINT('Ctrl Pts',(-16.655928001904,-2.19067073934843,0.729174145634008));
#33359=CARTESIAN_POINT('Ctrl Pts',(-16.5448884818913,-1.80199334427159,
-1.44345183849261));
#33360=CARTESIAN_POINT('Ctrl Pts',(-16.4338489618786,0.233396195306619,
-2.29701097929521));
#33361=CARTESIAN_POINT('Ctrl Pts',(-16.3228094418659,2.05550173441762,-1.05149695326574));
#33362=CARTESIAN_POINT('Ctrl Pts',(-16.2117699218532,1.99923203984308,1.15490453016024));
#33363=CARTESIAN_POINT('Ctrl Pts',(-16.1007304018405,0.116007939373285,
2.30592180720441));
#33364=CARTESIAN_POINT('Ctrl Pts',(-15.9896908818278,-1.8732274753089,1.34972295256322));
#33365=CARTESIAN_POINT('Ctrl Pts',(-15.8786513618151,-2.150654995229,-0.839890656231781));
#33366=CARTESIAN_POINT('Ctrl Pts',(-15.7676118418024,-0.462753558433016,
-2.26198858686089));
#33367=CARTESIAN_POINT('Ctrl Pts',(-15.6565723217897,1.6480250809965,-1.61701779685203));
#33368=CARTESIAN_POINT('Ctrl Pts',(-15.545532801777,2.25279210058805,0.505629285601668));
#33369=CARTESIAN_POINT('Ctrl Pts',(-15.4344932817643,0.798894407071541,
2.16621812135345));
#33370=CARTESIAN_POINT('Ctrl Pts',(-15.3234537617516,-1.38505544035138,
1.84725597849434));
#33371=CARTESIAN_POINT('Ctrl Pts',(-15.212414241739,-2.30330271361953,-0.159780575674832));
#33372=CARTESIAN_POINT('Ctrl Pts',(-15.1013747217263,-1.11672725650928,
-2.02080515079989));
#33373=CARTESIAN_POINT('Ctrl Pts',(-14.9903352017136,1.09034494175236,-2.03516120514448));
#33374=CARTESIAN_POINT('Ctrl Pts',(-14.8792956817009,2.30102929929156,-0.189729772919033));
#33375=CARTESIAN_POINT('Ctrl Pts',(-14.7682561616882,1.40896843633621,1.82908205620699));
#33376=CARTESIAN_POINT('Ctrl Pts',(-14.6572166416755,-0.770647368334038,
2.17642731480055));
#33377=CARTESIAN_POINT('Ctrl Pts',(-14.5461771216628,-2.24602395668922,
0.534892146986835));
#33378=CARTESIAN_POINT('Ctrl Pts',(-14.4351376016501,-1.66892075198025,
-1.59544249239507));
#33379=CARTESIAN_POINT('Ctrl Pts',(-14.3240980816374,0.433289123769849,
-2.26781695869681));
#33380=CARTESIAN_POINT('Ctrl Pts',(-14.2130585616247,2.13954722507716,-0.867796574431303));
#33381=CARTESIAN_POINT('Ctrl Pts',(-14.102019041612,1.89062696210268,1.32524070006188));
#33382=CARTESIAN_POINT('Ctrl Pts',(-13.9909795215993,-0.0860013354994131,
2.30723579055597));
#33383=CARTESIAN_POINT('Ctrl Pts',(-13.8799400015866,-1.98403919653764,
1.18081399446837));
#33384=CARTESIAN_POINT('Ctrl Pts',(-13.768900481574,-2.0690062987299,-1.02466880441734));
#33385=CARTESIAN_POINT('Ctrl Pts',(-13.6578609615612,-0.263257316964935,
-2.29378046203086));
#33386=CARTESIAN_POINT('Ctrl Pts',(-13.5468214415486,1.78306359718642,-1.46677109029281));
#33387=CARTESIAN_POINT('Ctrl Pts',(-13.4357819215358,2.19997090153458,0.700614912295794));
#33388=CARTESIAN_POINT('Ctrl Pts',(-13.3247424015232,0.606482988467133,
2.22775932444016));
#33389=CARTESIAN_POINT('Ctrl Pts',(-13.2137028815105,-1.5412261184387,1.71911467760951));
#33390=CARTESIAN_POINT('Ctrl Pts',(-13.1026633614978,-2.28051949798023,
-0.360505259687157));
#33391=CARTESIAN_POINT('Ctrl Pts',(-12.9916238414851,-0.935810089682886,
-2.11068536238299));
#33392=CARTESIAN_POINT('Ctrl Pts',(-12.8805843214724,1.26406886990054,-1.93206188179325));
#33393=CARTESIAN_POINT('Ctrl Pts',(-12.7695448014597,2.30880618249247,0.0121340271403076));
#33394=CARTESIAN_POINT('Ctrl Pts',(-12.658505281447,1.24369154023141,1.94524152117081));
#33395=CARTESIAN_POINT('Ctrl Pts',(-12.5474657614343,-0.95794337267385,
2.10073266211585));
#33396=CARTESIAN_POINT('Ctrl Pts',(-12.4364262414216,-2.28418271846725,
0.336515276897891));
#33397=CARTESIAN_POINT('Ctrl Pts',(-12.3253867214089,-1.52307172262353,
-1.73521922265594));
#33398=CARTESIAN_POINT('Ctrl Pts',(-12.2143472013963,0.629865003645723,
-2.22126164602743));
#33399=CARTESIAN_POINT('Ctrl Pts',(-12.1033076813835,2.20721339369492,-0.677452771507981));
#33400=CARTESIAN_POINT('Ctrl Pts',(-11.9922681613709,1.76754817351653,1.48543147846963));
#33401=CARTESIAN_POINT('Ctrl Pts',(-11.8812286413582,-0.287352226413828,
2.29088671062214));
#33402=CARTESIAN_POINT('Ctrl Pts',(-11.7701891213455,-2.07966208876338,
1.00286530475953));
#33403=CARTESIAN_POINT('Ctrl Pts',(-11.6591496013328,-1.97151830685153,
-1.2016025918245));
#33404=CARTESIAN_POINT('Ctrl Pts',(-11.5481100813201,-0.0617457068599174,
-2.30801228129628));
#33405=CARTESIAN_POINT('Ctrl Pts',(-11.4370705613074,1.90445185478939,-1.30529550513259));
#33406=CARTESIAN_POINT('Ctrl Pts',(-11.3260310412947,2.13030780646733,0.890236975548903));
#33407=CARTESIAN_POINT('Ctrl Pts',(-11.214991521282,0.409428634168118,2.2722458970044));
#33408=CARTESIAN_POINT('Ctrl Pts',(-11.1039520012693,-1.68559792682173,
1.57781267963734));
#33409=CARTESIAN_POINT('Ctrl Pts',(-10.9929124812566,-2.24027774585957,
-0.558470092606996));
#33410=CARTESIAN_POINT('Ctrl Pts',(-10.8818729612439,-0.74772882072763,
-2.18440720415937));
#33411=CARTESIAN_POINT('Ctrl Pts',(-10.7708334412313,1.42811570802619,-1.81417164221552));
#33412=CARTESIAN_POINT('Ctrl Pts',(-10.6597939212185,2.29890798025732,0.213904935051304));
#33413=CARTESIAN_POINT('Ctrl Pts',(-10.5487544012059,1.06889355292529,2.04650917306638));
#33414=CARTESIAN_POINT('Ctrl Pts',(-10.4377148811932,-1.13790583334797,
2.00895583260627));
#33415=CARTESIAN_POINT('Ctrl Pts',(-10.3266753611805,-2.30485489994822,
0.135562211234455));
#33416=CARTESIAN_POINT('Ctrl Pts',(-10.2156358411678,-1.36556280469463,
-1.86171196734742));
#33417=CARTESIAN_POINT('Ctrl Pts',(-10.1045963211551,0.821618946610189,
-2.15770144586809));
#33418=CARTESIAN_POINT('Ctrl Pts',(-9.99355680114238,2.25798222133836,-0.481922723110236));
#33419=CARTESIAN_POINT('Ctrl Pts',(-9.88251728112969,1.63093790480174,1.6342505235156));
#33420=CARTESIAN_POINT('Ctrl Pts',(-9.77147776111699,-0.48650328990636,
2.25699972792208));
#33421=CARTESIAN_POINT('Ctrl Pts',(-9.6604382411043,-2.15936411011838,0.817239171150482));
#33422=CARTESIAN_POINT('Ctrl Pts',(-9.5493987210916,-1.85893733974787,-1.36933750033409));
#33423=CARTESIAN_POINT('Ctrl Pts',(-9.43835920107892,0.140238598030964,
-2.30457509284302));
#33424=CARTESIAN_POINT('Ctrl Pts',(-9.32731968106622,2.01126056496325,-1.13382721909196));
#33425=CARTESIAN_POINT('Ctrl Pts',(-9.21628016105352,2.04433612180518,1.0730438220374));
#33426=CARTESIAN_POINT('Ctrl Pts',(-9.10524064104083,0.209239895465708,
2.29933727171017));
#33427=CARTESIAN_POINT('Ctrl Pts',(-8.99420112102815,-1.81706562588916,
1.42443172322934));
#33428=CARTESIAN_POINT('Ctrl Pts',(-8.88316160101544,-2.18288552833439,
-0.752159552966248));
#33429=CARTESIAN_POINT('Ctrl Pts',(-8.77212208100277,-0.553923307403332,
-2.24140629794008));
#33430=CARTESIAN_POINT('Ctrl Pts',(-8.66108256099004,1.58122959415986,-1.6823929961466));
#33431=CARTESIAN_POINT('Ctrl Pts',(-8.55004304097738,2.2714104683578,0.414038291906306));
#33432=CARTESIAN_POINT('Ctrl Pts',(-8.43900352096466,0.88591264190158,2.1321097565203));
#33433=CARTESIAN_POINT('Ctrl Pts',(-8.32796400095198,-1.30915704620272,
1.90179942457344));
#33434=CARTESIAN_POINT('Ctrl Pts',(-8.21692448093929,-2.30788224507037,
-0.0664286520941292));
#33435=CARTESIAN_POINT('Ctrl Pts',(-8.1058849609266,-1.19759980905913,-1.9739523601829));
#33436=CARTESIAN_POINT('Ctrl Pts',(-7.9948454409139,1.00708297871625,-2.07762294387363));
#33437=CARTESIAN_POINT('Ctrl Pts',(-7.88380592090121,2.29146504681414,-0.282703311192433));
#33438=CARTESIAN_POINT('Ctrl Pts',(-7.77276640088852,1.48184197703646,1.77055854973022));
#33439=CARTESIAN_POINT('Ctrl Pts',(-7.66172688087582,-0.68192992331063,
2.20583426454112));
#33440=CARTESIAN_POINT('Ctrl Pts',(-7.55068736086314,-2.2225351010979,0.62535665609143));
#33441=CARTESIAN_POINT('Ctrl Pts',(-7.43964784085043,-1.73212526197346,
-1.52658943392238));
#33442=CARTESIAN_POINT('Ctrl Pts',(-7.32860832083775,0.341149305137663,
-2.28349521009661));
#33443=CARTESIAN_POINT('Ctrl Pts',(-7.21756880082505,2.10267205271563,-0.953678909098191));
#33444=CARTESIAN_POINT('Ctrl Pts',(-7.10652928081236,1.94271400451386,1.24763597238771));
#33445=CARTESIAN_POINT('Ctrl Pts',(-6.99548976079966,0.00744931895763328,
2.3088260503072));
#33446=CARTESIAN_POINT('Ctrl Pts',(-6.88445024078697,-1.9346227635487,1.26014601760641));
#33447=CARTESIAN_POINT('Ctrl Pts',(-6.77341072077428,-2.10878221201579,
-0.940090849448));
#33448=CARTESIAN_POINT('Ctrl Pts',(-6.66237120076159,-0.355877229471387,
-2.28124628667617));
#33449=CARTESIAN_POINT('Ctrl Pts',(-6.55133168074889,1.72223836363943,-1.53773477613621));
#33450=CARTESIAN_POINT('Ctrl Pts',(-6.4402921607362,2.22652415423095,0.611001975083735));
#33451=CARTESIAN_POINT('Ctrl Pts',(-6.32925264072351,0.69614961908643,2.2013879555353));
#33452=CARTESIAN_POINT('Ctrl Pts',(-6.21821312071081,-1.47038599611639,
1.78008377481369));
#33453=CARTESIAN_POINT('Ctrl Pts',(-6.10717360069812,-2.29324157796728,
-0.267910970309621));
#33454=CARTESIAN_POINT('Ctrl Pts',(-5.99613408068543,-1.02046857786368,
-2.07108114387703));
#33455=CARTESIAN_POINT('Ctrl Pts',(-5.88509456067273,1.18483727848316,-1.98163918169952));
#33456=CARTESIAN_POINT('Ctrl Pts',(-5.77405504066004,2.30740554206606,-0.0813196616628663));
#33457=CARTESIAN_POINT('Ctrl Pts',(-5.66301552064734,1.32140179536823,1.89331204985541));
#33458=CARTESIAN_POINT('Ctrl Pts',(-5.55197600063466,-0.872136036366616,
2.13778201812083));
#33459=CARTESIAN_POINT('Ctrl Pts',(-5.44093648062196,-2.26869145564129,
0.428686717814187));
#33460=CARTESIAN_POINT('Ctrl Pts',(-5.32989696060927,-1.59205288447209,
-1.67215454906962));
#33461=CARTESIAN_POINT('Ctrl Pts',(-5.21885744059657,0.539448340827144,
-2.24493401027935));
#33462=CARTESIAN_POINT('Ctrl Pts',(-5.10781792058389,2.17798651662185,-0.766229702076018));
#33463=CARTESIAN_POINT('Ctrl Pts',(-4.99677840057118,1.82621942357963,1.41267683490264));
#33464=CARTESIAN_POINT('Ctrl Pts',(-4.8857388805585,-0.194398285875258,
2.30063959136994));
#33465=CARTESIAN_POINT('Ctrl Pts',(-4.7746993605458,-2.03736938012958,1.08621325339021));
#33466=CARTESIAN_POINT('Ctrl Pts',(-4.66365984053311,-2.01853509547436,
-1.12082527240798));
#33467=CARTESIAN_POINT('Ctrl Pts',(-4.55262032052042,-0.155106730371774,
-2.30362217499385));
#33468=CARTESIAN_POINT('Ctrl Pts',(-4.44158080050772,1.85006252262662,-1.38130441442235));
#33469=CARTESIAN_POINT('Ctrl Pts',(-4.33054128049504,2.16459266543765,0.803288127425982));
#33470=CARTESIAN_POINT('Ctrl Pts',(-4.21950176048233,0.501057216920676,
2.25381341026746));
#33471=CARTESIAN_POINT('Ctrl Pts',(-4.10846224046965,-1.62035839348706,
1.64474067852272));
#33472=CARTESIAN_POINT('Ctrl Pts',(-3.99742272045695,-2.26104498039055,
-0.467342293805651));
#33473=CARTESIAN_POINT('Ctrl Pts',(-3.88638320044426,-0.835525140761208,
-2.15235474819651));
#33474=CARTESIAN_POINT('Ctrl Pts',(-3.77534368043157,1.35352104635311,-1.8704849638577));
#33475=CARTESIAN_POINT('Ctrl Pts',(-3.66430416041887,2.30568167449427,0.120686531233159));
#33476=CARTESIAN_POINT('Ctrl Pts',(-3.55326464040618,1.15084561098174,2.00157128341837));
#33477=CARTESIAN_POINT('Ctrl Pts',(-3.44222512039349,-1.055665504561,2.05336396322383));
#33478=CARTESIAN_POINT('Ctrl Pts',(-3.3311856003808,-2.29747982336605,0.228734964692146));
#33479=CARTESIAN_POINT('Ctrl Pts',(-3.2201460803681,-1.43979253255639,-1.80491847076076));
#33480=CARTESIAN_POINT('Ctrl Pts',(-3.10910656035541,0.733617625198351,
-2.18918669904949));
#33481=CARTESIAN_POINT('Ctrl Pts',(-2.99806704034272,2.23662738604792,-0.572914616908127));
#33482=CARTESIAN_POINT('Ctrl Pts',(-2.88702752033002,1.69574420447561,1.56690293761921));
#33483=CARTESIAN_POINT('Ctrl Pts',(-2.77598800031733,-0.394757673379551,
2.27484056684494));
#33484=CARTESIAN_POINT('Ctrl Pts',(-2.66494848030463,-2.12451889725514,
0.903964973503894));
#33485=CARTESIAN_POINT('Ctrl Pts',(-2.55390896029194,-1.91283506775852,
-1.29297920633453));
#33486=CARTESIAN_POINT('Ctrl Pts',(-2.44286944027925,0.0468511924372969,
-2.30836266712224));
#33487=CARTESIAN_POINT('Ctrl Pts',(-2.33182992026656,1.96372350683224,-1.21429945920298));
#33488=CARTESIAN_POINT('Ctrl Pts',(-2.22079040025386,2.08609012919687,0.989424689671358));
#33489=CARTESIAN_POINT('Ctrl Pts',(-2.10975088024117,0.302128947588233,
2.28898479809507));
#33490=CARTESIAN_POINT('Ctrl Pts',(-1.99871136022848,-1.75792608649789,
1.49680621617262));
#33491=CARTESIAN_POINT('Ctrl Pts',(-1.88767184021578,-2.21153900378128,
-0.663195798735933));
#33492=CARTESIAN_POINT('Ctrl Pts',(-1.77663232020309,-0.644185200405014,
-2.21715112630666));
#33493=CARTESIAN_POINT('Ctrl Pts',(-1.6655928001904,1.51184266846055,-1.74501095853683));
#33494=CARTESIAN_POINT('Ctrl Pts',(-1.55455328017771,2.28630712417556,0.321768286248855));
#33495=CARTESIAN_POINT('Ctrl Pts',(-1.44351376016501,0.971478199189345,
2.09450846247627));
#33496=CARTESIAN_POINT('Ctrl Pts',(-1.33247424015232,-1.2311115678387,1.9532244763376));
#33497=CARTESIAN_POINT('Ctrl Pts',(-1.22143472013963,-2.3086831418981,0.0270357188913206));
#33498=CARTESIAN_POINT('Ctrl Pts',(-1.11039520012693,-1.27650350580558,
-1.92387165415099));
#33499=CARTESIAN_POINT('Ctrl Pts',(-0.999355680114239,0.922158647667554,
-2.11666705375319));
#33500=CARTESIAN_POINT('Ctrl Pts',(-0.888316160101547,2.27816865573076,
-0.375238308250741));
#33501=CARTESIAN_POINT('Ctrl Pts',(-0.777276640088857,1.55224358940625,
1.7091806553938));
#33502=CARTESIAN_POINT('Ctrl Pts',(-0.666237120076159,-0.592012005603808,
2.23153694542934));
#33503=CARTESIAN_POINT('Ctrl Pts',(-0.555197600063465,-2.1955620628257,
0.714966780555073));
#33504=CARTESIAN_POINT('Ctrl Pts',(-0.444158080050777,-1.79219063562177,
-1.45555925698041));
#33505=CARTESIAN_POINT('Ctrl Pts',(-0.33311856003808,0.247876640334474,
-2.29481134042266));
#33506=CARTESIAN_POINT('Ctrl Pts',(-0.22207904002539,2.0634575466964,-1.03920101979834));
#33507=CARTESIAN_POINT('Ctrl Pts',(-0.111039520012697,1.98938703685113,
1.170468582496));
#33508=CARTESIAN_POINT('Ctrl Pts',(-0.0370131733375646,0.733938965798303,
1.92376702457974));
#33509=CARTESIAN_POINT('Ctrl Pts',(0.,0.0853826423430472,1.95213365433479));
#33510=CARTESIAN_POINT('Ctrl Pts',(-19.7993827215147,1.0579354195126,-1.48236995244726));
#33511=CARTESIAN_POINT('Ctrl Pts',(-19.7623695481771,1.55042239868275,-1.1308926319223));
#33512=CARTESIAN_POINT('Ctrl Pts',(-19.688343201502,2.14914912251819,0.0953190480300262));
#33513=CARTESIAN_POINT('Ctrl Pts',(-19.5773036814893,1.08507218969133,1.85993354136436));
#33514=CARTESIAN_POINT('Ctrl Pts',(-19.4662641614766,-0.971466826935683,
1.91940918152277));
#33515=CARTESIAN_POINT('Ctrl Pts',(-19.3552246414639,-2.13978277206915,
0.227625634517308));
#33516=CARTESIAN_POINT('Ctrl Pts',(-19.2441851214512,-1.35295187154209,
-1.67359931093053));
#33517=CARTESIAN_POINT('Ctrl Pts',(-19.1331456014385,0.670374159930676,
-2.0446920186307));
#33518=CARTESIAN_POINT('Ctrl Pts',(-19.0221060814259,2.08102528428471,-0.547681768149684));
#33519=CARTESIAN_POINT('Ctrl Pts',(-18.9110665614132,1.59001286315942,1.4500225431683));
#33520=CARTESIAN_POINT('Ctrl Pts',(-18.8000270414005,-0.354016811486251,
2.12254668997377));
#33521=CARTESIAN_POINT('Ctrl Pts',(-18.6889875213878,-1.97452608250074,
0.855485233373004));
#33522=CARTESIAN_POINT('Ctrl Pts',(-18.5779480013751,-1.79066314608461,
-1.19337272293876));
#33523=CARTESIAN_POINT('Ctrl Pts',(-18.4669084813624,0.0295608146065764,
-2.15167735991307));
#33524=CARTESIAN_POINT('Ctrl Pts',(-18.3558689613497,1.82276983596386,-1.14372707715715));
#33525=CARTESIAN_POINT('Ctrl Pts',(-18.244829441337,1.95028132592011,0.909397504879913));
#33526=CARTESIAN_POINT('Ctrl Pts',(-18.1337899213243,0.295570550858466,
2.13148680442571));
#33527=CARTESIAN_POINT('Ctrl Pts',(-18.0227504013116,-1.62924068903274,
1.40576478377186));
#33528=CARTESIAN_POINT('Ctrl Pts',(-17.9117108812989,-2.06520612379439,
-0.604585224298059));
#33529=CARTESIAN_POINT('Ctrl Pts',(-17.8006713612862,-0.613928123624273,
-2.06244793584588));
#33530=CARTESIAN_POINT('Ctrl Pts',(-17.6896318412735,1.39837461379019,-1.63558795465258));
#33531=CARTESIAN_POINT('Ctrl Pts',(-17.5785923212608,2.13280335807138,0.285918342857852));
#33532=CARTESIAN_POINT('Ctrl Pts',(-17.4675528012481,0.918216464846976,
1.94614437754049));
#33533=CARTESIAN_POINT('Ctrl Pts',(-17.3565132812355,-1.13546242660618,
1.8279290290191));
#33534=CARTESIAN_POINT('Ctrl Pts',(-17.2454737612228,-2.15152385442317,
0.0393007652556636));
#33535=CARTESIAN_POINT('Ctrl Pts',(-17.1344342412101,-1.20146233636809,
-1.78524163492781));
#33536=CARTESIAN_POINT('Ctrl Pts',(-17.0233947211974,0.846529218784861,
-1.97838007691544));
#33537=CARTESIAN_POINT('Ctrl Pts',(-16.9123552011847,2.12093859113575,-0.363619220621685));
#33538=CARTESIAN_POINT('Ctrl Pts',(-16.801315681172,1.4571746915289,1.58342709424245));
#33539=CARTESIAN_POINT('Ctrl Pts',(-16.6902761611593,-0.53819638003717,
2.08349324496288));
#33540=CARTESIAN_POINT('Ctrl Pts',(-16.5792366411466,-2.04174847909078,
0.679604732970229));
#33541=CARTESIAN_POINT('Ctrl Pts',(-16.4681971211339,-1.67949345554894,
-1.34532567717577));
#33542=CARTESIAN_POINT('Ctrl Pts',(-16.3571576011212,0.217529872578918,
-2.14085968703163));
#33543=CARTESIAN_POINT('Ctrl Pts',(-16.2461180811086,1.91576829170772,-0.980015967957599));
#33544=CARTESIAN_POINT('Ctrl Pts',(-16.1350785610958,1.8633238228732,1.07639387590079));
#33545=CARTESIAN_POINT('Ctrl Pts',(-16.0240390410832,0.108121695115326,
2.14916475497463));
#33546=CARTESIAN_POINT('Ctrl Pts',(-15.9129995210704,-1.74588507529003,
1.25796850073853));
#33547=CARTESIAN_POINT('Ctrl Pts',(-15.8019600010578,-2.0044530137212,-0.782794711757463));
#33548=CARTESIAN_POINT('Ctrl Pts',(-15.6909204810451,-0.431295473643615,
-2.10821812424334));
#33549=CARTESIAN_POINT('Ctrl Pts',(-15.5798809610324,1.53599198738047,-1.50709258497119));
#33550=CARTESIAN_POINT('Ctrl Pts',(-15.4688414410197,2.09964681705268,0.471256499809728));
#33551=CARTESIAN_POINT('Ctrl Pts',(-15.357801921007,0.744585396287178,2.0189581552396));
#33552=CARTESIAN_POINT('Ctrl Pts',(-15.2467624009943,-1.29089907853287,
1.72167912632273));
#33553=CARTESIAN_POINT('Ctrl Pts',(-15.1357228809816,-2.14672370792567,
-0.148918658341753));
#33554=CARTESIAN_POINT('Ctrl Pts',(-15.0246833609689,-1.04081190138835,
-1.88343038918375));
#33555=CARTESIAN_POINT('Ctrl Pts',(-14.9136438409562,1.01622306196928,-1.89681051591725));
#33556=CARTESIAN_POINT('Ctrl Pts',(-14.8026043209435,2.14460484078461,-0.176831902822113));
#33557=CARTESIAN_POINT('Ctrl Pts',(-14.6915648009308,1.31318646399232,1.70474067111682));
#33558=CARTESIAN_POINT('Ctrl Pts',(-14.5805252809181,-0.718258597218173,
2.0284733255566));
#33559=CARTESIAN_POINT('Ctrl Pts',(-14.4694857609054,-2.09333877300777,
0.498530065687933));
#33560=CARTESIAN_POINT('Ctrl Pts',(-14.3584462408927,-1.55546716623066,
-1.48698397427506));
#33561=CARTESIAN_POINT('Ctrl Pts',(-14.24740672088,0.403834037481487,-2.11365028212897));
#33562=CARTESIAN_POINT('Ctrl Pts',(-14.1363672008674,1.99410035213392,-0.808803579734818));
#33563=CARTESIAN_POINT('Ctrl Pts',(-14.0253276808547,1.76210174129103,1.23515055694098));
#33564=CARTESIAN_POINT('Ctrl Pts',(-13.914288160842,-0.0801549465201214,
2.15038941346001));
#33565=CARTESIAN_POINT('Ctrl Pts',(-13.8032486408293,-1.84916379226943,
1.10054200934459));
#33566=CARTESIAN_POINT('Ctrl Pts',(-13.6922091208166,-1.92835481288141,
-0.955011602342901));
#33567=CARTESIAN_POINT('Ctrl Pts',(-13.5811696008039,-0.245361028870353,
-2.13784878101426));
#33568=CARTESIAN_POINT('Ctrl Pts',(-13.4701300807912,1.66185055667484,-1.36705968130584));
#33569=CARTESIAN_POINT('Ctrl Pts',(-13.3590905607785,2.05041641428424,0.652986962355509));
#33570=CARTESIAN_POINT('Ctrl Pts',(-13.2480510407658,0.565254146620652,
2.07631577432255));
#33571=CARTESIAN_POINT('Ctrl Pts',(-13.1370115207531,-1.43645324088873,
1.60224889817803));
#33572=CARTESIAN_POINT('Ctrl Pts',(-13.0259720007404,-2.12548930010491,
-0.335998035875247));
#33573=CARTESIAN_POINT('Ctrl Pts',(-12.9149324807277,-0.87219352183257,
-1.9672005249709));
#33574=CARTESIAN_POINT('Ctrl Pts',(-12.803892960715,1.1781372007338,-1.80071990637623));
#33575=CARTESIAN_POINT('Ctrl Pts',(-12.6928534407024,2.15185304982047,0.0113091534085617));
#33576=CARTESIAN_POINT('Ctrl Pts',(-12.5818139206897,1.15914512624606,1.81300359108097));
#33577=CARTESIAN_POINT('Ctrl Pts',(-12.470774400677,-0.892822179563889,
1.95792441137325));
#33578=CARTESIAN_POINT('Ctrl Pts',(-12.3597348806643,-2.12890349408833,
0.313638897190672));
#33579=CARTESIAN_POINT('Ctrl Pts',(-12.2486953606516,-1.41953298474134,
-1.61725865284556));
#33580=CARTESIAN_POINT('Ctrl Pts',(-12.1376558406389,0.587046647461331,
-2.07025980946279));
#33581=CARTESIAN_POINT('Ctrl Pts',(-12.0266163206262,2.05716656029549,-0.631399388798012));
#33582=CARTESIAN_POINT('Ctrl Pts',(-11.9155768006135,1.64738987478806,1.38445153234711));
#33583=CARTESIAN_POINT('Ctrl Pts',(-11.8045372806008,-0.267817961278038,
2.13515174743843));
#33584=CARTESIAN_POINT('Ctrl Pts',(-11.6934977605881,-1.93828622005437,
0.934690309203982));
#33585=CARTESIAN_POINT('Ctrl Pts',(-11.5824582405754,-1.83749407531276,
-1.11991739345498));
#33586=CARTESIAN_POINT('Ctrl Pts',(-11.4714187205627,-0.0575482206464092,
-2.15111311819553));
#33587=CARTESIAN_POINT('Ctrl Pts',(-11.36037920055,1.77498681484848,-1.21656124058205));
#33588=CARTESIAN_POINT('Ctrl Pts',(-11.2493396805373,1.98548903115562,0.829718477637558));
#33589=CARTESIAN_POINT('Ctrl Pts',(-11.1383001605246,0.381595589010167,
2.11777814027354));
#33590=CARTESIAN_POINT('Ctrl Pts',(-11.027260640512,-1.57101062319865,1.47055263991789));
#33591=CARTESIAN_POINT('Ctrl Pts',(-10.9162211204993,-2.08798319080583,
-0.520505177577319));
#33592=CARTESIAN_POINT('Ctrl Pts',(-10.8051816004866,-0.696898057326079,
-2.03591074034881));
#33593=CARTESIAN_POINT('Ctrl Pts',(-10.6941420804739,1.33103210010252,-1.69084387022254));
#33594=CARTESIAN_POINT('Ctrl Pts',(-10.5831025604612,2.14262772946706,0.199363632318784));
#33595=CARTESIAN_POINT('Ctrl Pts',(-10.4720630404485,0.99622994309236,1.90738704657934));
#33596=CARTESIAN_POINT('Ctrl Pts',(-10.3610235204358,-1.06055075409358,
1.87238659014746));
#33597=CARTESIAN_POINT('Ctrl Pts',(-10.2499840004231,-2.1481703762994,0.126346663439019));
#33598=CARTESIAN_POINT('Ctrl Pts',(-10.1389444804104,-1.27273155637141,
-1.73515239399567));
#33599=CARTESIAN_POINT('Ctrl Pts',(-10.0279049603977,0.765765116820998,
-2.01102044515529));
#33600=CARTESIAN_POINT('Ctrl Pts',(-9.91686544038503,2.10448411229651,-0.449161514451188));
#33601=CARTESIAN_POINT('Ctrl Pts',(-9.80582592037233,1.52006640103793,1.52315382723088));
#33602=CARTESIAN_POINT('Ctrl Pts',(-9.69478640035963,-0.453430693347546,
2.1035684089905));
#33603=CARTESIAN_POINT('Ctrl Pts',(-9.58374688034695,-2.01257008113814,
0.76168307942353));
#33604=CARTESIAN_POINT('Ctrl Pts',(-9.47270736033426,-1.73256638616727,
-1.2762496474028));
#33605=CARTESIAN_POINT('Ctrl Pts',(-9.36166784032154,0.130705148471866,
-2.1479095905404));
#33606=CARTESIAN_POINT('Ctrl Pts',(-9.25062832030888,1.87453464631127,-1.05674940489747));
#33607=CARTESIAN_POINT('Ctrl Pts',(-9.13958880029616,1.90536171980257,1.00009807603229));
#33608=CARTESIAN_POINT('Ctrl Pts',(-9.02854928028348,0.195015723111051,
2.14302783759613));
#33609=CARTESIAN_POINT('Ctrl Pts',(-8.91750976027079,-1.69354112027386,
1.32759855337147));
#33610=CARTESIAN_POINT('Ctrl Pts',(-8.80647024025808,-2.0344925083683,-0.70102758744985));
#33611=CARTESIAN_POINT('Ctrl Pts',(-8.69543072024542,-0.516267483793617,
-2.08903502367717));
#33612=CARTESIAN_POINT('Ctrl Pts',(-8.58439120023269,1.47373727186836,-1.56802356438877));
#33613=CARTESIAN_POINT('Ctrl Pts',(-8.47335168022003,2.11699950424307,0.385891881240195));
#33614=CARTESIAN_POINT('Ctrl Pts',(-8.36231216020731,0.825688113106338,
1.98716848426282));
#33615=CARTESIAN_POINT('Ctrl Pts',(-8.25127264019463,-1.22016027327337,
1.7725146973997));
#33616=CARTESIAN_POINT('Ctrl Pts',(-8.14023312018193,-2.15099192185977,
-0.0619128182729752));
#33617=CARTESIAN_POINT('Ctrl Pts',(-8.02919360016924,-1.11618672070874,
-1.83976266118376));
#33618=CARTESIAN_POINT('Ctrl Pts',(-7.91815408015655,0.938621264792929,
-1.93638569666557));
#33619=CARTESIAN_POINT('Ctrl Pts',(-7.80711456014386,2.13569076821376,-0.263485080296819));
#33620=CARTESIAN_POINT('Ctrl Pts',(-7.69607504013116,1.38110604598068,1.65019560498993));
#33621=CARTESIAN_POINT('Ctrl Pts',(-7.58503552011847,-0.635572182874023,
2.05588118463331));
#33622=CARTESIAN_POINT('Ctrl Pts',(-7.47399600010578,-2.07144669478819,
0.582844778327466));
#33623=CARTESIAN_POINT('Ctrl Pts',(-7.36295648009308,-1.61437502026476,
-1.42281156128196));
#33624=CARTESIAN_POINT('Ctrl Pts',(-7.25191696008039,0.317957903210428,
-2.12826272268217));
#33625=CARTESIAN_POINT('Ctrl Pts',(-7.1408774400677,1.9597319617898,-0.888847615124196));
#33626=CARTESIAN_POINT('Ctrl Pts',(-7.029837920055,1.81064789554103,1.16282141506997));
#33627=CARTESIAN_POINT('Ctrl Pts',(-6.91879840004231,0.00694291267913799,
2.15187156701696));
#33628=CARTESIAN_POINT('Ctrl Pts',(-6.80775888002961,-1.80310669884822,
1.17448102476845));
#33629=CARTESIAN_POINT('Ctrl Pts',(-6.69671936001694,-1.96542675116825,
-0.876183274643305));
#33630=CARTESIAN_POINT('Ctrl Pts',(-6.58567984000421,-0.331684620132549,
-2.12616668155156));
#33631=CARTESIAN_POINT('Ctrl Pts',(-6.47464031999155,1.60516023537086,-1.43319924077452));
#33632=CARTESIAN_POINT('Ctrl Pts',(-6.36360079997884,2.07516457124545,0.569465931571117));
#33633=CARTESIAN_POINT('Ctrl Pts',(-6.25256127996616,0.648825220723096,
2.05173713665423));
#33634=CARTESIAN_POINT('Ctrl Pts',(-6.14152175995345,-1.37042884506684,
1.65907330325736));
#33635=CARTESIAN_POINT('Ctrl Pts',(-6.03048223994078,-2.13734653040332,
-0.249698325876242));
#33636=CARTESIAN_POINT('Ctrl Pts',(-5.91944271992806,-0.951096908078864,
-1.93028860961653));
#33637=CARTESIAN_POINT('Ctrl Pts',(-5.80840319991538,1.10429178966098,-1.84692693094769));
#33638=CARTESIAN_POINT('Ctrl Pts',(-5.69736367990268,2.15054762522653,-0.0757915338613339));
#33639=CARTESIAN_POINT('Ctrl Pts',(-5.58632415989,1.23157262180047,1.76460429621033));
#33640=CARTESIAN_POINT('Ctrl Pts',(-5.47528463987729,-0.812848044129805,
1.99245514431989));
#33641=CARTESIAN_POINT('Ctrl Pts',(-5.36424511986461,-2.11446533058618,
0.399544504056276));
#33642=CARTESIAN_POINT('Ctrl Pts',(-5.25320559985191,-1.48382479261571,
-1.55848112910982));
#33643=CARTESIAN_POINT('Ctrl Pts',(-5.14216607983922,0.502776528507167,
-2.09232292138541));
#33644=CARTESIAN_POINT('Ctrl Pts',(-5.03112655982653,2.02992653250826,-0.714141244846878));
#33645=CARTESIAN_POINT('Ctrl Pts',(-4.92008703981383,1.70207264086103,1.31664276483973));
#33646=CARTESIAN_POINT('Ctrl Pts',(-4.80904751980114,-0.181183049280004,
2.14424162528995));
#33647=CARTESIAN_POINT('Ctrl Pts',(-4.69800799978845,-1.89886857869975,
1.012372246656));
#33648=CARTESIAN_POINT('Ctrl Pts',(-4.58696847977575,-1.88131465269946,
-1.04463133329937));
#33649=CARTESIAN_POINT('Ctrl Pts',(-4.47592895976307,-0.144562542031095,
-2.14702145224819));
#33650=CARTESIAN_POINT('Ctrl Pts',(-4.36488943975037,1.72429488099121,-1.28740304813998));
#33651=CARTESIAN_POINT('Ctrl Pts',(-4.25384991973768,2.0174431981608,0.748680430602484));
#33652=CARTESIAN_POINT('Ctrl Pts',(-4.14281039972499,0.466995241324839,
2.10059869788404));
#33653=CARTESIAN_POINT('Ctrl Pts',(-4.03177087971229,-1.51020608714031,
1.53293085928163));
#33654=CARTESIAN_POINT('Ctrl Pts',(-3.9207313596996,-2.10733866434047,-0.435572265814925));
#33655=CARTESIAN_POINT('Ctrl Pts',(-3.8096918396869,-0.778725964952054,
-2.00603721712242));
#33656=CARTESIAN_POINT('Ctrl Pts',(-3.69865231967421,1.26150839930913,-1.74332900034742));
#33657=CARTESIAN_POINT('Ctrl Pts',(-3.58761279966152,2.14894094653692,0.112482235310861));
#33658=CARTESIAN_POINT('Ctrl Pts',(-3.47657327964882,1.07261088290665,1.86550404417541));
#33659=CARTESIAN_POINT('Ctrl Pts',(-3.36553375963613,-0.983901140254003,
1.9137758466519));
#33660=CARTESIAN_POINT('Ctrl Pts',(-3.25449423962344,-2.14129665898335,
0.213185513407649));
#33661=CARTESIAN_POINT('Ctrl Pts',(-3.14345471961075,-1.34191513163117,
-1.68221973132061));
#33662=CARTESIAN_POINT('Ctrl Pts',(-3.03241519959805,0.683746143853823,
-2.04036532416529));
#33663=CARTESIAN_POINT('Ctrl Pts',(-2.92137567958536,2.08458098322634,-0.533967760061011));
#33664=CARTESIAN_POINT('Ctrl Pts',(-2.81033615957267,1.58046715475138,1.46038454446989));
#33665=CARTESIAN_POINT('Ctrl Pts',(-2.69929663955997,-0.367921963239354,
2.12019642390948));
#33666=CARTESIAN_POINT('Ctrl Pts',(-2.58825711954728,-1.98009365321621,
0.842513243387684));
#33667=CARTESIAN_POINT('Ctrl Pts',(-2.47721759953459,-1.78280013522666,
-1.20508220638155));
#33668=CARTESIAN_POINT('Ctrl Pts',(-2.36617807952189,0.0436662384648719,
-2.15143968471892));
#33669=CARTESIAN_POINT('Ctrl Pts',(-2.2551385595092,1.83022916744761,-1.1317511251033));
#33670=CARTESIAN_POINT('Ctrl Pts',(-2.14409903949651,1.94427728093947,0.9221633899726));
#33671=CARTESIAN_POINT('Ctrl Pts',(-2.03305951948381,0.281590157821288,
2.13337912732726));
#33672=CARTESIAN_POINT('Ctrl Pts',(-1.92201999947113,-1.6384218992803,1.39505301297495));
#33673=CARTESIAN_POINT('Ctrl Pts',(-1.81098047945843,-2.06119811449319,
-0.61811160805078));
#33674=CARTESIAN_POINT('Ctrl Pts',(-1.69994095944574,-0.600393354215775,
-2.06642872374214));
#33675=CARTESIAN_POINT('Ctrl Pts',(-1.58890143943304,1.40906728405564,-1.62638474445002));
#33676=CARTESIAN_POINT('Ctrl Pts',(-1.47786191942035,2.13088348224722,0.299894410085385));
#33677=CARTESIAN_POINT('Ctrl Pts',(-1.36682239940766,0.905436905709838,
1.95212333414178));
#33678=CARTESIAN_POINT('Ctrl Pts',(-1.25578287939496,-1.14742034303764,
1.82044386326689));
#33679=CARTESIAN_POINT('Ctrl Pts',(-1.14474335938227,-2.15173837355173,
0.0251978250021854));
#33680=CARTESIAN_POINT('Ctrl Pts',(-1.03370383936958,-1.18972652745971,
-1.79308645214156));
#33681=CARTESIAN_POINT('Ctrl Pts',(-0.922664319356884,0.859470107733127,
-1.97277557969645));
#33682=CARTESIAN_POINT('Ctrl Pts',(-0.811624799344192,2.12329826860884,
-0.349729528680995));
#33683=CARTESIAN_POINT('Ctrl Pts',(-0.700585279331502,1.44672174184939,
1.59299019289389));
#33684=CARTESIAN_POINT('Ctrl Pts',(-0.589545759318803,-0.55176690423342,
2.07983659183781));
#33685=CARTESIAN_POINT('Ctrl Pts',(-0.478506239306111,-2.04630728936339,
0.66636318757467));
#33686=CARTESIAN_POINT('Ctrl Pts',(-0.367466719293421,-1.67035713710672,
-1.35661003079366));
#33687=CARTESIAN_POINT('Ctrl Pts',(-0.256427199280725,0.231025933890705,
-2.13880958007493));
#33688=CARTESIAN_POINT('Ctrl Pts',(-0.145387679268034,1.92318326618488,
-0.968555914648296));
#33689=CARTESIAN_POINT('Ctrl Pts',(-0.0343481592553421,1.85414808526718,
1.09089988066647));
#33690=CARTESIAN_POINT('Ctrl Pts',(0.0396781874197904,0.684045639651843,
1.79298893531071));
#33691=CARTESIAN_POINT('Ctrl Pts',(0.0766913607573549,0.0795783122554267,
1.81942719557457));
#33692=CARTESIAN_POINT('Ctrl Pts',(-19.7226913607574,0.980771099081406,
-1.37424797458504));
#33693=CARTESIAN_POINT('Ctrl Pts',(-19.6856781874198,1.43733677117747,-1.04840691510689));
#33694=CARTESIAN_POINT('Ctrl Pts',(-19.6116518407446,1.99239321049778,0.0883666108304189));
#33695=CARTESIAN_POINT('Ctrl Pts',(-19.500612320732,1.00592855143894,1.72427260675583));
#33696=CARTESIAN_POINT('Ctrl Pts',(-19.3895728007192,-0.900609403940542,
1.77941017743441));
#33697=CARTESIAN_POINT('Ctrl Pts',(-19.2785332807066,-1.98371002846714,
0.211022941123868));
#33698=CARTESIAN_POINT('Ctrl Pts',(-19.1674937606938,-1.25426946634223,
-1.55152933282018));
#33699=CARTESIAN_POINT('Ctrl Pts',(-19.0564542406812,0.621478012272129,
-1.89555506074211));
#33700=CARTESIAN_POINT('Ctrl Pts',(-18.9454147206685,1.92923822913921,-0.507734630855354));
#33701=CARTESIAN_POINT('Ctrl Pts',(-18.8343752006558,1.4740395628997,1.34425993980917));
#33702=CARTESIAN_POINT('Ctrl Pts',(-18.7233356806431,-0.328195323543107,
1.96773112193963));
#33703=CARTESIAN_POINT('Ctrl Pts',(-18.6122961606304,-1.83050692923332,
0.793087344565633));
#33704=CARTESIAN_POINT('Ctrl Pts',(-18.5012566406177,-1.66005469660814,
-1.10632979622673));
#33705=CARTESIAN_POINT('Ctrl Pts',(-18.390217120605,0.0274046903966734,
-1.99473704181564));
#33706=CARTESIAN_POINT('Ctrl Pts',(-18.2791776005923,1.68981956971848,-1.06030523397109));
#33707=CARTESIAN_POINT('Ctrl Pts',(-18.1681380805796,1.80803055107265,0.843067330871544));
#33708=CARTESIAN_POINT('Ctrl Pts',(-18.0570985605669,0.274012050901109,
1.97601915702686));
#33709=CARTESIAN_POINT('Ctrl Pts',(-17.9460590405543,-1.51040616636786,
1.30323027908932));
#33710=CARTESIAN_POINT('Ctrl Pts',(-17.8350195205416,-1.91457289594923,
-0.56048762900514));
#33711=CARTESIAN_POINT('Ctrl Pts',(-17.7239800005289,-0.569149070404872,
-1.91201588634746));
#33712=CARTESIAN_POINT('Ctrl Pts',(-17.6129404805162,1.29637913770427,-1.51629047136732));
#33713=CARTESIAN_POINT('Ctrl Pts',(-17.5019009605035,1.9772396831027,0.265063861366327));
#33714=CARTESIAN_POINT('Ctrl Pts',(-17.3908614404908,0.851243048311522,
1.80419534588497));
#33715=CARTESIAN_POINT('Ctrl Pts',(-17.2798219204781,-1.05264339539859,
1.69460245849397));
#33716=CARTESIAN_POINT('Ctrl Pts',(-17.1687824004654,-1.99459473280011,
0.0364342227546489));
#33717=CARTESIAN_POINT('Ctrl Pts',(-17.0577428804527,-1.11382936463886,
-1.65502862284421));
#33718=CARTESIAN_POINT('Ctrl Pts',(-16.9467033604401,0.784784569075727,
-1.83407981872));
#33719=CARTESIAN_POINT('Ctrl Pts',(-16.8356638404273,1.96624031556741,-0.337097346471846));
#33720=CARTESIAN_POINT('Ctrl Pts',(-16.7246243204147,1.35089042053518,1.4679341506979));
#33721=CARTESIAN_POINT('Ctrl Pts',(-16.6135848004019,-0.498941093600838,
1.93152618023922));
#33722=CARTESIAN_POINT('Ctrl Pts',(-16.5025452803893,-1.89282621883312,
0.630035320306451));
#33723=CARTESIAN_POINT('Ctrl Pts',(-16.3915057603766,-1.55699356682629,
-1.24719951585892));
#33724=CARTESIAN_POINT('Ctrl Pts',(-16.2804662403639,0.201663549851218,
-1.98470839476804));
#33725=CARTESIAN_POINT('Ctrl Pts',(-16.1694267203512,1.77603484899781,-0.908534982649458));
#33726=CARTESIAN_POINT('Ctrl Pts',(-16.0583872003385,1.72741560590332,0.99788322164133));
#33727=CARTESIAN_POINT('Ctrl Pts',(-15.9473476803258,0.100235450857364,
1.99240770274486));
#33728=CARTESIAN_POINT('Ctrl Pts',(-15.8363081603131,-1.61854267527115,
1.16621404891383));
#33729=CARTESIAN_POINT('Ctrl Pts',(-15.7252686403004,-1.8582510322134,-0.725698767283147));
#33730=CARTESIAN_POINT('Ctrl Pts',(-15.6142291202877,-0.399837388854213,
-1.95444766162579));
#33731=CARTESIAN_POINT('Ctrl Pts',(-15.503189600275,1.42395889376444,-1.39716737309035));
#33732=CARTESIAN_POINT('Ctrl Pts',(-15.3921500802623,1.94650153351731,0.436883714017789));
#33733=CARTESIAN_POINT('Ctrl Pts',(-15.2811105602496,0.690276385502817,
1.87169818912575));
#33734=CARTESIAN_POINT('Ctrl Pts',(-15.1700710402369,-1.19674271671436,
1.59610227415113));
#33735=CARTESIAN_POINT('Ctrl Pts',(-15.0590315202242,-1.99014470223182,
-0.138056741008676));
#33736=CARTESIAN_POINT('Ctrl Pts',(-14.9479920002116,-0.964896546267425,
-1.74605562756762));
#33737=CARTESIAN_POINT('Ctrl Pts',(-14.8369524801988,0.942101182186204,
-1.75845982669002));
#33738=CARTESIAN_POINT('Ctrl Pts',(-14.7259129601862,1.98818038227767,-0.163934032725192));
#33739=CARTESIAN_POINT('Ctrl Pts',(-14.6148734401735,1.21740449164842,1.58039928602666));
#33740=CARTESIAN_POINT('Ctrl Pts',(-14.5038339201608,-0.665869826102309,
1.88051933631266));
#33741=CARTESIAN_POINT('Ctrl Pts',(-14.3927944001481,-1.94065358932632,
0.462167984389029));
#33742=CARTESIAN_POINT('Ctrl Pts',(-14.2817548801354,-1.44201358048108,
-1.37852545615505));
#33743=CARTESIAN_POINT('Ctrl Pts',(-14.1707153601227,0.374378951193126,
-1.95948360556114));
#33744=CARTESIAN_POINT('Ctrl Pts',(-14.05967584011,1.84865347919068,-0.749810585038333));
#33745=CARTESIAN_POINT('Ctrl Pts',(-13.9486363200973,1.63357652047938,1.14506041382008));
#33746=CARTESIAN_POINT('Ctrl Pts',(-13.8375968000846,-0.0743085575408296,
1.99354303636404));
#33747=CARTESIAN_POINT('Ctrl Pts',(-13.7265572800719,-1.71428838800121,
1.02027002422082));
#33748=CARTESIAN_POINT('Ctrl Pts',(-13.6155177600592,-1.78770332703292,
-0.885354400268458));
#33749=CARTESIAN_POINT('Ctrl Pts',(-13.5044782400465,-0.227464740775772,
-1.98191709999766));
#33750=CARTESIAN_POINT('Ctrl Pts',(-13.3934387200338,1.54063751616327,-1.26734827231887));
#33751=CARTESIAN_POINT('Ctrl Pts',(-13.2823992000211,1.9008619270339,0.605359012415223));
#33752=CARTESIAN_POINT('Ctrl Pts',(-13.1713596800085,0.524025304774173,
1.92487222420494));
#33753=CARTESIAN_POINT('Ctrl Pts',(-13.0603201599958,-1.33168036333877,
1.48538311874655));
#33754=CARTESIAN_POINT('Ctrl Pts',(-12.9492806399831,-1.97045910222959,
-0.311490812063336));
#33755=CARTESIAN_POINT('Ctrl Pts',(-12.8382411199704,-0.808576953982255,
-1.82371568755882));
#33756=CARTESIAN_POINT('Ctrl Pts',(-12.7272015999577,1.09220553156706,-1.66937793095921));
#33757=CARTESIAN_POINT('Ctrl Pts',(-12.616162079945,1.99489991714847,0.0104842796768135));
#33758=CARTESIAN_POINT('Ctrl Pts',(-12.5051225599323,1.0745987122607,1.68076566099114));
#33759=CARTESIAN_POINT('Ctrl Pts',(-12.3940830399196,-0.827700986453924,
1.81511616063064));
#33760=CARTESIAN_POINT('Ctrl Pts',(-12.2830435199069,-1.97362426970941,
0.290762517483453));
#33761=CARTESIAN_POINT('Ctrl Pts',(-12.1720039998942,-1.31599424685915,
-1.49929808303518));
#33762=CARTESIAN_POINT('Ctrl Pts',(-12.0609644798815,0.544228291276939,
-1.91925797289815));
#33763=CARTESIAN_POINT('Ctrl Pts',(-11.9499249598688,1.90711972689606,-0.585346006088044));
#33764=CARTESIAN_POINT('Ctrl Pts',(-11.8388854398562,1.52723157605959,1.28347158622459));
#33765=CARTESIAN_POINT('Ctrl Pts',(-11.7278459198434,-0.248283696142248,
1.97941678425471));
#33766=CARTESIAN_POINT('Ctrl Pts',(-11.6168063998308,-1.79691035134536,
0.866515313648441));
#33767=CARTESIAN_POINT('Ctrl Pts',(-11.505766879818,-1.70346984377399,-1.03823219508546));
#33768=CARTESIAN_POINT('Ctrl Pts',(-11.3947273598054,-0.0533507344329003,
-1.99421395509479));
#33769=CARTESIAN_POINT('Ctrl Pts',(-11.2836878397927,1.64552177490757,-1.12782697603151));
#33770=CARTESIAN_POINT('Ctrl Pts',(-11.17264831978,1.84067025584392,0.76919997972621));
#33771=CARTESIAN_POINT('Ctrl Pts',(-11.0616087997673,0.353762543852217,
1.96331038354269));
#33772=CARTESIAN_POINT('Ctrl Pts',(-10.9505692797546,-1.45642331957557,
1.36329260019844));
#33773=CARTESIAN_POINT('Ctrl Pts',(-10.8395297597419,-1.93568863575209,
-0.48254026254764));
#33774=CARTESIAN_POINT('Ctrl Pts',(-10.7284902397292,-0.646067293924532,
-1.88741427653824));
#33775=CARTESIAN_POINT('Ctrl Pts',(-10.6174507197165,1.23394849217886,-1.56751609822957));
#33776=CARTESIAN_POINT('Ctrl Pts',(-10.5064111997038,1.98634747867679,0.184822329586263));
#33777=CARTESIAN_POINT('Ctrl Pts',(-10.3953716796911,0.923566333259427,
1.76826492009231));
#33778=CARTESIAN_POINT('Ctrl Pts',(-10.2843321596784,-0.983195674839188,
1.73581734768865));
#33779=CARTESIAN_POINT('Ctrl Pts',(-10.1732926396658,-1.99148585265059,
0.117131115643584));
#33780=CARTESIAN_POINT('Ctrl Pts',(-10.0622531196531,-1.17990030804818,
-1.60859282064391));
#33781=CARTESIAN_POINT('Ctrl Pts',(-9.95121359964037,0.709911287031804,
-1.8643394444425));
#33782=CARTESIAN_POINT('Ctrl Pts',(-9.84017407962766,1.95098600325465,-0.416400305792137));
#33783=CARTESIAN_POINT('Ctrl Pts',(-9.72913455961498,1.40919489727413,1.41205713094616));
#33784=CARTESIAN_POINT('Ctrl Pts',(-9.61809503960227,-0.420358096788729,
1.95013709005892));
#33785=CARTESIAN_POINT('Ctrl Pts',(-9.50705551958959,-1.86577605215789,
0.706126987696579));
#33786=CARTESIAN_POINT('Ctrl Pts',(-9.3960159995769,-1.60619543258667,-1.18316179447151));
#33787=CARTESIAN_POINT('Ctrl Pts',(-9.28497647956421,0.12117169891277,-1.99124408823779));
#33788=CARTESIAN_POINT('Ctrl Pts',(-9.17393695955151,1.73780872765929,-0.979671590702989));
#33789=CARTESIAN_POINT('Ctrl Pts',(-9.06289743953882,1.76638731779995,0.927152330027173));
#33790=CARTESIAN_POINT('Ctrl Pts',(-8.95185791952612,0.180791550756394,
1.98671840348209));
#33791=CARTESIAN_POINT('Ctrl Pts',(-8.84081839951343,-1.57001661465857,
1.23076538351361));
#33792=CARTESIAN_POINT('Ctrl Pts',(-8.72977887950074,-1.88609948840221,
-0.649895621933452));
#33793=CARTESIAN_POINT('Ctrl Pts',(-8.61873935948805,-0.478611660183903,
-1.93666374941427));
#33794=CARTESIAN_POINT('Ctrl Pts',(-8.50769983947534,1.36624494957686,-1.45365413263095));
#33795=CARTESIAN_POINT('Ctrl Pts',(-8.39666031946266,1.96258854012834,0.357745470574083));
#33796=CARTESIAN_POINT('Ctrl Pts',(-8.28562079944997,0.765463584311097,
1.84222721200533));
#33797=CARTESIAN_POINT('Ctrl Pts',(-8.17458127943727,-1.13116350034402,
1.64322997022596));
#33798=CARTESIAN_POINT('Ctrl Pts',(-8.06354175942458,-1.99410159864917,
-0.0573969844518235));
#33799=CARTESIAN_POINT('Ctrl Pts',(-7.95250223941189,-1.03477363235835,
-1.70557296218463));
#33800=CARTESIAN_POINT('Ctrl Pts',(-7.84146271939919,0.87015955086961,-1.79514844945752));
#33801=CARTESIAN_POINT('Ctrl Pts',(-7.7304231993865,1.97991648961337,-0.244266849401202));
#33802=CARTESIAN_POINT('Ctrl Pts',(-7.61938367937381,1.2803701149249,1.52983266024965));
#33803=CARTESIAN_POINT('Ctrl Pts',(-7.50834415936111,-0.589214442437421,
1.90592810472549));
#33804=CARTESIAN_POINT('Ctrl Pts',(-7.39730463934842,-1.92035828847847,
0.540332900563502));
#33805=CARTESIAN_POINT('Ctrl Pts',(-7.28626511933573,-1.49662477855607,
-1.31903368864154));
#33806=CARTESIAN_POINT('Ctrl Pts',(-7.17522559932303,0.294766501283195,
-1.97303023526772));
#33807=CARTESIAN_POINT('Ctrl Pts',(-7.06418607931034,1.81679187086397,-0.8240163211502));
#33808=CARTESIAN_POINT('Ctrl Pts',(-6.95314655929765,1.6785817865682,1.07800685775223));
#33809=CARTESIAN_POINT('Ctrl Pts',(-6.84210703928495,0.00643650640064556,
1.99491708372672));
#33810=CARTESIAN_POINT('Ctrl Pts',(-6.73106751927226,-1.67159063414775,
1.0888160319305));
#33811=CARTESIAN_POINT('Ctrl Pts',(-6.62002799925957,-1.82207129032072,
-0.812275699838614));
#33812=CARTESIAN_POINT('Ctrl Pts',(-6.50898847924688,-0.307492010793712,
-1.97108707642695));
#33813=CARTESIAN_POINT('Ctrl Pts',(-6.39794895923418,1.48808210710229,-1.32866370541284));
#33814=CARTESIAN_POINT('Ctrl Pts',(-6.28690943922149,1.92380498825995,0.527929888058504));
#33815=CARTESIAN_POINT('Ctrl Pts',(-6.1758699192088,0.601500822359763,1.90208631777315));
#33816=CARTESIAN_POINT('Ctrl Pts',(-6.0648303991961,-1.27047169401729,1.53806283170103));
#33817=CARTESIAN_POINT('Ctrl Pts',(-5.95379087918341,-1.98145148283935,
-0.231485681442862));
#33818=CARTESIAN_POINT('Ctrl Pts',(-5.84275135917072,-0.881725238294048,
-1.78949607535603));
#33819=CARTESIAN_POINT('Ctrl Pts',(-5.73171183915802,1.0237463008388,-1.71221468019586));
#33820=CARTESIAN_POINT('Ctrl Pts',(-5.62067231914534,1.993689708387,-0.0702634060598052));
#33821=CARTESIAN_POINT('Ctrl Pts',(-5.50963279913263,1.14174344823272,1.63589654256526));
#33822=CARTESIAN_POINT('Ctrl Pts',(-5.39859327911995,-0.753560051892996,
1.84712827051895));
#33823=CARTESIAN_POINT('Ctrl Pts',(-5.28755375910725,-1.96023920553107,
0.370402290298364));
#33824=CARTESIAN_POINT('Ctrl Pts',(-5.17651423909456,-1.37559670075934,
-1.44480770915003));
#33825=CARTESIAN_POINT('Ctrl Pts',(-5.06547471908186,0.466104716187191,
-1.93971183249147));
#33826=CARTESIAN_POINT('Ctrl Pts',(-4.95443519906918,1.88186654839468,-0.662052787617739));
#33827=CARTESIAN_POINT('Ctrl Pts',(-4.84339567905647,1.57792585814243,1.22060869477682));
#33828=CARTESIAN_POINT('Ctrl Pts',(-4.73235615904379,-0.16796781268475,
1.98784365920996));
#33829=CARTESIAN_POINT('Ctrl Pts',(-4.62131663903109,-1.76036777726992,
0.938531239921795));
#33830=CARTESIAN_POINT('Ctrl Pts',(-4.5102771190184,-1.74409420992455,-0.968437394190764));
#33831=CARTESIAN_POINT('Ctrl Pts',(-4.39923759900571,-0.134018353690417,
-1.99042072950253));
#33832=CARTESIAN_POINT('Ctrl Pts',(-4.28819807899301,1.59852723935581,-1.19350168185761));
#33833=CARTESIAN_POINT('Ctrl Pts',(-4.17715855898033,1.87029373088395,0.694072733778989));
#33834=CARTESIAN_POINT('Ctrl Pts',(-4.06611903896762,0.432933265729,1.94738398550062));
#33835=CARTESIAN_POINT('Ctrl Pts',(-3.95507951895494,-1.40005378079356,
1.42112104004054));
#33836=CARTESIAN_POINT('Ctrl Pts',(-3.84403999894224,-1.95363234829038,
-0.403802237824197));
#33837=CARTESIAN_POINT('Ctrl Pts',(-3.73300047892955,-0.721926789142902,
-1.85971968604833));
#33838=CARTESIAN_POINT('Ctrl Pts',(-3.62196095891686,1.16949575226516,-1.61617303683714));
#33839=CARTESIAN_POINT('Ctrl Pts',(-3.51092143890416,1.99220021857957,0.104277939388565));
#33840=CARTESIAN_POINT('Ctrl Pts',(-3.39988191889147,0.99437615483157,1.72943680493244));
#33841=CARTESIAN_POINT('Ctrl Pts',(-3.28884239887877,-0.912136775947003,
1.77418773007997));
#33842=CARTESIAN_POINT('Ctrl Pts',(-3.17780287886609,-1.98511349460065,
0.197636062123149));
#33843=CARTESIAN_POINT('Ctrl Pts',(-3.06676335885339,-1.24403773070594,
-1.55952099188045));
#33844=CARTESIAN_POINT('Ctrl Pts',(-2.95572383884069,0.633874662509295,
-1.89154394928109));
#33845=CARTESIAN_POINT('Ctrl Pts',(-2.84468431882801,1.93253458040476,-0.495020903213892));
#33846=CARTESIAN_POINT('Ctrl Pts',(-2.73364479881531,1.46519010502714,1.35386615132057));
#33847=CARTESIAN_POINT('Ctrl Pts',(-2.62260527880262,-0.341086253099156,
1.96555228097401));
#33848=CARTESIAN_POINT('Ctrl Pts',(-2.51156575878993,-1.83566840917728,
0.781061513271475));
#33849=CARTESIAN_POINT('Ctrl Pts',(-2.40052623877724,-1.65276520269481,
-1.11718520642857));
#33850=CARTESIAN_POINT('Ctrl Pts',(-2.28948671876454,0.0404812844924485,
-1.99451670231561));
#33851=CARTESIAN_POINT('Ctrl Pts',(-2.17844719875185,1.69673482806298,-1.04920279100363));
#33852=CARTESIAN_POINT('Ctrl Pts',(-2.06740767873915,1.80246443268206,0.854902090273845));
#33853=CARTESIAN_POINT('Ctrl Pts',(-1.95636815872646,0.261051368054344,
1.97777345655945));
#33854=CARTESIAN_POINT('Ctrl Pts',(-1.84532863871377,-1.51891771206272,
1.29329980977728));
#33855=CARTESIAN_POINT('Ctrl Pts',(-1.73428911870107,-1.91085722520509,
-0.573027417365632));
#33856=CARTESIAN_POINT('Ctrl Pts',(-1.62324959868838,-0.556601508026538,
-1.91570632117762));
#33857=CARTESIAN_POINT('Ctrl Pts',(-1.51221007867569,1.30629189965073,-1.50775853036321));
#33858=CARTESIAN_POINT('Ctrl Pts',(-1.401170558663,1.97545984031888,0.278020533921918));
#33859=CARTESIAN_POINT('Ctrl Pts',(-1.2901310386503,0.83939561223033,1.80973820580727));
#33860=CARTESIAN_POINT('Ctrl Pts',(-1.17909151863761,-1.06372911823659,
1.68766325019619));
#33861=CARTESIAN_POINT('Ctrl Pts',(-1.06805199862492,-1.99479360520537,
0.0233599311130506));
#33862=CARTESIAN_POINT('Ctrl Pts',(-0.957012478612224,-1.10294954911385,
-1.66230125013214));
#33863=CARTESIAN_POINT('Ctrl Pts',(-0.845972958599527,0.796781567798704,
-1.82888410563971));
#33864=CARTESIAN_POINT('Ctrl Pts',(-0.734933438586838,1.96842788148691,
-0.324220749111252));
#33865=CARTESIAN_POINT('Ctrl Pts',(-0.623893918574146,1.34119989429253,
1.47679973039398));
#33866=CARTESIAN_POINT('Ctrl Pts',(-0.51285439856145,-0.511521802863037,
1.92813623824627));
#33867=CARTESIAN_POINT('Ctrl Pts',(-0.401814878548755,-1.89705251590108,
0.61775959459427));
#33868=CARTESIAN_POINT('Ctrl Pts',(-0.290775358536067,-1.54852363859167,
-1.2576608046069));
#33869=CARTESIAN_POINT('Ctrl Pts',(-0.17973583852337,0.214175227446937,
-1.98280781972719));
#33870=CARTESIAN_POINT('Ctrl Pts',(-0.0686963185106793,1.78290898567335,
-0.897910809498253));
#33871=CARTESIAN_POINT('Ctrl Pts',(0.0423432015020128,1.71890913368323,
1.01133117883693));
#33872=CARTESIAN_POINT('Ctrl Pts',(0.116369548177145,0.634152313505382,
1.66221084604168));
#33873=CARTESIAN_POINT('Ctrl Pts',(0.15338272151471,0.0737739821678063,
1.68672073681435));
#33874=CARTESIAN_POINT('Ctrl Pts',(-19.646,0.903606778650211,-1.26612599672283));
#33875=CARTESIAN_POINT('Ctrl Pts',(-19.6089868266624,1.32425114367218,-0.965921198291487));
#33876=CARTESIAN_POINT('Ctrl Pts',(-19.5349604799873,1.83563729847737,0.081414173630813));
#33877=CARTESIAN_POINT('Ctrl Pts',(-19.4239209599746,0.926784913186551,
1.58861167214729));
#33878=CARTESIAN_POINT('Ctrl Pts',(-19.3128814399619,-0.829751980945401,
1.63941117334604));
#33879=CARTESIAN_POINT('Ctrl Pts',(-19.2018419199493,-1.82763728486514,
0.194420247730427));
#33880=CARTESIAN_POINT('Ctrl Pts',(-19.0908023999365,-1.15558706114236,
-1.42945935470984));
#33881=CARTESIAN_POINT('Ctrl Pts',(-18.9797628799239,0.572581864613586,
-1.74641810285352));
#33882=CARTESIAN_POINT('Ctrl Pts',(-18.8687233599111,1.7774511739937,-0.467787493561026));
#33883=CARTESIAN_POINT('Ctrl Pts',(-18.7576838398985,1.35806626263998,1.23849733645003));
#33884=CARTESIAN_POINT('Ctrl Pts',(-18.6466443198858,-0.302373835599965,
1.81291555390549));
#33885=CARTESIAN_POINT('Ctrl Pts',(-18.5356047998731,-1.68648777596589,
0.730689455758268));
#33886=CARTESIAN_POINT('Ctrl Pts',(-18.4245652798604,-1.52944624713167,
-1.0192868695147));
#33887=CARTESIAN_POINT('Ctrl Pts',(-18.3135257598477,0.0252485661867687,
-1.83779672371819));
#33888=CARTESIAN_POINT('Ctrl Pts',(-18.202486239835,1.5568693034731,-0.976883390785028));
#33889=CARTESIAN_POINT('Ctrl Pts',(-18.0914467198223,1.66577977622518,0.776737156863176));
#33890=CARTESIAN_POINT('Ctrl Pts',(-17.9804071998096,0.252453550943756,
1.820551509628));
#33891=CARTESIAN_POINT('Ctrl Pts',(-17.8693676797969,-1.39157164370297,
1.20069577440679));
#33892=CARTESIAN_POINT('Ctrl Pts',(-17.7583281597842,-1.76393966810407,
-0.516390033712223));
#33893=CARTESIAN_POINT('Ctrl Pts',(-17.6472886397715,-0.524370017185474,
-1.76158383684904));
#33894=CARTESIAN_POINT('Ctrl Pts',(-17.5362491197588,1.19438366161834,-1.39699298808207));
#33895=CARTESIAN_POINT('Ctrl Pts',(-17.4252095997461,1.821676008134,0.244209379874806));
#33896=CARTESIAN_POINT('Ctrl Pts',(-17.3141700797334,0.784269631776072,
1.66224631422945));
#33897=CARTESIAN_POINT('Ctrl Pts',(-17.2031305597208,-0.96982436419101,
1.56127588796884));
#33898=CARTESIAN_POINT('Ctrl Pts',(-17.0920910397081,-1.83766561117703,
0.0335676802536325));
#33899=CARTESIAN_POINT('Ctrl Pts',(-16.9810515196953,-1.02619639290964,
-1.5248156107606));
#33900=CARTESIAN_POINT('Ctrl Pts',(-16.8700119996827,0.723039919366596,
-1.68977956052457));
#33901=CARTESIAN_POINT('Ctrl Pts',(-16.7589724796699,1.81154203999908,-0.310575472322002));
#33902=CARTESIAN_POINT('Ctrl Pts',(-16.6479329596573,1.24460614954145,1.35244120715334));
#33903=CARTESIAN_POINT('Ctrl Pts',(-16.5368934396446,-0.459685807164506,
1.77955911551557));
#33904=CARTESIAN_POINT('Ctrl Pts',(-16.4258539196319,-1.74390395857547,
0.58046590764267));
#33905=CARTESIAN_POINT('Ctrl Pts',(-16.3148143996192,-1.43449367810364,
-1.14907335454206));
#33906=CARTESIAN_POINT('Ctrl Pts',(-16.2037748796065,0.185797227123519,
-1.82855710250446));
#33907=CARTESIAN_POINT('Ctrl Pts',(-16.0927353595938,1.63630140628791,-0.837053997341315));
#33908=CARTESIAN_POINT('Ctrl Pts',(-15.9816958395811,1.59150738893344,0.919372567381872));
#33909=CARTESIAN_POINT('Ctrl Pts',(-15.8706563195684,0.0923492065994037,
1.83565065051508));
#33910=CARTESIAN_POINT('Ctrl Pts',(-15.7596167995557,-1.49120027525227,
1.07445959708913));
#33911=CARTESIAN_POINT('Ctrl Pts',(-15.648577279543,-1.7120490507056,-0.668602822808828));
#33912=CARTESIAN_POINT('Ctrl Pts',(-15.5375377595304,-0.368379304064812,
-1.80067719900824));
#33913=CARTESIAN_POINT('Ctrl Pts',(-15.4264982395177,1.31192580014841,-1.28724216120951));
#33914=CARTESIAN_POINT('Ctrl Pts',(-15.315458719505,1.79335624998195,0.402510928225848));
#33915=CARTESIAN_POINT('Ctrl Pts',(-15.2044191994923,0.635967374718456,
1.72443822301191));
#33916=CARTESIAN_POINT('Ctrl Pts',(-15.0933796794796,-1.10258635489586,
1.47052542197953));
#33917=CARTESIAN_POINT('Ctrl Pts',(-14.9823401594669,-1.83356569653797,
-0.127194823675595));
#33918=CARTESIAN_POINT('Ctrl Pts',(-14.8713006394542,-0.888981191146498,
-1.60868086595148));
#33919=CARTESIAN_POINT('Ctrl Pts',(-14.7602611194415,0.867979302403128,
-1.62010913746279));
#33920=CARTESIAN_POINT('Ctrl Pts',(-14.6492215994288,1.83175592377073,-0.151036162628272));
#33921=CARTESIAN_POINT('Ctrl Pts',(-14.5381820794161,1.12162251930453,1.4560579009365));
#33922=CARTESIAN_POINT('Ctrl Pts',(-14.4271425594034,-0.613481054986446,
1.73256534706872));
#33923=CARTESIAN_POINT('Ctrl Pts',(-14.3161030393907,-1.78796840564486,
0.425805903090126));
#33924=CARTESIAN_POINT('Ctrl Pts',(-14.205063519378,-1.32855999473149,-1.27006693803504));
#33925=CARTESIAN_POINT('Ctrl Pts',(-14.0940239993653,0.344923864904767,
-1.8053169289933));
#33926=CARTESIAN_POINT('Ctrl Pts',(-13.9829844793526,1.70320660624744,-0.690817590341849));
#33927=CARTESIAN_POINT('Ctrl Pts',(-13.8719449593399,1.50505129966774,1.05497027069917));
#33928=CARTESIAN_POINT('Ctrl Pts',(-13.7609054393273,-0.0684621685615409,
1.83669665926807));
#33929=CARTESIAN_POINT('Ctrl Pts',(-13.6498659193145,-1.57941298373299,
0.939998039097045));
#33930=CARTESIAN_POINT('Ctrl Pts',(-13.5388263993019,-1.64705184118444,
-0.815697198194015));
#33931=CARTESIAN_POINT('Ctrl Pts',(-13.4277868792892,-0.209568452681189,
-1.82598541898106));
#33932=CARTESIAN_POINT('Ctrl Pts',(-13.3167473592765,1.4194244756517,-1.1676368633319));
#33933=CARTESIAN_POINT('Ctrl Pts',(-13.2057078392638,1.75130743978355,0.557731062474938));
#33934=CARTESIAN_POINT('Ctrl Pts',(-13.0946683192511,0.482796462927691,
1.77342867408733));
#33935=CARTESIAN_POINT('Ctrl Pts',(-12.9836287992384,-1.22690748578881,
1.36851733931507));
#33936=CARTESIAN_POINT('Ctrl Pts',(-12.8725892792257,-1.81542890435427,
-0.286983588251427));
#33937=CARTESIAN_POINT('Ctrl Pts',(-12.761549759213,-0.744960386131938,
-1.68023085014673));
#33938=CARTESIAN_POINT('Ctrl Pts',(-12.6505102392003,1.00627386240032,-1.53803595554219));
#33939=CARTESIAN_POINT('Ctrl Pts',(-12.5394707191877,1.83794678447648,0.00965940594506788));
#33940=CARTESIAN_POINT('Ctrl Pts',(-12.4284311991749,0.990052298275348,
1.5485277309013));
#33941=CARTESIAN_POINT('Ctrl Pts',(-12.3173916791622,-0.762579793343959,
1.67230790988804));
#33942=CARTESIAN_POINT('Ctrl Pts',(-12.2063521591496,-1.8183450453305,0.267886137776231));
#33943=CARTESIAN_POINT('Ctrl Pts',(-12.0953126391368,-1.21245550897696,
-1.3813375132248));
#33944=CARTESIAN_POINT('Ctrl Pts',(-11.9842731191242,0.501409935092548,
-1.76825613633351));
#33945=CARTESIAN_POINT('Ctrl Pts',(-11.8732335991115,1.75707289349663,-0.539292623378071));
#33946=CARTESIAN_POINT('Ctrl Pts',(-11.7621940790988,1.40707327733112,1.18249164010207));
#33947=CARTESIAN_POINT('Ctrl Pts',(-11.6511545590861,-0.228749431006459,
1.82368182107101));
#33948=CARTESIAN_POINT('Ctrl Pts',(-11.5401150390734,-1.65553448263634,
0.798340318092896));
#33949=CARTESIAN_POINT('Ctrl Pts',(-11.4290755190607,-1.56944561223521,
-0.956546996715934));
#33950=CARTESIAN_POINT('Ctrl Pts',(-11.318035999048,-0.0491532482193918,
-1.83731479199404));
#33951=CARTESIAN_POINT('Ctrl Pts',(-11.2069964790353,1.51605673496666,-1.03909271148097));
#33952=CARTESIAN_POINT('Ctrl Pts',(-11.0959569590226,1.69585148053222,0.708681481814863));
#33953=CARTESIAN_POINT('Ctrl Pts',(-10.9849174390099,0.325929498694267,
1.80884262681183));
#33954=CARTESIAN_POINT('Ctrl Pts',(-10.8738779189972,-1.34183601595248,
1.25603256047899));
#33955=CARTESIAN_POINT('Ctrl Pts',(-10.7628383989846,-1.78339408069835,
-0.444575347517961));
#33956=CARTESIAN_POINT('Ctrl Pts',(-10.6517988789718,-0.595236530522984,
-1.73891781272768));
#33957=CARTESIAN_POINT('Ctrl Pts',(-10.5407593589592,1.1368648842552,-1.44418832623659));
#33958=CARTESIAN_POINT('Ctrl Pts',(-10.4297198389465,1.83006722788652,0.170281026853745));
#33959=CARTESIAN_POINT('Ctrl Pts',(-10.3186803189338,0.850902723426497,
1.62914279360528));
#33960=CARTESIAN_POINT('Ctrl Pts',(-10.2076407989211,-0.905840595584799,
1.59924810522983));
#33961=CARTESIAN_POINT('Ctrl Pts',(-10.0966012789084,-1.83480132900177,
0.107915567848148));
#33962=CARTESIAN_POINT('Ctrl Pts',(-9.98556175889571,-1.08706905972496,
-1.48203324729215));
#33963=CARTESIAN_POINT('Ctrl Pts',(-9.874522238883,0.654057457242615,-1.71765844372971));
#33964=CARTESIAN_POINT('Ctrl Pts',(-9.76348271887031,1.79748789421279,-0.38363909713309));
#33965=CARTESIAN_POINT('Ctrl Pts',(-9.65244319885762,1.29832339351032,1.30096043466144));
#33966=CARTESIAN_POINT('Ctrl Pts',(-9.54140367884492,-0.387285500229918,
1.79670577112734));
#33967=CARTESIAN_POINT('Ctrl Pts',(-9.43036415883223,-1.71898202317764,
0.65057089596963));
#33968=CARTESIAN_POINT('Ctrl Pts',(-9.31932463881954,-1.47982447900607,
-1.09007394154023));
#33969=CARTESIAN_POINT('Ctrl Pts',(-9.20828511880685,0.111638249353674,
-1.83457858593517));
#33970=CARTESIAN_POINT('Ctrl Pts',(-9.09724559879415,1.60108280900731,-0.902593776508504));
#33971=CARTESIAN_POINT('Ctrl Pts',(-8.98620607878146,1.62741291579734,0.854206584022058));
#33972=CARTESIAN_POINT('Ctrl Pts',(-8.87516655876877,0.166567378401736,
1.83040896936805));
#33973=CARTESIAN_POINT('Ctrl Pts',(-8.76412703875608,-1.44649210904326,
1.13393221365574));
#33974=CARTESIAN_POINT('Ctrl Pts',(-8.65308751874338,-1.73770646843612,
-0.598763656417053));
#33975=CARTESIAN_POINT('Ctrl Pts',(-8.5420479987307,-0.44095583657419,-1.78429247515137));
#33976=CARTESIAN_POINT('Ctrl Pts',(-8.43100847871798,1.25875262728536,-1.33928470087313));
#33977=CARTESIAN_POINT('Ctrl Pts',(-8.31996895870532,1.8081775760136,0.329599059907972));
#33978=CARTESIAN_POINT('Ctrl Pts',(-8.2089294386926,0.705239055515858,1.69728593974785));
#33979=CARTESIAN_POINT('Ctrl Pts',(-8.09788991867992,-1.04216672741466,
1.51394524305222));
#33980=CARTESIAN_POINT('Ctrl Pts',(-7.98685039866723,-1.83721127543857,
-0.0528811506306726));
#33981=CARTESIAN_POINT('Ctrl Pts',(-7.87581087865453,-0.953360544007956,
-1.57138326318549));
#33982=CARTESIAN_POINT('Ctrl Pts',(-7.76477135864184,0.80169783694629,-1.65391120224947));
#33983=CARTESIAN_POINT('Ctrl Pts',(-7.65373183862914,1.82414221101299,-0.225048618505586));
#33984=CARTESIAN_POINT('Ctrl Pts',(-7.54269231861645,1.17963418386913,1.40946971550936));
#33985=CARTESIAN_POINT('Ctrl Pts',(-7.43165279860376,-0.54285670200082,
1.75597502481768));
#33986=CARTESIAN_POINT('Ctrl Pts',(-7.32061327859107,-1.76926988216876,
0.49782102279954));
#33987=CARTESIAN_POINT('Ctrl Pts',(-7.20957375857836,-1.37887453684738,
-1.21525581600112));
#33988=CARTESIAN_POINT('Ctrl Pts',(-7.09853423856569,0.271575099355961,
-1.81779774785327));
#33989=CARTESIAN_POINT('Ctrl Pts',(-6.98749471855298,1.67385177993814,-0.75918502717621));
#33990=CARTESIAN_POINT('Ctrl Pts',(-6.8764551985403,1.54651567759537,0.993192300434498));
#33991=CARTESIAN_POINT('Ctrl Pts',(-6.7654156785276,0.00593010012215213,
1.83796260043647));
#33992=CARTESIAN_POINT('Ctrl Pts',(-6.65437615851491,-1.54007456944727,
1.00315103909255));
#33993=CARTESIAN_POINT('Ctrl Pts',(-6.54333663850221,-1.67871582947318,
-0.748368125033921));
#33994=CARTESIAN_POINT('Ctrl Pts',(-6.43229711848952,-0.283299401454877,
-1.81600747130234));
#33995=CARTESIAN_POINT('Ctrl Pts',(-6.32125759847683,1.37100397883372,-1.22412817005115));
#33996=CARTESIAN_POINT('Ctrl Pts',(-6.21021807846413,1.77244540527444,0.486393844545889));
#33997=CARTESIAN_POINT('Ctrl Pts',(-6.09917855845144,0.55417642399643,1.75243549889208));
#33998=CARTESIAN_POINT('Ctrl Pts',(-5.98813903843875,-1.17051454296774,
1.4170523601447));
#33999=CARTESIAN_POINT('Ctrl Pts',(-5.87709951842606,-1.82555643527539,
-0.213273037009483));
#34000=CARTESIAN_POINT('Ctrl Pts',(-5.76605999841336,-0.812353568509229,
-1.64870354109554));
#34001=CARTESIAN_POINT('Ctrl Pts',(-5.65502047840067,0.943200812016622,
-1.57750242944403));
#34002=CARTESIAN_POINT('Ctrl Pts',(-5.54398095838797,1.83683179154747,-0.0647352782582765));
#34003=CARTESIAN_POINT('Ctrl Pts',(-5.43294143837528,1.05191427466497,1.50718878892018));
#34004=CARTESIAN_POINT('Ctrl Pts',(-5.32190191836259,-0.694272059656186,
1.70180139671801));
#34005=CARTESIAN_POINT('Ctrl Pts',(-5.2108623983499,-1.80601308047596,0.341260076540456));
#34006=CARTESIAN_POINT('Ctrl Pts',(-5.0998228783372,-1.26736860890297,-1.33113428919024));
#34007=CARTESIAN_POINT('Ctrl Pts',(-4.98878335832452,0.429432903867215,
-1.78710074359752));
#34008=CARTESIAN_POINT('Ctrl Pts',(-4.87774383831181,1.73380656428109,-0.6099643303886));
#34009=CARTESIAN_POINT('Ctrl Pts',(-4.76670431829913,1.45377907542383,1.12457462471391));
#34010=CARTESIAN_POINT('Ctrl Pts',(-4.65566479828643,-0.154752576089497,
1.83144569312997));
#34011=CARTESIAN_POINT('Ctrl Pts',(-4.54462527827374,-1.62186697584008,
0.864690233187587));
#34012=CARTESIAN_POINT('Ctrl Pts',(-4.43358575826105,-1.60687376714965,
-0.892243455082156));
#34013=CARTESIAN_POINT('Ctrl Pts',(-4.32254623824836,-0.123474165349735,
-1.83382000675687));
#34014=CARTESIAN_POINT('Ctrl Pts',(-4.21150671823566,1.4727595977204,-1.09960031557524));
#34015=CARTESIAN_POINT('Ctrl Pts',(-4.10046719822297,1.72314426360711,0.639465036955492));
#34016=CARTESIAN_POINT('Ctrl Pts',(-3.98942767821027,0.398871290133161,
1.79416927311721));
#34017=CARTESIAN_POINT('Ctrl Pts',(-3.87838815819758,-1.28990147444681,
1.30931122079946));
#34018=CARTESIAN_POINT('Ctrl Pts',(-3.76734863818489,-1.79992603224029,
-0.372032209833472));
#34019=CARTESIAN_POINT('Ctrl Pts',(-3.6563091181722,-0.665127613333747,
-1.71340215497423));
#34020=CARTESIAN_POINT('Ctrl Pts',(-3.5452695981595,1.07748310522118,-1.48901707332687));
#34021=CARTESIAN_POINT('Ctrl Pts',(-3.43423007814681,1.83545949062223,0.0960736434662692));
#34022=CARTESIAN_POINT('Ctrl Pts',(-3.32319055813411,0.916141426756487,
1.59336956568948));
#34023=CARTESIAN_POINT('Ctrl Pts',(-3.21215103812143,-0.840372411640004,
1.63459961350804));
#34024=CARTESIAN_POINT('Ctrl Pts',(-3.10111151810872,-1.82893033021795,
0.18208661083865));
#34025=CARTESIAN_POINT('Ctrl Pts',(-2.99007199809604,-1.14616032978072,
-1.43682225244029));
#34026=CARTESIAN_POINT('Ctrl Pts',(-2.87903247808334,0.584003181164767,
-1.74272257439688));
#34027=CARTESIAN_POINT('Ctrl Pts',(-2.76799295807065,1.78048817758317,-0.456074046366774));
#34028=CARTESIAN_POINT('Ctrl Pts',(-2.65695343805795,1.34991305530291,1.24734775817125));
#34029=CARTESIAN_POINT('Ctrl Pts',(-2.54591391804527,-0.314250542958959,
1.81090813803855));
#34030=CARTESIAN_POINT('Ctrl Pts',(-2.43487439803257,-1.69124316513835,
0.719609783155264));
#34031=CARTESIAN_POINT('Ctrl Pts',(-2.32383487801988,-1.52273027016296,
-1.02928820647559));
#34032=CARTESIAN_POINT('Ctrl Pts',(-2.21279535800718,0.0372963305200237,
-1.8375937199123));
#34033=CARTESIAN_POINT('Ctrl Pts',(-2.10175583799449,1.56324048867835,-0.966654456903947));
#34034=CARTESIAN_POINT('Ctrl Pts',(-1.9907163179818,1.66065158442465,0.787640790575088));
#34035=CARTESIAN_POINT('Ctrl Pts',(-1.87967679796911,0.2405125782874,1.82216778579164));
#34036=CARTESIAN_POINT('Ctrl Pts',(-1.76863727795641,-1.39941352484514,
1.19154660657962));
#34037=CARTESIAN_POINT('Ctrl Pts',(-1.65759775794372,-1.760516335917,-0.527943226680482));
#34038=CARTESIAN_POINT('Ctrl Pts',(-1.54655823793103,-0.512809661837298,
-1.76498391861309));
#34039=CARTESIAN_POINT('Ctrl Pts',(-1.43551871791833,1.20351651524581,-1.3891323162764));
#34040=CARTESIAN_POINT('Ctrl Pts',(-1.32447919790564,1.82003619839053,0.256146657758448));
#34041=CARTESIAN_POINT('Ctrl Pts',(-1.21343967789295,0.77335431875082,1.66735307747278));
#34042=CARTESIAN_POINT('Ctrl Pts',(-1.10240015788025,-0.980037893435529,
1.55488263712548));
#34043=CARTESIAN_POINT('Ctrl Pts',(-0.991360637867559,-1.837848836859,0.0215220372239174));
#34044=CARTESIAN_POINT('Ctrl Pts',(-0.88032111785487,-1.01617257076799,
-1.53151604812273));
#34045=CARTESIAN_POINT('Ctrl Pts',(-0.769281597842172,0.734093027864279,
-1.68499263158297));
#34046=CARTESIAN_POINT('Ctrl Pts',(-0.658242077829484,1.81355749436498,
-0.29871196954151));
#34047=CARTESIAN_POINT('Ctrl Pts',(-0.547202557816791,1.23567804673567,
1.36060926789406));
#34048=CARTESIAN_POINT('Ctrl Pts',(-0.436163037804095,-0.47127670149265,
1.77643588465474));
#34049=CARTESIAN_POINT('Ctrl Pts',(-0.3251235177914,-1.74779774243877,0.569156001613867));
#34050=CARTESIAN_POINT('Ctrl Pts',(-0.214083997778712,-1.42669014007662,
-1.15871157842014));
#34051=CARTESIAN_POINT('Ctrl Pts',(-0.103044477766015,0.197324521003166,
-1.82680605937946));
#34052=CARTESIAN_POINT('Ctrl Pts',(0.00799504224667571,1.64263470516183,
-0.827265704348207));
#34053=CARTESIAN_POINT('Ctrl Pts',(0.119034562259368,1.58367018209927,0.931762477007397));
#34054=CARTESIAN_POINT('Ctrl Pts',(0.1930609089345,0.584258987358921,1.53143275677265));
#34055=CARTESIAN_POINT('Ctrl Pts',(0.230074082272065,0.0679696520801858,
1.55401427805413));
#34056=CARTESIAN_POINT('',(0.,0.0853826423430472,1.95213365433479));
#34057=CARTESIAN_POINT('Ctrl Pts',(2.77555756156289E-17,1.33819577673882,
-0.797970124357286));
#34058=CARTESIAN_POINT('Ctrl Pts',(1.85767714458696E-16,1.36144302530136,
-0.768447784071024));
#34059=CARTESIAN_POINT('Ctrl Pts',(4.34722244779448E-15,1.38350431609264,
-0.738083050538838));
#34060=CARTESIAN_POINT('Ctrl Pts',(3.30291349825984E-15,1.40431382449103,
-0.706922234106086));
#34061=CARTESIAN_POINT('Ctrl Pts',(1.64949265289499E-15,1.43726085131009,
-0.657586313475071));
#34062=CARTESIAN_POINT('Ctrl Pts',(-1.84250246973165E-15,1.46707229630311,
-0.606256863967469));
#34063=CARTESIAN_POINT('Ctrl Pts',(-1.2490009027033E-15,1.49380501049835,
-0.553258599699532));
#34064=CARTESIAN_POINT('Ctrl Pts',(-9.0035866934265E-16,1.50950868121903,
-0.522125685744261));
#34065=CARTESIAN_POINT('Ctrl Pts',(-6.10224942617705E-15,1.52414930935612,
-0.49041610674948));
#34066=CARTESIAN_POINT('Ctrl Pts',(-5.71764857681956E-15,1.53773259716531,
-0.458190051451294));
#34067=CARTESIAN_POINT('Ctrl Pts',(-5.5403078360827E-15,1.54399589670235,
-0.443330509338595));
#34068=CARTESIAN_POINT('Ctrl Pts',(1.3347825398265E-15,1.55003513608504,
-0.428358552453907));
#34069=CARTESIAN_POINT('Ctrl Pts',(1.11022302462516E-15,1.55584236110343,
-0.413302430982821));
#34070=CARTESIAN_POINT('Ctrl Pts',(2.43036775803427E-16,1.57826824528491,
-0.355159886951195));
#34071=CARTESIAN_POINT('Ctrl Pts',(3.22432105167343E-16,1.59726695275495,
-0.295698115059786));
#34072=CARTESIAN_POINT('Ctrl Pts',(1.66533453693773E-16,1.61289818059431,
-0.235272160005541));
#34073=CARTESIAN_POINT('Ctrl Pts',(4.64879345376463E-17,1.62493458272665,
-0.188742795726714));
#34074=CARTESIAN_POINT('Ctrl Pts',(4.60117079108609E-15,1.63497355098178,
-0.141640714047145));
#34075=CARTESIAN_POINT('Ctrl Pts',(6.02295990859147E-15,1.64302567919564,
-0.0941152689092269));
#34076=CARTESIAN_POINT('Ctrl Pts',(6.50794676775413E-15,1.64577234276476,
-0.0779038518404372));
#34077=CARTESIAN_POINT('Ctrl Pts',(-2.48752701466179E-15,1.6482876960855,
-0.0616430990017152));
#34078=CARTESIAN_POINT('Ctrl Pts',(-2.22044604925031E-15,1.65057175197968,
-0.0453387342717473));
#34079=CARTESIAN_POINT('Ctrl Pts',(-1.95995858369583E-15,1.65279942076971,
-0.0294368797931177));
#34080=CARTESIAN_POINT('Ctrl Pts',(2.01657362464638E-16,1.65480738528587,
-0.0134894297485523));
#34081=CARTESIAN_POINT('Ctrl Pts',(1.66533453693773E-16,1.65659278118466,
0.00247052324260472));
#34082=CARTESIAN_POINT('Ctrl Pts',(2.50013631112385E-17,1.66378704921789,
0.0667812902239603));
#34083=CARTESIAN_POINT('Ctrl Pts',(2.78729284858849E-15,1.66738409972544,
0.131373953612928));
#34084=CARTESIAN_POINT('Ctrl Pts',(2.22044604925031E-15,1.66744264184217,
0.19588728583938));
#34085=CARTESIAN_POINT('Ctrl Pts',(1.64177178678514E-15,1.6675024054613,
0.261746712035136));
#34086=CARTESIAN_POINT('Ctrl Pts',(2.74120336787342E-15,1.6638748341243,
0.327524480561884));
#34087=CARTESIAN_POINT('Ctrl Pts',(1.85962356624714E-15,1.65657462015792,
0.392860803376907));
#34088=CARTESIAN_POINT('Ctrl Pts',(1.27711720799663E-15,1.65175098304174,
0.43603196427947));
#34089=CARTESIAN_POINT('Ctrl Pts',(-9.10818389979693E-16,1.64532289717713,
0.479010876745845));
#34090=CARTESIAN_POINT('Ctrl Pts',(-5.55111512312578E-16,1.63728231888051,
0.521695995682809));
#34091=CARTESIAN_POINT('Ctrl Pts',(-3.80822141106348E-16,1.63334259372073,
0.542610864094066));
#34092=CARTESIAN_POINT('Ctrl Pts',(-3.4150718129913E-15,1.62901558792228,
0.56345520655164));
#34093=CARTESIAN_POINT('Ctrl Pts',(-3.71924713249427E-15,1.62429946022137,
0.584217038477149));
#34094=CARTESIAN_POINT('Ctrl Pts',(-3.90626465249348E-15,1.62139982159171,
0.596982131725653));
#34095=CARTESIAN_POINT('Ctrl Pts',(3.41061712681253E-15,1.61835307480705,
0.609716033053302));
#34096=CARTESIAN_POINT('Ctrl Pts',(3.71924713249427E-15,1.61515867855561,
0.622415937599459));
#34097=CARTESIAN_POINT('Ctrl Pts',(3.9772647208833E-15,1.61248813323602,
0.633033177282724));
#34098=CARTESIAN_POINT('Ctrl Pts',(-2.16347027594684E-15,1.60971491624366,
0.643624280439148));
#34099=CARTESIAN_POINT('Ctrl Pts',(-2.16493489801906E-15,1.60684190188332,
0.654177060515785));
#34100=CARTESIAN_POINT('Ctrl Pts',(-2.17400880471352E-15,1.58904245400387,
0.719555661315922));
#34101=CARTESIAN_POINT('Ctrl Pts',(-2.56174063694999E-15,1.56738808989198,
0.783577323980778));
#34102=CARTESIAN_POINT('Ctrl Pts',(-2.23432383705813E-15,1.5419084220951,
0.845867575772783));
#34103=CARTESIAN_POINT('Ctrl Pts',(-2.15110675602605E-15,1.53543244535713,
0.861699423535622));
#34104=CARTESIAN_POINT('Ctrl Pts',(1.01114729712598E-15,1.52870910174203,
0.87741947571057));
#34105=CARTESIAN_POINT('Ctrl Pts',(9.43689570931383E-16,1.52173834456087,
0.893021649046084));
#34106=CARTESIAN_POINT('Ctrl Pts',(7.03007412007331E-16,1.49528259824579,
0.952235752908995));
#34107=CARTESIAN_POINT('Ctrl Pts',(-1.51979766192264E-15,1.46526720058678,
1.00975289709403));
#34108=CARTESIAN_POINT('Ctrl Pts',(-3.33066907387547E-16,1.43198511538068,
1.06544449418259));
#34109=CARTESIAN_POINT('Ctrl Pts',(3.10283512530559E-16,1.41394223293977,
1.09563602013396));
#34110=CARTESIAN_POINT('Ctrl Pts',(5.3238620172534E-15,1.39493838269964,
1.12529083901457));
#34111=CARTESIAN_POINT('Ctrl Pts',(5.59274848654923E-15,1.37501431840528,
1.1543865469354));
#34112=CARTESIAN_POINT('Ctrl Pts',(5.79604585589064E-15,1.35995030321613,
1.17638497956356));
#34113=CARTESIAN_POINT('Ctrl Pts',(3.98761921311371E-15,1.34436016743568,
1.19806377318932));
#34114=CARTESIAN_POINT('Ctrl Pts',(4.63518112781003E-15,1.32826011938545,
1.21941254397355));
#34115=CARTESIAN_POINT('Ctrl Pts',(5.00670657023675E-15,1.31902304515486,
1.23166096583232));
#34116=CARTESIAN_POINT('Ctrl Pts',(-2.81519590396613E-15,1.30961522599116,
1.24380414149294));
#34117=CARTESIAN_POINT('Ctrl Pts',(-2.76167977375508E-15,1.30005809876754,
1.25581735673097));
#34118=CARTESIAN_POINT('Ctrl Pts',(-2.52523500380136E-15,1.2578328343679,
1.3088941001756));
#34119=CARTESIAN_POINT('Ctrl Pts',(-4.17224765824516E-15,1.21263786762318,
1.35951742488655));
#34120=CARTESIAN_POINT('Ctrl Pts',(-2.99760216648792E-15,1.16481156614242,
1.40755648980915));
#34121=CARTESIAN_POINT('Ctrl Pts',(-1.7982525475441E-15,1.1159794232883,
1.45660587076164));
#34122=CARTESIAN_POINT('Ctrl Pts',(-2.21069601816558E-18,1.06440359303693,
1.50296188609699));
#34123=CARTESIAN_POINT('Ctrl Pts',(-6.73072708679001E-16,1.01039246439479,
1.54646595937401));
#34124=CARTESIAN_POINT('Ctrl Pts',(-1.3489991402192E-15,0.955973599177281,
1.59029845018829));
#34125=CARTESIAN_POINT('Ctrl Pts',(-1.1547791066913E-16,0.899081837248503,
1.63123654739737));
#34126=CARTESIAN_POINT('Ctrl Pts',(1.33226762955019E-15,0.839989874352363,
1.66908726954678));
#34127=CARTESIAN_POINT('Ctrl Pts',(1.69882738300955E-15,0.825028173729644,
1.67867082618288));
#34128=CARTESIAN_POINT('Ctrl Pts',(-5.43398623855677E-16,0.809925242478508,
1.68805627460793));
#34129=CARTESIAN_POINT('Ctrl Pts',(-7.21644966006352E-16,0.79468516045783,
1.69724007942585));
#34130=CARTESIAN_POINT('Ctrl Pts',(-8.49633924018289E-16,0.783742090354353,
1.70383446781581));
#34131=CARTESIAN_POINT('Ctrl Pts',(7.66742462836056E-16,0.772727015708312,
1.71032552223986));
#34132=CARTESIAN_POINT('Ctrl Pts',(6.93889390390723E-16,0.761657574914039,
1.71670288403641));
#34133=CARTESIAN_POINT('Ctrl Pts',(2.82215011875755E-16,0.69910695067084,
1.7527397506508));
#34134=CARTESIAN_POINT('Ctrl Pts',(-3.781339996231E-15,0.634711960700427,
1.78521757183589));
#34135=CARTESIAN_POINT('Ctrl Pts',(-4.03843625207401E-15,0.568806275526336,
1.81397636836835));
#34136=CARTESIAN_POINT('Ctrl Pts',(-4.29614369899938E-15,0.502743913752955,
1.84280353275751));
#34137=CARTESIAN_POINT('Ctrl Pts',(-1.97887160151066E-15,0.435162865154654,
1.86789472013933));
#34138=CARTESIAN_POINT('Ctrl Pts',(-2.9767854847762E-15,0.366360222072395,
1.88905407399748));
#34139=CARTESIAN_POINT('Ctrl Pts',(-3.9534463475613E-15,0.299022899802941,
1.90976278758652));
#34140=CARTESIAN_POINT('Ctrl Pts',(2.03258476747404E-15,0.230514597231587,
1.92670591644718));
#34141=CARTESIAN_POINT('Ctrl Pts',(2.71224015468974E-15,0.161089063758093,
1.93965721286968));
#34142=CARTESIAN_POINT('Ctrl Pts',(2.95814837249331E-15,0.13596999676082,
1.94434316148629));
#34143=CARTESIAN_POINT('Ctrl Pts',(3.98524470648727E-17,0.110730680189629,
1.94850609293125));
#34144=CARTESIAN_POINT('Ctrl Pts',(-1.38777878078145E-17,0.0853826423430475,
1.95213365433479));
#34145=CARTESIAN_POINT('Ctrl Pts',(-1.73472347597681E-17,0.0853826423430476,
1.95213365433479));
#34146=CARTESIAN_POINT('Ctrl Pts',(-0.0370131733375648,0.733938965798307,
1.92376702457974));
#34147=CARTESIAN_POINT('Ctrl Pts',(-0.0740263466751305,1.36166300132472,
1.54711780353787));
#34148=CARTESIAN_POINT('Ctrl Pts',(-0.111039520012696,1.68787010406214,
0.990514925967878));
#34149=CARTESIAN_POINT('Ctrl Pts',(-0.148052693350262,2.01407720679956,
0.433912048397882));
#34150=CARTESIAN_POINT('Ctrl Pts',(-0.185065866687825,2.03876737674798,
-0.302644485700221));
#34151=CARTESIAN_POINT('Ctrl Pts',(-0.222079040025389,1.7485156439952,-0.880191139520007));
#34152=CARTESIAN_POINT('Ctrl Pts',(-0.259092213362953,1.45826391124243,
-1.45773779333978));
#34153=CARTESIAN_POINT('Ctrl Pts',(-0.296105386700518,0.853070275788427,
-1.87627456688123));
#34154=CARTESIAN_POINT('Ctrl Pts',(-0.333118560038082,0.210462245402071,
-1.94566760641157));
#34155=CARTESIAN_POINT('Ctrl Pts',(-0.370131733375646,-0.432145784984285,
-2.01506064594191));
#34156=CARTESIAN_POINT('Ctrl Pts',(-0.407144906713211,-1.11216821030301,
-1.73530995146117));
#34157=CARTESIAN_POINT('Ctrl Pts',(-0.444158080050774,-1.51940799416304,
-1.23368026463156));
#34158=CARTESIAN_POINT('Ctrl Pts',(-0.469482155992443,-1.79803774360075,
-0.890469803642078));
#34159=CARTESIAN_POINT('Ctrl Pts',(-0.494806231934111,-1.94897325447817,
-0.443393976333821));
#34160=CARTESIAN_POINT('Ctrl Pts',(-0.520130307875779,-1.95245178959834,
0.00157515171675247));
#34161=CARTESIAN_POINT('Origin',(0.329462113107775,0.,0.));
#34162=CARTESIAN_POINT('',(-0.0510757737844506,0.,0.));
#34163=CARTESIAN_POINT('',(0.7,-1.23357587978679,1.51069475268627E-16));
#34164=CARTESIAN_POINT('',(0.329462113107775,-0.625,-7.65404249467096E-17));
#34165=CARTESIAN_POINT('Origin',(0.7,0.,0.));
#34166=CARTESIAN_POINT('Origin',(2.3,-2.77555756156289E-16,-1.44337567297406));
#34167=CARTESIAN_POINT('',(2.08323056361362,-2.65143809681227E-16,-1.44337567297406));
#34168=CARTESIAN_POINT('',(2.08323056361362,-1.25,-0.721687836487032));
#34169=CARTESIAN_POINT('Ctrl Pts',(2.08323056361362,-5.89805981832114E-16,
-1.44337567297406));
#34170=CARTESIAN_POINT('Ctrl Pts',(2.11697695076186,-0.213078403143805,
-1.32035479956049));
#34171=CARTESIAN_POINT('Ctrl Pts',(2.13099428157845,-0.425048382906795,
-1.19797387468421));
#34172=CARTESIAN_POINT('Ctrl Pts',(2.13099428157845,-0.824951617093206,
-0.967089634776885));
#34173=CARTESIAN_POINT('Ctrl Pts',(2.11697695076186,-1.0369215968562,-0.844708709900604));
#34174=CARTESIAN_POINT('Ctrl Pts',(2.08323056361362,-1.25,-0.721687836487033));
#34175=CARTESIAN_POINT('',(0.7,-2.77555756156289E-16,-1.44337567297406));
#34176=CARTESIAN_POINT('',(2.3,-2.65143809681227E-16,-1.44337567297406));
#34177=CARTESIAN_POINT('',(0.7,-1.25,-0.721687836487032));
#34178=CARTESIAN_POINT('',(0.7,-1.25,-0.721687836487032));
#34179=CARTESIAN_POINT('',(2.3,-1.25,-0.721687836487032));
#34180=CARTESIAN_POINT('Origin',(2.3,-1.25,-0.721687836487032));
#34181=CARTESIAN_POINT('',(2.08323056361362,-1.25,0.721687836487032));
#34182=CARTESIAN_POINT('Ctrl Pts',(2.08323056361362,-1.25,-0.721687836487033));
#34183=CARTESIAN_POINT('Ctrl Pts',(2.11697695076186,-1.25,-0.475646089659891));
#34184=CARTESIAN_POINT('Ctrl Pts',(2.13099428157846,-1.25,-0.230884239907327));
#34185=CARTESIAN_POINT('Ctrl Pts',(2.13099428157846,-1.25,0.230884239907327));
#34186=CARTESIAN_POINT('Ctrl Pts',(2.11697695076186,-1.25,0.475646089659889));
#34187=CARTESIAN_POINT('Ctrl Pts',(2.08323056361362,-1.25,0.721687836487032));
#34188=CARTESIAN_POINT('',(0.7,-1.25,0.721687836487032));
#34189=CARTESIAN_POINT('',(0.7,-1.25,0.721687836487032));
#34190=CARTESIAN_POINT('',(2.3,-1.25,0.721687836487032));
#34191=CARTESIAN_POINT('Origin',(2.3,-1.25,0.721687836487032));
#34192=CARTESIAN_POINT('',(2.08323056361362,8.83812698937422E-17,1.44337567297406));
#34193=CARTESIAN_POINT('Ctrl Pts',(2.08323056361362,-1.25,0.721687836487032));
#34194=CARTESIAN_POINT('Ctrl Pts',(2.11697695076186,-1.0369215968562,0.844708709900604));
#34195=CARTESIAN_POINT('Ctrl Pts',(2.13099428157845,-0.824951617093207,
0.967089634776885));
#34196=CARTESIAN_POINT('Ctrl Pts',(2.13099428157846,-0.425048382906794,
1.19797387468421));
#34197=CARTESIAN_POINT('Ctrl Pts',(2.11697695076186,-0.213078403143805,
1.32035479956049));
#34198=CARTESIAN_POINT('Ctrl Pts',(2.08323056361362,3.46944695195361E-17,
1.44337567297406));
#34199=CARTESIAN_POINT('',(0.7,1.38777878078145E-16,1.44337567297406));
#34200=CARTESIAN_POINT('',(0.7,8.83812698937422E-17,1.44337567297406));
#34201=CARTESIAN_POINT('',(2.3,8.83812698937422E-17,1.44337567297406));
#34202=CARTESIAN_POINT('Origin',(2.3,0.,1.44337567297406));
#34203=CARTESIAN_POINT('',(2.08323056361362,1.25,0.721687836487032));
#34204=CARTESIAN_POINT('Ctrl Pts',(2.08323056361362,0.,1.44337567297406));
#34205=CARTESIAN_POINT('Ctrl Pts',(2.11697695076186,0.213078403143805,1.32035479956049));
#34206=CARTESIAN_POINT('Ctrl Pts',(2.13099428157846,0.425048382906794,1.19797387468421));
#34207=CARTESIAN_POINT('Ctrl Pts',(2.13099428157846,0.824951617093207,0.967089634776885));
#34208=CARTESIAN_POINT('Ctrl Pts',(2.11697695076186,1.0369215968562,0.844708709900604));
#34209=CARTESIAN_POINT('Ctrl Pts',(2.08323056361362,1.25,0.721687836487032));
#34210=CARTESIAN_POINT('',(0.7,1.25,0.721687836487032));
#34211=CARTESIAN_POINT('',(0.7,1.25,0.721687836487032));
#34212=CARTESIAN_POINT('',(2.3,1.25,0.721687836487032));
#34213=CARTESIAN_POINT('Origin',(2.3,1.25,-0.721687836487033));
#34214=CARTESIAN_POINT('',(2.08323056361362,1.25,-0.721687836487033));
#34215=CARTESIAN_POINT('Ctrl Pts',(2.08323056361362,1.25,-0.721687836487033));
#34216=CARTESIAN_POINT('Ctrl Pts',(2.11697695076186,1.03692159685619,-0.844708709900604));
#34217=CARTESIAN_POINT('Ctrl Pts',(2.13099428157846,0.824951617093206,-0.967089634776885));
#34218=CARTESIAN_POINT('Ctrl Pts',(2.13099428157846,0.425048382906794,-1.19797387468421));
#34219=CARTESIAN_POINT('Ctrl Pts',(2.11697695076186,0.213078403143804,-1.32035479956049));
#34220=CARTESIAN_POINT('Ctrl Pts',(2.08323056361362,-8.67361737988404E-16,
-1.44337567297407));
#34221=CARTESIAN_POINT('',(0.7,1.25,-0.721687836487033));
#34222=CARTESIAN_POINT('',(2.3,1.25,-0.721687836487033));
#34223=CARTESIAN_POINT('',(0.7,-2.65143809681227E-16,-1.44337567297406));
#34224=CARTESIAN_POINT('Origin',(2.3,1.25,0.721687836487032));
#34225=CARTESIAN_POINT('Ctrl Pts',(2.08323056361362,1.25,0.721687836487032));
#34226=CARTESIAN_POINT('Ctrl Pts',(2.11697695076186,1.25,0.47564608965989));
#34227=CARTESIAN_POINT('Ctrl Pts',(2.13099428157846,1.25,0.230884239907327));
#34228=CARTESIAN_POINT('Ctrl Pts',(2.13099428157846,1.25,-0.230884239907328));
#34229=CARTESIAN_POINT('Ctrl Pts',(2.11697695076186,1.25,-0.47564608965989));
#34230=CARTESIAN_POINT('Ctrl Pts',(2.08323056361362,1.25,-0.721687836487033));
#34231=CARTESIAN_POINT('',(0.7,1.25,-0.721687836487033));
#34232=CARTESIAN_POINT('Origin',(0.7,0.,0.));
#34233=CARTESIAN_POINT('Origin',(-20.,1.6,0.));
#34234=CARTESIAN_POINT('',(-20.,-1.6,-1.95943487863576E-16));
#34235=CARTESIAN_POINT('Origin',(-20.,0.,0.));
#34236=CARTESIAN_POINT('Origin',(-19.8,0.,0.));
#34237=CARTESIAN_POINT('',(-19.8,-1.8,-2.20436423846524E-16));
#34238=CARTESIAN_POINT('Origin',(-9.8,0.,0.));
#34239=CARTESIAN_POINT('Origin',(0.,0.,0.));
#34240=CARTESIAN_POINT('Origin',(0.,3.8,0.));
#34241=CARTESIAN_POINT('',(1.73472347597681E-17,-3.8,-4.65365783675994E-16));
#34242=CARTESIAN_POINT('Origin',(0.,0.,0.));
#34243=CARTESIAN_POINT('Origin',(0.125,0.,0.));
#34244=CARTESIAN_POINT('',(0.25,-3.8,-4.65365783675994E-16));
#34245=CARTESIAN_POINT('',(0.25,-4.65365783675994E-16,3.8));
#34246=CARTESIAN_POINT('Origin',(0.25,0.,0.));
#34247=CARTESIAN_POINT('',(0.125,-3.8,-4.65365783675994E-16));
#34248=CARTESIAN_POINT('Origin',(0.25,0.,0.));
#34249=CARTESIAN_POINT('Ctrl Pts',(0.25,0.,3.8));
#34250=CARTESIAN_POINT('Ctrl Pts',(0.25,-3.8,3.8));
#34251=CARTESIAN_POINT('Ctrl Pts',(0.25,-3.8,0.));
#34252=CARTESIAN_POINT('Ctrl Pts',(0.25,-3.8,-3.8));
#34253=CARTESIAN_POINT('Ctrl Pts',(0.25,0.,-3.8));
#34254=CARTESIAN_POINT('Ctrl Pts',(0.25,3.8,-3.8));
#34255=CARTESIAN_POINT('Ctrl Pts',(0.25,3.8,0.));
#34256=CARTESIAN_POINT('Ctrl Pts',(0.25,3.8,3.8));
#34257=CARTESIAN_POINT('Ctrl Pts',(0.25,0.,3.8));
#34258=CARTESIAN_POINT('Ctrl Pts',(1.75830245810501,0.,2.94383864898856));
#34259=CARTESIAN_POINT('Ctrl Pts',(1.75830245810501,-2.94383864898856,2.94383864898856));
#34260=CARTESIAN_POINT('Ctrl Pts',(1.75830245810501,-2.94383864898856,0.));
#34261=CARTESIAN_POINT('Ctrl Pts',(1.75830245810501,-2.94383864898856,-2.94383864898856));
#34262=CARTESIAN_POINT('Ctrl Pts',(1.75830245810501,0.,-2.94383864898856));
#34263=CARTESIAN_POINT('Ctrl Pts',(1.75830245810501,2.94383864898856,-2.94383864898856));
#34264=CARTESIAN_POINT('Ctrl Pts',(1.75830245810501,2.94383864898856,0.));
#34265=CARTESIAN_POINT('Ctrl Pts',(1.75830245810501,2.94383864898856,2.94383864898856));
#34266=CARTESIAN_POINT('Ctrl Pts',(1.75830245810501,0.,2.94383864898856));
#34267=CARTESIAN_POINT('Ctrl Pts',(2.13099428157846,0.,1.25));
#34268=CARTESIAN_POINT('Ctrl Pts',(2.13099428157846,-1.25,1.25));
#34269=CARTESIAN_POINT('Ctrl Pts',(2.13099428157846,-1.25,0.));
#34270=CARTESIAN_POINT('Ctrl Pts',(2.13099428157846,-1.25,-1.25));
#34271=CARTESIAN_POINT('Ctrl Pts',(2.13099428157846,0.,-1.25));
#34272=CARTESIAN_POINT('Ctrl Pts',(2.13099428157846,1.25,-1.25));
#34273=CARTESIAN_POINT('Ctrl Pts',(2.13099428157846,1.25,0.));
#34274=CARTESIAN_POINT('Ctrl Pts',(2.13099428157846,1.25,1.25));
#34275=CARTESIAN_POINT('Ctrl Pts',(2.13099428157846,0.,1.25));
#34276=CARTESIAN_POINT('Ctrl Pts',(2.08323056361362,0.,1.44337567297407));
#34277=CARTESIAN_POINT('Ctrl Pts',(1.65564775032955,0.,3.00210878759666));
#34278=CARTESIAN_POINT('Ctrl Pts',(0.25,0.,3.8));
#37162=UNCERTAINTY_MEASURE_WITH_UNIT(LENGTH_MEASURE(0.01),#37182,
'DISTANCE_ACCURACY_VALUE',
'Maximum model space distance between geometric entities at asserted c
onnectivities');
#37166=UNCERTAINTY_MEASURE_WITH_UNIT(LENGTH_MEASURE(0.01),#37182,
'DISTANCE_ACCURACY_VALUE',
'Maximum model space distance between geometric entities at asserted c
onnectivities');
#37177=(
GEOMETRIC_REPRESENTATION_CONTEXT(3)
GLOBAL_UNCERTAINTY_ASSIGNED_CONTEXT((#37162))
GLOBAL_UNIT_ASSIGNED_CONTEXT((#37182,#37184,#37185))
REPRESENTATION_CONTEXT('','3D')
);
#37181=(
GEOMETRIC_REPRESENTATION_CONTEXT(3)
GLOBAL_UNCERTAINTY_ASSIGNED_CONTEXT((#37166))
GLOBAL_UNIT_ASSIGNED_CONTEXT((#37182,#37184,#37185))
REPRESENTATION_CONTEXT('','3D')
);
#37182=(
LENGTH_UNIT()
NAMED_UNIT(*)
SI_UNIT(.MILLI.,.METRE.)
);
#37184=(
NAMED_UNIT(*)
PLANE_ANGLE_UNIT()
SI_UNIT($,.RADIAN.)
);
#37185=(
NAMED_UNIT(*)
SI_UNIT($,.STERADIAN.)
SOLID_ANGLE_UNIT()
);
#37196=SHAPE_DEFINITION_REPRESENTATION(#37210,#37247);
#37210=PRODUCT_DEFINITION_SHAPE('',$,#37262);
#37247=SHAPE_REPRESENTATION('',(#15916),#37177);
#37251=PRODUCT_DEFINITION_CONTEXT('part definition',#37295,'design');
#37262=PRODUCT_DEFINITION('2026-10-20-13-24-03-042','11_ISO_7380_M4x20',
#37276,#37251);
#37276=PRODUCT_DEFINITION_FORMATION('',$,#37307);
#37295=APPLICATION_CONTEXT(
'Core Data for Automotive Mechanical Design Process');
#37296=PRODUCT_CONTEXT('part definition',#37295,'mechanical');
#37307=PRODUCT('2026-10-20-13-24-03-042','11_ISO_7380_M4x20',$,(#37296));
#37374=COLOUR_RGB('Black',0.12,0.14,0.17);
#37375=FILL_AREA_STYLE_COLOUR('',#37374);
#37376=FILL_AREA_STYLE('',(#37375));
#37377=SURFACE_STYLE_FILL_AREA(#37376);
#37378=SURFACE_SIDE_STYLE('',(#37377));
#37379=SURFACE_STYLE_USAGE(.BOTH.,#37378);
#37380=PRESENTATION_STYLE_ASSIGNMENT((#37379));
ENDSEC;
END-ISO-10303-21;
